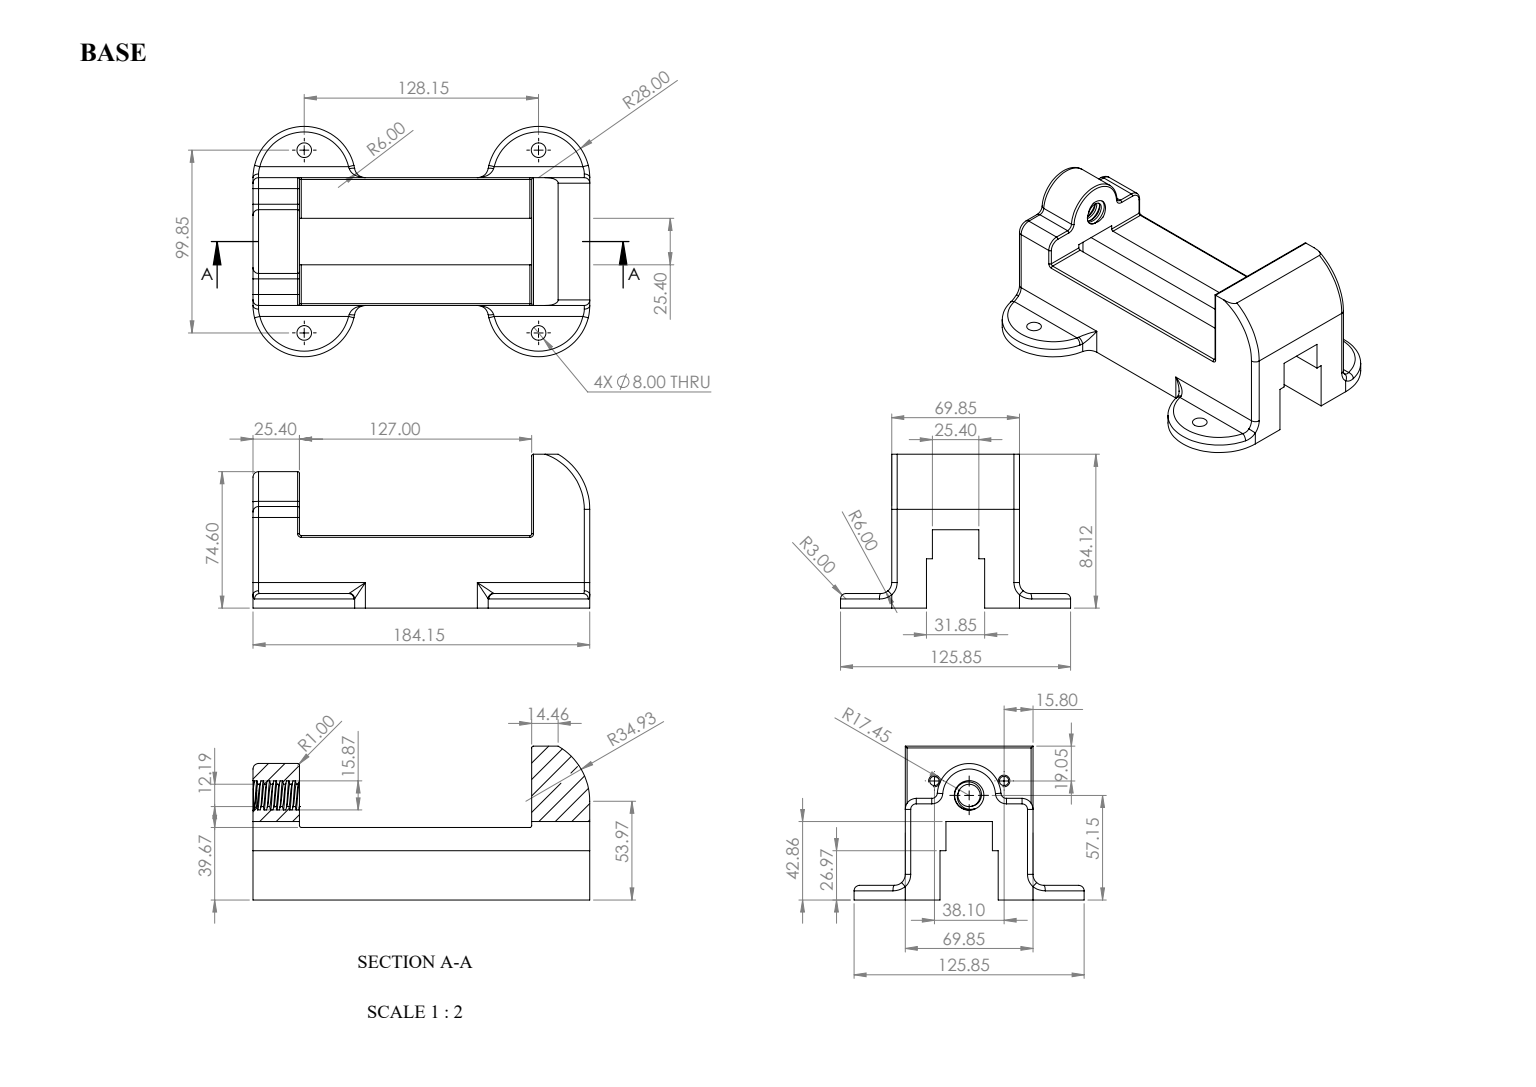
ISO-10303-21;
HEADER;
FILE_DESCRIPTION (('STEP AP214'),
    '1' );
FILE_NAME ('1.0 Base.step',
    '2026-10-06T08:51:13',
    ( '' ),
    ( '' ),
    'SwSTEP 2.0',
    'SolidWorks 2021',
    '' );
FILE_SCHEMA (( 'AUTOMOTIVE_DESIGN' ));
ENDSEC;

DATA;
#2=DIRECTION ( 'NONE',  ( 0.000000000000000000, 0.000000000000000000, -1.000000000000000000 ) ) ;
#4=CARTESIAN_POINT ( 'NONE',  ( 156.1499999999997783, -49.14999999999999147, -40.92499999999998295 ) ) ;
#20=DIRECTION ( 'NONE',  ( -1.000000000000000000, -0.000000000000000000, -0.000000000000000000 ) ) ;
#21=CYLINDRICAL_SURFACE ( 'NONE', #62371, 5.999999999999998224 ) ;
#28=AXIS2_PLACEMENT_3D ( 'NONE', #83260, #28167, #72429 ) ;
#56=ORIENTED_EDGE ( 'NONE', *, *, #91353, .F. ) ;
#80=CARTESIAN_POINT ( 'NONE',  ( 166.6274442290528555, 26.96999999999994202, -32.76433874914447131 ) ) ;
#88=CARTESIAN_POINT ( 'NONE',  ( 23.54623647476855552, -7.934999999999990727, 4.858786175617117713E-16 ) ) ;
#107=LINE ( 'NONE', #77033, #97406 ) ;
#112=MECHANICAL_DESIGN_GEOMETRIC_PRESENTATION_REPRESENTATION('',(#37206),#67225);
#141=( NAMED_UNIT ( * ) SI_UNIT ( $, .STERADIAN. ) SOLID_ANGLE_UNIT ( ) );
#143=ORIENTED_EDGE ( 'NONE', *, *, #47317, .T. ) ;
#169=AXIS2_PLACEMENT_3D ( 'NONE', #60485, #124990, #72084 ) ;
#182=CARTESIAN_POINT ( 'NONE',  ( 0.1600000000000011136, 3.289720434613005118, -7.220939306079887210 ) ) ;
#201=ORIENTED_EDGE ( 'NONE', *, *, #80508, .F. ) ;
#210=AXIS2_PLACEMENT_3D ( 'NONE', #18854, #51517, #105848 ) ;
#244=B_SPLINE_CURVE_WITH_KNOTS ( 'NONE', 3,
 ( #116047, #19597, #116769, #42097, #141380, #17451, #127667, #74728, #105869, #52917, #50814, #86307 ),
 .UNSPECIFIED., .F., .F.,
 ( 4, 2, 2, 2, 2, 4 ),
 ( 9.813815432834144085E-18, 0.001837441947543535809, 0.003674883895087062077, 0.004593604868858823694, 0.005512325842630587044, 0.007349767790174136298 ),
 .UNSPECIFIED. ) ;
#248=ADVANCED_FACE ( 'NONE', ( #84846 ), #37182, .F. ) ;
#274=CARTESIAN_POINT ( 'NONE',  ( -0.2245968585647807325, -2.126176841940958351, -7.934999999999989839 ) ) ;
#307=SURFACE_SIDE_STYLE ('',( #35140 ) ) ;
#315=ORIENTED_EDGE ( 'NONE', *, *, #1789, .F. ) ;
#365=MECHANICAL_DESIGN_GEOMETRIC_PRESENTATION_REPRESENTATION('',(#53591),#69867);
#369=EDGE_CURVE ( 'NONE', #137573, #138987, #81190, .T. ) ;
#372=CARTESIAN_POINT ( 'NONE',  ( 24.39999999999999858, -5.520864266206504263E-14, 0.000000000000000000 ) ) ;
#377=SURFACE_STYLE_USAGE ( .BOTH. , #24296 ) ;
#387=( NAMED_UNIT ( * ) SI_UNIT ( $, .STERADIAN. ) SOLID_ANGLE_UNIT ( ) );
#408=AXIS2_PLACEMENT_3D ( 'NONE', #118351, #30665, #74896 ) ;
#412=LINE ( 'NONE', #119338, #62884 ) ;
#443=MECHANICAL_DESIGN_GEOMETRIC_PRESENTATION_REPRESENTATION('',(#97739),#18987);
#457=CARTESIAN_POINT ( 'NONE',  ( 1.504139616203772789, -3.047499999999994547, 5.278424836066145431 ) ) ;
#484=CARTESIAN_POINT ( 'NONE',  ( 10.33290314143522082, -3.967499999999994476, 6.871911579029513106 ) ) ;
#486=DIRECTION ( 'NONE',  ( 0.000000000000000000, 0.000000000000000000, -1.000000000000000000 ) ) ;
#518=ORIENTED_EDGE ( 'NONE', *, *, #141850, .T. ) ;
#524=( NAMED_UNIT ( * ) SI_UNIT ( $, .STERADIAN. ) SOLID_ANGLE_UNIT ( ) );
#528=CARTESIAN_POINT ( 'NONE',  ( 18.22916666666666785, -6.094999999999989093, 1.633150327867691765 ) ) ;
#532=VECTOR ( 'NONE', #82631, 1000.000000000000000 ) ;
#538=COLOUR_RGB ( '', 0.09019608, 0.27058824, 0.51372549) ;
#587=ORIENTED_EDGE ( 'NONE', *, *, #53900, .F. ) ;
#590=CARTESIAN_POINT ( 'NONE',  ( 18.00456980810188767, 6.871911579029510442, -3.967499999999998916 ) ) ;
#592=CARTESIAN_POINT ( 'NONE',  ( 166.4267503027637929, 26.96999999999993847, 33.05223327726561422 ) ) ;
#634=CARTESIAN_POINT ( 'NONE',  ( 24.39999999999999858, -16.48000000000005016, 33.92499999999998295 ) ) ;
#651=B_SPLINE_CURVE_WITH_KNOTS ( 'NONE', 3,
 ( #139201, #42017, #96340, #72543, #117387, #140584, #118840, #17386, #41274, #9323, #39892, #85482, #18060, #129710, #30417, #19530, #31144, #107932, #8601, #52849, #97044, #141306, #86234, #119521, #53605, #103316, #91068, #114212, #48245, #79507, #101192, #14894, #25050, #57018 ),
 .UNSPECIFIED., .F., .F.,
 ( 4, 2, 2, 2, 2, 2, 2, 2, 2, 2, 2, 2, 2, 2, 2, 2, 4 ),
 ( 0.000000000000000000, 0.002428652292010244872, 0.003642978438015367741, 0.004857304584020490611, 0.006071630730025613480, 0.007285956876030735482, 0.008500283022035860087, 0.009714609168040984691, 0.01032177224104354613, 0.01092893531404610583, 0.01214326146005123043, 0.01335758760605635503, 0.01457191375206147964, 0.01578623989806660424, 0.01700056604407173058, 0.01821489219007685345, 0.01942921833608197632 ),
 .UNSPECIFIED. ) ;
#666=CARTESIAN_POINT ( 'NONE',  ( 16.10873647476855552, -5.808823158059033709, 5.808823158059035485 ) ) ;
#672=VERTEX_POINT ( 'NONE', #81409 ) ;
#679=FILL_AREA_STYLE ('',( #44971 ) ) ;
#692=FILL_AREA_STYLE_COLOUR ( '', #111503 ) ;
#702=CARTESIAN_POINT ( 'NONE',  ( 20.68706980810189222, -2.126176841940956130, 7.934999999999991616 ) ) ;
#720=CARTESIAN_POINT ( 'NONE',  ( 22.75000000000000355, -7.464222240803106570E-16, -6.094999999999989981 ) ) ;
#725=DIRECTION ( 'NONE',  ( -1.000000000000000000, 0.000000000000000000, -0.000000000000000000 ) ) ;
#768=EDGE_CURVE ( 'NONE', #109345, #74861, #53227, .T. ) ;
#785=EDGE_CURVE ( 'NONE', #137573, #33799, #105265, .T. ) ;
#826=CARTESIAN_POINT ( 'NONE',  ( 28.21290314143522338, 3.967499999999992699, -6.871911579029513994 ) ) ;
#875=EDGE_LOOP ( 'NONE', ( #85490, #63150, #94760, #112992 ) ) ;
#892=CARTESIAN_POINT ( 'NONE',  ( 1.342642840338568844, 0.4167709042101988004, 6.752357159661401376 ) ) ;
#910=ORIENTED_EDGE ( 'NONE', *, *, #110228, .T. ) ;
#939=ADVANCED_FACE ( 'NONE', ( #54479 ), #21, .F. ) ;
#946=AXIS2_PLACEMENT_3D ( 'NONE', #78392, #9523, #76993 ) ;
#975=ADVANCED_FACE ( 'NONE', ( #25374 ), #2165, .F. ) ;
#998=CARTESIAN_POINT ( 'NONE',  ( 31.98330628287044064, 6.094999999999991758, 1.633150327867687102 ) ) ;
#1009=EDGE_CURVE ( 'NONE', #4395, #106598, #120848, .T. ) ;
#1028=PRESENTATION_STYLE_ASSIGNMENT (( #46764 ) ) ;
#1035=DIRECTION ( 'NONE',  ( -0.000000000000000000, 1.000000000000000000, -0.000000000000000000 ) ) ;
#1043=( NAMED_UNIT ( * ) SI_UNIT ( $, .STERADIAN. ) SOLID_ANGLE_UNIT ( ) );
#1061=UNCERTAINTY_MEASURE_WITH_UNIT (LENGTH_MEASURE( 1.000000000000000082E-05 ), #107553, 'distance_accuracy_value', 'NONE');
#1082=AXIS2_PLACEMENT_3D ( 'NONE', #48681, #26916, #84193 ) ;
#1090=DIRECTION ( 'NONE',  ( -1.000000000000000000, -0.000000000000000000, 0.000000000000000000 ) ) ;
#1101=CIRCLE ( 'NONE', #47540, 2.552699999999990865 ) ;
#1141=CARTESIAN_POINT ( 'NONE',  ( 4.420806282870438864, 3.047499999999997655, 5.278424836066143655 ) ) ;
#1154=ORIENTED_EDGE ( 'NONE', *, *, #33420, .T. ) ;
#1163=CARTESIAN_POINT ( 'NONE',  ( 6.462472949537106715, -7.464222240803106570E-16, -6.094999999999989981 ) ) ;
#1194=CARTESIAN_POINT ( 'NONE',  ( 17.04123647476855652, 0.000000000000000000, 7.934999999999990727 ) ) ;
#1203=CARTESIAN_POINT ( 'NONE',  ( 156.1500000000000057, -49.14999999999999147, 49.92499999999997584 ) ) ;
#1221=( NAMED_UNIT ( * ) SI_UNIT ( $, .STERADIAN. ) SOLID_ANGLE_UNIT ( ) );
#1229=ORIENTED_EDGE ( 'NONE', *, *, #123542, .F. ) ;
#1240=CARTESIAN_POINT ( 'NONE',  ( 15.60416666666666430, -1.633150327867691987, -6.094999999999989093 ) ) ;
#1265=CARTESIAN_POINT ( 'NONE',  ( 156.1499999999997783, -52.14999999999999147, 34.92500000000004690 ) ) ;
#1268=CARTESIAN_POINT ( 'NONE',  ( 184.1499999999998067, -3.180000000000061444, 31.92499999999998295 ) ) ;
#1297=CARTESIAN_POINT ( 'NONE',  ( 24.85873647476855552, 5.808823158059031044, -5.808823158059037262 ) ) ;
#1322=CARTESIAN_POINT ( 'NONE',  ( 25.39999999999999858, 0.000000000000000000, 0.000000000000000000 ) ) ;
#1327=SURFACE_STYLE_FILL_AREA ( #56502 ) ;
#1332=ORIENTED_EDGE ( 'NONE', *, *, #26827, .F. ) ;
#1354=CARTESIAN_POINT ( 'NONE',  ( 13.75413961620377457, 3.047499999999993214, -5.278424836066146320 ) ) ;
#1363=CARTESIAN_POINT ( 'NONE',  ( 22.08790314143522338, 6.871911579029515771, 3.967499999999989146 ) ) ;
#1392=SURFACE_SIDE_STYLE ('',( #100744 ) ) ;
#1393=UNCERTAINTY_MEASURE_WITH_UNIT (LENGTH_MEASURE( 1.000000000000000082E-05 ), #82010, 'distance_accuracy_value', 'NONE');
#1407=CARTESIAN_POINT ( 'NONE',  ( 21.85373647476855297, -5.808823158059035485, -5.808823158059033709 ) ) ;
#1408=CARTESIAN_POINT ( 'NONE',  ( 0.7079031414352193741, -6.871911579029513106, -3.967499999999993587 ) ) ;
#1447=TOROIDAL_SURFACE ( 'NONE', #52377, 16.45000000000002061, 1.000000000000000000 ) ;
#1454=EDGE_CURVE ( 'NONE', #23170, #56532, #105103, .T. ) ;
#1462=DIRECTION ( 'NONE',  ( -0.000000000000000000, 1.000000000000000000, 0.000000000000000000 ) ) ;
#1477=STYLED_ITEM ( 'NONE', ( #106319 ), #33707 ) ;
#1480=CARTESIAN_POINT ( 'NONE',  ( 24.39999999999999858, -7.600000000000061817, 28.92499999999998650 ) ) ;
#1482=COLOUR_RGB ( '', 0.66274510, 0.83137255, 0.94901961) ;
#1484=ORIENTED_EDGE ( 'NONE', *, *, #38988, .F. ) ;
#1494=VECTOR ( 'NONE', #70882, 1000.000000000000000 ) ;
#1525=CARTESIAN_POINT ( 'NONE',  ( 23.98373647476855197, -5.808823158059035485, -5.808823158059033709 ) ) ;
#1556=CIRCLE ( 'NONE', #98752, 3.000000000000003109 ) ;
#1568=DIRECTION ( 'NONE',  ( 0.000000000000000000, 5.075120898959323014E-15, 1.000000000000000000 ) ) ;
#1597=DIRECTION ( 'NONE',  ( 0.000000000000000000, -0.000000000000000000, -1.000000000000000000 ) ) ;
#1618=CARTESIAN_POINT ( 'NONE',  ( 152.4000000000000057, 26.55578643762684266, -34.51078643762689069 ) ) ;
#1627=( LENGTH_UNIT ( ) NAMED_UNIT ( * ) SI_UNIT ( .MILLI., .METRE. ) );
#1645=DIRECTION ( 'NONE',  ( -0.000000000000000000, -1.000000000000000000, 0.000000000000000000 ) ) ;
#1687=EDGE_CURVE ( 'NONE', #77069, #96033, #119634, .T. ) ;
#1689=VECTOR ( 'NONE', #126123, 1000.000000000000227 ) ;
#1690=CARTESIAN_POINT ( 'NONE',  ( -1.245430191898114103, -6.871911579029512218, 3.967499999999996252 ) ) ;
#1722=SURFACE_SIDE_STYLE ('',( #57606 ) ) ;
#1732=CARTESIAN_POINT ( 'NONE',  ( 0.000000000000000000, -43.14999999999996305, -31.92499999999998295 ) ) ;
#1733=( LENGTH_UNIT ( ) NAMED_UNIT ( * ) SI_UNIT ( .MILLI., .METRE. ) );
#1789=EDGE_CURVE ( 'NONE', #98679, #119012, #89647, .T. ) ;
#1819=( BOUNDED_SURFACE ( )  B_SPLINE_SURFACE ( 3, 2, ( 
 ( #75238, #141164, #5640 ),
 ( #30275, #8477, #72404 ),
 ( #73785, #50607, #62935 ),
 ( #52728, #28860, #94792 ),
 ( #40465, #19397, #96921 ),
 ( #63650, #52038, #84666 ),
 ( #117253, #128868, #116573 ),
 ( #7786, #119399, #17258 ),
 ( #20093, #61519, #96217 ),
 ( #7051, #139052, #62213 ),
 ( #106368, #104975, #29544 ),
 ( #140459, #41150, #118705 ) ),
 .UNSPECIFIED., .F., .F., .F. ) 
 B_SPLINE_SURFACE_WITH_KNOTS ( ( 4, 2, 2, 2, 2, 4 ),
 ( 3, 3 ),
 ( 0.000000000000000000, 0.001647923167088021293, 0.002471884750632031939, 0.003295846334176042586, 0.004943769501264063879, 0.006591692668352085172 ),
 ( 0.000000000000000000, 1.000000000000000000 ),
 .UNSPECIFIED. ) 
 GEOMETRIC_REPRESENTATION_ITEM ( )  RATIONAL_B_SPLINE_SURFACE ( (
 ( 1.000000000000000000, 0.7071067811865475727, 1.000000000000000000),
 ( 1.000000000000000000, 0.7122033721489959834, 1.000000000000000000),
 ( 1.000000000000000000, 0.7158366153114920083, 1.000000000000000000),
 ( 1.000000000000000000, 0.7192720032935927543, 1.000000000000000000),
 ( 1.000000000000000000, 0.7200809050419634261, 1.000000000000000000),
 ( 1.000000000000000000, 0.7210491446662590231, 1.000000000000000000),
 ( 1.000000000000000000, 0.7212054070301950892, 1.000000000000000000),
 ( 1.000000000000000000, 0.7207522793911053105, 1.000000000000000000),
 ( 1.000000000000000000, 0.7192424821648278899, 1.000000000000000000),
 ( 1.000000000000000000, 0.7143802006615703748, 1.000000000000000000),
 ( 1.000000000000000000, 0.7109884861396060796, 1.000000000000000000),
 ( 1.000000000000000000, 0.7071067811865475727, 1.000000000000000000) ) ) 
 REPRESENTATION_ITEM ( '' )  SURFACE ( )  );
#1824=CARTESIAN_POINT ( 'NONE',  ( 3.108306282870440640, 1.633150327867692431, -6.094999999999989093 ) ) ;
#1849=CARTESIAN_POINT ( 'NONE',  ( 3.545806282870439308, 5.278424836066143655, -3.047499999999997655 ) ) ;
#1857=CARTESIAN_POINT ( 'NONE',  ( 156.1500000000000057, -49.14999999999999147, -49.92499999999968452 ) ) ;
#1881=CARTESIAN_POINT ( 'NONE',  ( 23.74956980810188867, 3.967499999999998916, 6.871911579029510442 ) ) ;
#1889=FILL_AREA_STYLE ('',( #136727 ) ) ;
#1893=SURFACE_SIDE_STYLE ('',( #93240 ) ) ;
#1898=DIRECTION ( 'NONE',  ( 0.000000000000000000, 0.000000000000000000, 1.000000000000000000 ) ) ;
#1909=CIRCLE ( 'NONE', #85349, 1.000000000000000888 ) ;
#1913=SURFACE_STYLE_USAGE ( .BOTH. , #78832 ) ;
#1930=CARTESIAN_POINT ( 'NONE',  ( 9.625000000000001776, 6.094999999999989981, -1.119633336120465690E-15 ) ) ;
#1931=CARTESIAN_POINT ( 'NONE',  ( 23.02040314143522082, 7.934999999999988951, -2.126176841940961904 ) ) ;
#1941=CYLINDRICAL_SURFACE ( 'NONE', #89996, 6.094999999999989093 ) ;
#1943=CARTESIAN_POINT ( 'NONE',  ( 126.2665610010987649, -48.52444309369079178, -36.09967824800681768 ) ) ;
#1986=CARTESIAN_POINT ( 'NONE',  ( 25.34729149122530245, 7.934999999999992504, 0.7443565279215664798 ) ) ;
#1988=MECHANICAL_DESIGN_GEOMETRIC_PRESENTATION_REPRESENTATION('',(#117493),#76141);
#1990=CARTESIAN_POINT ( 'NONE',  ( 122.6835989386367345, -49.14999999999999147, 40.92499999999998295 ) ) ;
#1992=CARTESIAN_POINT ( 'NONE',  ( 25.39999999999999858, -7.600000000000055600, -34.92499999999998295 ) ) ;
#2000=MECHANICAL_DESIGN_GEOMETRIC_PRESENTATION_REPRESENTATION('',(#32175),#101598);
#2002=EDGE_LOOP ( 'NONE', ( #24135, #30818, #116626, #50545 ) ) ;
#2035=EDGE_CURVE ( 'NONE', #89687, #67143, #85183, .T. ) ;
#2058=DIRECTION ( 'NONE',  ( 0.000000000000000000, 0.000000000000000000, 1.000000000000000000 ) ) ;
#2062=B_SPLINE_CURVE_WITH_KNOTS ( 'NONE', 3,
 ( #100924, #13179, #111820, #90042, #23356, #101638, #45166, #79231, #89342, #135028, #47329, #123436, #2291, #46612, #58919, #35722, #91500, #12482, #113220, #122669, #79942, #135712, #56764, #113949, #124113, #69039, #24790, #36396 ),
 .UNSPECIFIED., .F., .F.,
 ( 4, 2, 2, 2, 2, 2, 2, 2, 2, 2, 2, 2, 2, 4 ),
 ( 0.002830889048686786869, 0.003748869865235868355, 0.004666850681784949842, 0.005584831498334031329, 0.006502812314883112815, 0.008338773947981275789, 0.009256754764530356408, 0.01017473558107943703, 0.01109271639762851765, 0.01201069721417759653, 0.01292867803072667542, 0.01384665884727575430, 0.01568262048037391554, 0.01751858211347207331 ),
 .UNSPECIFIED. ) ;
#2063=CARTESIAN_POINT ( 'NONE',  ( 16.40040314143521982, -7.934999999999989839, 2.126176841940957907 ) ) ;
#2070=ORIENTED_EDGE ( 'NONE', *, *, #46056, .T. ) ;
#2076=SURFACE_STYLE_USAGE ( .BOTH. , #123925 ) ;
#2092=SURFACE_SIDE_STYLE ('',( #68167 ) ) ;
#2104=CARTESIAN_POINT ( 'NONE',  ( 23.16623647476855652, 7.934999999999990727, -1.457635852685135314E-15 ) ) ;
#2106=VECTOR ( 'NONE', #67234, 1000.000000000000000 ) ;
#2153=EDGE_CURVE ( 'NONE', #103874, #56532, #135388, .T. ) ;
#2158=CARTESIAN_POINT ( 'NONE',  ( 8.649972949537106715, -4.461849672132299105, 4.461849672132299993 ) ) ;
#2165=PLANE ( 'NONE',  #97069 ) ;
#2168=ORIENTED_EDGE ( 'NONE', *, *, #2569, .T. ) ;
#2219=ORIENTED_EDGE ( 'NONE', *, *, #107714, .F. ) ;
#2238=CARTESIAN_POINT ( 'NONE',  ( 24.27540314143521982, -2.126176841940958351, -7.934999999999989839 ) ) ;
#2245=ORIENTED_EDGE ( 'NONE', *, *, #101650, .F. ) ;
#2246=CARTESIAN_POINT ( 'NONE',  ( 25.39999999999999858, 1.194621026894847171, -17.40906030209848510 ) ) ;
#2278=LINE ( 'NONE', #124814, #21647 ) ;
#2291=CARTESIAN_POINT ( 'NONE',  ( 1.000065336733412913, -5.551087553957981591, -4.428894815882122415 ) ) ;
#2414=AXIS2_PLACEMENT_3D ( 'NONE', #81917, #4980, #106434 ) ;
#2417=CARTESIAN_POINT ( 'NONE',  ( 3.858736474768553304, 5.808823158059031044, -5.808823158059038150 ) ) ;
#2444=CARTESIAN_POINT ( 'NONE',  ( 21.19163961620376924, 6.094999999999988205, -1.633150327867694651 ) ) ;
#2449=EDGE_CURVE ( 'NONE', #21837, #31597, #130626, .T. ) ;
#2455=CARTESIAN_POINT ( 'NONE',  ( 0.2704031414352194296, -7.934999999999989839, 2.126176841940957907 ) ) ;
#2461=UNCERTAINTY_MEASURE_WITH_UNIT (LENGTH_MEASURE( 1.000000000000000082E-05 ), #59794, 'distance_accuracy_value', 'NONE');
#2466=CARTESIAN_POINT ( 'NONE',  ( 156.1500000000000057, -49.14999999999999147, 45.92499999999998295 ) ) ;
#2473=CARTESIAN_POINT ( 'NONE',  ( 26.40000000000000568, -17.48000000000005016, 12.69999999999954454 ) ) ;
#2482=UNCERTAINTY_MEASURE_WITH_UNIT (LENGTH_MEASURE( 1.000000000000000082E-05 ), #112838, 'distance_accuracy_value', 'NONE');
#2484=DIRECTION ( 'NONE',  ( -1.000000000000000000, -0.000000000000000000, 0.000000000000000000 ) ) ;
#2547=CIRCLE ( 'NONE', #139195, 25.00000000000002842 ) ;
#2558=( GEOMETRIC_REPRESENTATION_CONTEXT ( 3 ) GLOBAL_UNCERTAINTY_ASSIGNED_CONTEXT ( ( #139093 ) ) GLOBAL_UNIT_ASSIGNED_CONTEXT ( ( #79225, #54587, #141 ) ) REPRESENTATION_CONTEXT ( 'NONE', 'WORKASPACE' ) );
#2569=EDGE_CURVE ( 'NONE', #119600, #105140, #15754, .T. ) ;
#2572=ORIENTED_EDGE ( 'NONE', *, *, #62327, .T. ) ;
#2594=CARTESIAN_POINT ( 'NONE',  ( 8.212472949537106715, 0.000000000000000000, 6.094999999999989981 ) ) ;
#2606=SURFACE_STYLE_FILL_AREA ( #78778 ) ;
#2621=( LENGTH_UNIT ( ) NAMED_UNIT ( * ) SI_UNIT ( .MILLI., .METRE. ) );
#2630=CARTESIAN_POINT ( 'NONE',  ( 19.66623647476855297, 7.934999999999990727, -1.457635852685135314E-15 ) ) ;
#2660=ORIENTED_EDGE ( 'NONE', *, *, #41190, .F. ) ;
#2675=CARTESIAN_POINT ( 'NONE',  ( 17.50000000000000000, 0.000000000000000000, 6.094999999999989981 ) ) ;
#2677=CARTESIAN_POINT ( 'NONE',  ( 24.18706980810188867, -2.126176841940956130, 7.934999999999990727 ) ) ;
#2691=CARTESIAN_POINT ( 'NONE',  ( 124.0768256643040388, -45.23984008851422089, -35.04755940937664604 ) ) ;
#2693=DIRECTION ( 'NONE',  ( 0.000000000000000000, 0.000000000000000000, 1.000000000000000000 ) ) ;
#2739=FACE_OUTER_BOUND ( 'NONE', #96191, .T. ) ;
#2740=CARTESIAN_POINT ( 'NONE',  ( 25.15040314143521627, 7.934999999999988951, -2.126176841940961904 ) ) ;
#2753=EDGE_CURVE ( 'NONE', #89590, #131877, #7216, .T. ) ;
#2777=VERTEX_POINT ( 'NONE', #129650 ) ;
#2786=STYLED_ITEM ( 'NONE', ( #120887 ), #31273 ) ;
#2799=CARTESIAN_POINT ( 'NONE',  ( 14.33747294953710494, 6.094999999999989981, -1.119633336120465690E-15 ) ) ;
#2808=CARTESIAN_POINT ( 'NONE',  ( 30.69206980810189123, -7.934999999999991616, -2.126176841940955242 ) ) ;
#2831=STYLED_ITEM ( 'NONE', ( #89354 ), #66228 ) ;
#2835=CARTESIAN_POINT ( 'NONE',  ( 60.76962477605442814, -44.19516442797058886, -34.92499999999998295 ) ) ;
#2842=UNCERTAINTY_MEASURE_WITH_UNIT (LENGTH_MEASURE( 1.000000000000000082E-05 ), #105526, 'distance_accuracy_value', 'NONE');
#2852=CARTESIAN_POINT ( 'NONE',  ( 23.31206980810188512, 7.934999999999993392, 2.126176841940951689 ) ) ;
#2862=B_SPLINE_CURVE_WITH_KNOTS ( 'NONE', 3,
 ( #57172, #101347, #46299, #18589, #127377, #96156, #83174, #116512, #70891, #16449, #94730, #40400, #51980, #60754 ),
 .UNSPECIFIED., .F., .F.,
 ( 4, 2, 2, 2, 2, 2, 4 ),
 ( 0.000000000000000000, 0.001506850370412668103, 0.002260275555619002154, 0.003013700740825336205, 0.003767125926031670256, 0.004520551111238004308, 0.006027401481650672410 ),
 .UNSPECIFIED. ) ;
#2879=CARTESIAN_POINT ( 'NONE',  ( 26.40000000000000568, -16.48000000000005016, 34.92499999999998295 ) ) ;
#2909=CARTESIAN_POINT ( 'NONE',  ( 1.233736474768552860, 5.808823158059035485, 5.808823158059032821 ) ) ;
#2933=ADVANCED_FACE ( 'NONE', ( #92376 ), #37674, .T. ) ;
#2978=CARTESIAN_POINT ( 'NONE',  ( 29.52540314143522338, 2.126176841940962348, 7.934999999999989839 ) ) ;
#2979=CARTESIAN_POINT ( 'NONE',  ( 0.6504031414352192675, 7.934999999999989839, -2.126176841940961904 ) ) ;
#3010=EDGE_CURVE ( 'NONE', #9331, #58595, #93214, .T. ) ;
#3016=SURFACE_STYLE_USAGE ( .BOTH. , #22088 ) ;
#3105=FILL_AREA_STYLE ('',( #68415 ) ) ;
#3140=VERTEX_POINT ( 'NONE', #21270 ) ;
#3149=CARTESIAN_POINT ( 'NONE',  ( -1.099596858564781066, -7.934999999999989839, 2.126176841940957907 ) ) ;
#3172=CARTESIAN_POINT ( 'NONE',  ( 20.60830628287044419, 1.633150327867706864, -6.094999999999981100 ) ) ;
#3181=AXIS2_PLACEMENT_3D ( 'NONE', #78101, #67216, #1898 ) ;
#3185=DIRECTION ( 'NONE',  ( -0.000000000000000000, 0.000000000000000000, 1.000000000000000000 ) ) ;
#3192=FILL_AREA_STYLE ('',( #26399 ) ) ;
#3206=CARTESIAN_POINT ( 'NONE',  ( 24.39999999999999858, -16.48000000000005016, 34.92499999999998295 ) ) ;
#3278=( LENGTH_UNIT ( ) NAMED_UNIT ( * ) SI_UNIT ( .MILLI., .METRE. ) );
#3307=CARTESIAN_POINT ( 'NONE',  ( 2.087472949537105826, -6.094999999999989981, 3.732111120401553285E-16 ) ) ;
#3324=ORIENTED_EDGE ( 'NONE', *, *, #105654, .T. ) ;
#3328=( NAMED_UNIT ( * ) SI_UNIT ( $, .STERADIAN. ) SOLID_ANGLE_UNIT ( ) );
#3338=CARTESIAN_POINT ( 'NONE',  ( 26.66623647476855652, 7.934999999999990727, -1.457635852685135314E-15 ) ) ;
#3354=MECHANICAL_DESIGN_GEOMETRIC_PRESENTATION_REPRESENTATION('',(#65920),#119170);
#3369=SURFACE_STYLE_FILL_AREA ( #102724 ) ;
#3383=CARTESIAN_POINT ( 'NONE',  ( 19.25000000000000355, -7.464222240803106570E-16, -6.094999999999989981 ) ) ;
#3440=CARTESIAN_POINT ( 'NONE',  ( 55.56056557994604361, -49.14999999999999147, -39.86617647058817937 ) ) ;
#3447=( GEOMETRIC_REPRESENTATION_CONTEXT ( 3 ) GLOBAL_UNCERTAINTY_ASSIGNED_CONTEXT ( ( #46051 ) ) GLOBAL_UNIT_ASSIGNED_CONTEXT ( ( #123452, #36410, #103772 ) ) REPRESENTATION_CONTEXT ( 'NONE', 'WORKASPACE' ) );
#3501=CARTESIAN_POINT ( 'NONE',  ( 25.44206980810188412, 7.934999999999993392, 2.126176841940951689 ) ) ;
#3503=LINE ( 'NONE', #47794, #110755 ) ;
#3529=( NAMED_UNIT ( * ) PLANE_ANGLE_UNIT ( ) SI_UNIT ( $, .RADIAN. ) );
#3537=( BOUNDED_CURVE ( )  B_SPLINE_CURVE ( 2, ( #138028, #61913, #72821, #114807, #71352, #93800, #25682, #126417, #59081, #4581, #92352, #27829, #94498 ),
 .UNSPECIFIED., .F., .T. ) 
 B_SPLINE_CURVE_WITH_KNOTS ( ( 3, 2, 2, 2, 2, 2, 3 ),
 ( 0.3000000000000000444, 0.3083333333333334036, 0.3166666666666667074, 0.3250000000000000666, 0.3333333333333333703, 0.3416666666666667296, 0.3500000000000000333 ),
 .UNSPECIFIED. ) 
 CURVE ( )  GEOMETRIC_REPRESENTATION_ITEM ( )  RATIONAL_B_SPLINE_CURVE ( ( 0.9999999999999997780, 0.9659258262890685343, 1.000000000000000000, 0.9659258262890683122, 1.000000000000000000, 0.9659258262890683122, 1.000000000000000000, 0.9659258262890683122, 1.000000000000000000, 0.9659258262890683122, 1.000000000000000000, 0.9659258262890680902, 1.000000000000000222 ) ) 
 REPRESENTATION_ITEM ( '' )  );
#3545=CARTESIAN_POINT ( 'NONE',  ( 30.45790314143522437, 6.871911579029515771, 3.967499999999989146 ) ) ;
#3558=CARTESIAN_POINT ( 'NONE',  ( 25.39999999999999858, -57.15000000000009095, 34.92499999999998295 ) ) ;
#3574=CARTESIAN_POINT ( 'NONE',  ( 25.39999999999999858, -43.14999999999999147, 34.92499999999998295 ) ) ;
#3600=CARTESIAN_POINT ( 'NONE',  ( 1.962903141435219601, -3.967499999999994476, 6.871911579029513106 ) ) ;
#3601=EDGE_CURVE ( 'NONE', #112055, #60580, #89222, .T. ) ;
#3620=DIRECTION ( 'NONE',  ( 0.000000000000000000, 0.000000000000000000, -1.000000000000000000 ) ) ;
#3633=ORIENTED_EDGE ( 'NONE', *, *, #118658, .T. ) ;
#3660=CARTESIAN_POINT ( 'NONE',  ( 32.73373647476854842, 5.808823158059036373, 5.808823158059032821 ) ) ;
#3662=CARTESIAN_POINT ( 'NONE',  ( 0.9420698081018860082, 7.934999999999993392, 2.126176841940951689 ) ) ;
#3666=CIRCLE ( 'NONE', #29167, 5.999999999999998224 ) ;
#3677=CARTESIAN_POINT ( 'NONE',  ( 56.90810577924025893, -46.18886352141517904, -34.92499999999998295 ) ) ;
#3695=DIRECTION ( 'NONE',  ( 0.000000000000000000, -1.000000000000000000, 0.000000000000000000 ) ) ;
#3702=CARTESIAN_POINT ( 'NONE',  ( 184.1500000000000057, -30.18000000000009564, -15.92500000000064375 ) ) ;
#3707=ORIENTED_EDGE ( 'NONE', *, *, #112697, .F. ) ;
#3713=EDGE_LOOP ( 'NONE', ( #114435, #13870, #8632, #138126 ) ) ;
#3729=CARTESIAN_POINT ( 'NONE',  ( 0.7902862351827044662, 7.048400157404861588, 1.962111654240061398 ) ) ;
#3737=( LENGTH_UNIT ( ) NAMED_UNIT ( * ) SI_UNIT ( .MILLI., .METRE. ) );
#3746=DIRECTION ( 'NONE',  ( -1.000000000000000000, -0.000000000000000000, 0.000000000000000000 ) ) ;
#3788=SURFACE_STYLE_FILL_AREA ( #37178 ) ;
#3809=( GEOMETRIC_REPRESENTATION_CONTEXT ( 3 ) GLOBAL_UNCERTAINTY_ASSIGNED_CONTEXT ( ( #30502 ) ) GLOBAL_UNIT_ASSIGNED_CONTEXT ( ( #103757, #72641, #27642 ) ) REPRESENTATION_CONTEXT ( 'NONE', 'WORKASPACE' ) );
#3824=CARTESIAN_POINT ( 'NONE',  ( 5.608736474768551972, -5.808823158059033709, 5.808823158059035485 ) ) ;
#3832=CARTESIAN_POINT ( 'NONE',  ( 24.50000000000000000, 0.000000000000000000, 6.094999999999989981 ) ) ;
#3843=EDGE_CURVE ( 'NONE', #4395, #28418, #104084, .T. ) ;
#3863=CARTESIAN_POINT ( 'NONE',  ( 1.145403141435219485, -2.126176841940958351, -7.934999999999989839 ) ) ;
#3891=UNCERTAINTY_MEASURE_WITH_UNIT (LENGTH_MEASURE( 1.000000000000000082E-05 ), #7913, 'distance_accuracy_value', 'NONE');
#3906=COLOUR_RGB ( '', 0.40784314, 0.44705882, 0.49803922) ;
#3966=( NAMED_UNIT ( * ) SI_UNIT ( $, .STERADIAN. ) SOLID_ANGLE_UNIT ( ) );
#3982=CARTESIAN_POINT ( 'NONE',  ( 10.25413961620377457, 3.047499999999993214, -5.278424836066146320 ) ) ;
#4005=SURFACE_STYLE_USAGE ( .BOTH. , #25818 ) ;
#4011=ORIENTED_EDGE ( 'NONE', *, *, #127323, .T. ) ;
#4014=CARTESIAN_POINT ( 'NONE',  ( 18.35373647476854941, -5.808823158059035485, -5.808823158059033709 ) ) ;
#4047=( NAMED_UNIT ( * ) SI_UNIT ( $, .STERADIAN. ) SOLID_ANGLE_UNIT ( ) );
#4061=CARTESIAN_POINT ( 'NONE',  ( 20.12500000000000000, 6.094999999999989981, -1.119633336120465690E-15 ) ) ;
#4111=FILL_AREA_STYLE_COLOUR ( '', #91954 ) ;
#4147=ADVANCED_FACE ( 'NONE', ( #92736 ), #28926, .F. ) ;
#4156=SURFACE_STYLE_USAGE ( .BOTH. , #17921 ) ;
#4174=CARTESIAN_POINT ( 'NONE',  ( 23.98373647476855197, -5.808823158059035485, -5.808823158059033709 ) ) ;
#4197=FILL_AREA_STYLE_COLOUR ( '', #16370 ) ;
#4217=CARTESIAN_POINT ( 'NONE',  ( 24.39999999999999858, -2.599999999999900169, -1.445354724476153568E-14 ) ) ;
#4218=CARTESIAN_POINT ( 'NONE',  ( 30.31206980810188512, 7.934999999999993392, 2.126176841940951689 ) ) ;
#4220=CARTESIAN_POINT ( 'NONE',  ( 15.21247294953710671, 0.000000000000000000, 6.094999999999989981 ) ) ;
#4228=FILL_AREA_STYLE_COLOUR ( '', #87383 ) ;
#4232=MECHANICAL_DESIGN_GEOMETRIC_PRESENTATION_REPRESENTATION('',(#34422),#124659);
#4237=COLOUR_RGB ( '', 0.09019608, 0.27058824, 0.51372549) ;
#4257=CONICAL_SURFACE ( 'NONE', #36705, 2.552699999999928693, 1.029744258676634772 ) ;
#4267=FACE_OUTER_BOUND ( 'NONE', #27129, .T. ) ;
#4277=CARTESIAN_POINT ( 'NONE',  ( 3.275403141435219823, -2.126176841940958351, -7.934999999999988951 ) ) ;
#4278=( LENGTH_UNIT ( ) NAMED_UNIT ( * ) SI_UNIT ( .MILLI., .METRE. ) );
#4285=CIRCLE ( 'NONE', #64597, 2.552699999999990865 ) ;
#4299=( NAMED_UNIT ( * ) PLANE_ANGLE_UNIT ( ) SI_UNIT ( $, .RADIAN. ) );
#4324=COLOUR_RGB ( '', 0.66274510, 0.83137255, 0.94901961) ;
#4327=FILL_AREA_STYLE_COLOUR ( '', #10280 ) ;
#4344=CARTESIAN_POINT ( 'NONE',  ( -0.9537635252314473622, -7.934999999999990727, 4.858786175617117713E-16 ) ) ;
#4355=( NAMED_UNIT ( * ) SI_UNIT ( $, .STERADIAN. ) SOLID_ANGLE_UNIT ( ) );
#4357=LINE ( 'NONE', #1992, #28863 ) ;
#4360=SURFACE_SIDE_STYLE ('',( #15271 ) ) ;
#4386=CARTESIAN_POINT ( 'NONE',  ( 2.187499999999999556, 4.461849672132297329, -4.461849672132302658 ) ) ;
#4395=VERTEX_POINT ( 'NONE', #65617 ) ;
#4466=STYLED_ITEM ( 'NONE', ( #105922 ), #96794 ) ;
#4495=MECHANICAL_DESIGN_GEOMETRIC_PRESENTATION_REPRESENTATION('',(#18400),#32319);
#4503=B_SPLINE_CURVE_WITH_KNOTS ( 'NONE', 3,
 ( #32332, #76565, #120745, #21451 ),
 .UNSPECIFIED., .F., .F.,
 ( 4, 4 ),
 ( 0.000000000000000000, 0.001824211539880358363 ),
 .UNSPECIFIED. ) ;
#4516=CARTESIAN_POINT ( 'NONE',  ( 5.171236474768553748, 0.000000000000000000, 7.934999999999990727 ) ) ;
#4554=CARTESIAN_POINT ( 'NONE',  ( 3.187069808101886448, -2.126176841940956130, 7.934999999999991616 ) ) ;
#4571=( NAMED_UNIT ( * ) PLANE_ANGLE_UNIT ( ) SI_UNIT ( $, .RADIAN. ) );
#4581=CARTESIAN_POINT ( 'NONE',  ( 11.81250000000000178, -4.461849672132299993, -4.461849672132299105 ) ) ;
#4610=CARTESIAN_POINT ( 'NONE',  ( 25.39999999999999858, -2.599999999999908606, 1.319531433729349815E-14 ) ) ;
#4627=CYLINDRICAL_SURFACE ( 'NONE', #126308, 5.999999999999998224 ) ;
#4645=VECTOR ( 'NONE', #19677, 1000.000000000000000 ) ;
#4662=SHAPE_DEFINITION_REPRESENTATION ( #15602, #40289 ) ;
#4696=CARTESIAN_POINT ( 'NONE',  ( 13.17080628287043886, -3.047499999999997211, -5.278424836066143655 ) ) ;
#4718=( NAMED_UNIT ( * ) PLANE_ANGLE_UNIT ( ) SI_UNIT ( $, .RADIAN. ) );
#4727=CARTESIAN_POINT ( 'NONE',  ( 20.83290314143522082, -3.967499999999994476, 6.871911579029513106 ) ) ;
#4764=CARTESIAN_POINT ( 'NONE',  ( 156.1499999999997783, -52.14999999999999147, -34.92499999999975557 ) ) ;
#4779=CARTESIAN_POINT ( 'NONE',  ( 27.85416666666666785, 1.633150327867695095, 6.094999999999988205 ) ) ;
#4804=CARTESIAN_POINT ( 'NONE',  ( 1.534715839894093881, -2.368487323979017400, 6.120741323661095024 ) ) ;
#4807=ORIENTED_EDGE ( 'NONE', *, *, #20774, .T. ) ;
#4814=( NAMED_UNIT ( * ) PLANE_ANGLE_UNIT ( ) SI_UNIT ( $, .RADIAN. ) );
#4831=ORIENTED_EDGE ( 'NONE', *, *, #48583, .F. ) ;
#4849=SURFACE_STYLE_USAGE ( .BOTH. , #94045 ) ;
#4852=SURFACE_STYLE_USAGE ( .BOTH. , #70905 ) ;
#4872=ORIENTED_EDGE ( 'NONE', *, *, #107178, .F. ) ;
#4906=FILL_AREA_STYLE_COLOUR ( '', #83444 ) ;
#4910=CARTESIAN_POINT ( 'NONE',  ( 29.96290314143522338, -3.967499999999994476, 6.871911579029513106 ) ) ;
#4916=MECHANICAL_DESIGN_GEOMETRIC_PRESENTATION_REPRESENTATION('',(#51342),#48971);
#4954=CARTESIAN_POINT ( 'NONE',  ( 33.08290314143522437, 3.967499999999992699, -6.871911579029513994 ) ) ;
#4955=CARTESIAN_POINT ( 'NONE',  ( 6.249569808101886004, 3.967499999999998916, 6.871911579029510442 ) ) ;
#4963=ORIENTED_EDGE ( 'NONE', *, *, #113865, .T. ) ;
#4971=VECTOR ( 'NONE', #7647, 1000.000000000000000 ) ;
#4980=DIRECTION ( 'NONE',  ( 0.2400000000000085398, 0.000000000000000000, -0.9707728879609256456 ) ) ;
#4990=ORIENTED_EDGE ( 'NONE', *, *, #122325, .F. ) ;
#5009=FILL_AREA_STYLE ('',( #59471 ) ) ;
#5019=CARTESIAN_POINT ( 'NONE',  ( 8.962903141435219823, -3.967499999999994476, 6.871911579029513106 ) ) ;
#5021=CARTESIAN_POINT ( 'NONE',  ( 21.29166666666666785, -3.047499999999994547, 5.278424836066145431 ) ) ;
#5030=EDGE_CURVE ( 'NONE', #53957, #2777, #59742, .T. ) ;
#5048=CARTESIAN_POINT ( 'NONE',  ( 131.5423521607622490, -49.05583548141700589, 39.86617647058822911 ) ) ;
#5063=ORIENTED_EDGE ( 'NONE', *, *, #50610, .F. ) ;
#5080=DIRECTION ( 'NONE',  ( 0.000000000000000000, -0.000000000000000000, 1.000000000000000000 ) ) ;
#5091=CARTESIAN_POINT ( 'NONE',  ( 3.421236474768552860, -9.717572351234235426E-16, -7.934999999999990727 ) ) ;
#5095=( NAMED_UNIT ( * ) SI_UNIT ( $, .STERADIAN. ) SOLID_ANGLE_UNIT ( ) );
#5102=FILL_AREA_STYLE_COLOUR ( '', #42754 ) ;
#5104=CARTESIAN_POINT ( 'NONE',  ( 183.9400257540259531, -51.66308182546809746, -38.35990878063539355 ) ) ;
#5117=ADVANCED_FACE ( 'NONE', ( #15237 ), #37016, .F. ) ;
#5124=STYLED_ITEM ( 'NONE', ( #127792 ), #25975 ) ;
#5136=CYLINDRICAL_SURFACE ( 'NONE', #12259, 6.094999999999989093 ) ;
#5141=CARTESIAN_POINT ( 'NONE',  ( 24.39999999999999858, -2.600000000000013856, 20.40202195861968448 ) ) ;
#5143=EDGE_CURVE ( 'NONE', #60071, #48370, #140733, .T. ) ;
#5165=AXIS2_PLACEMENT_3D ( 'NONE', #117507, #137881, #71926 ) ;
#5175=ORIENTED_EDGE ( 'NONE', *, *, #110228, .F. ) ;
#5238=DIRECTION ( 'NONE',  ( 1.000000000000000000, 0.000000000000000000, 0.000000000000000000 ) ) ;
#5240=VERTEX_POINT ( 'NONE', #42762 ) ;
#5275=CARTESIAN_POINT ( 'NONE',  ( 5.900403141435219823, -7.934999999999989839, 2.126176841940957907 ) ) ;
#5277=VERTEX_POINT ( 'NONE', #44929 ) ;
#5289=DIRECTION ( 'NONE',  ( 0.000000000000000000, -1.000000000000000000, 0.000000000000000000 ) ) ;
#5303=CARTESIAN_POINT ( 'NONE',  ( 22.06663961620377279, 1.633150327867675555, 6.094999999999998863 ) ) ;
#5306=FILL_AREA_STYLE_COLOUR ( '', #110919 ) ;
#5315=CARTESIAN_POINT ( 'NONE',  ( 2.749569808101886004, 3.967499999999998916, 6.871911579029510442 ) ) ;
#5340=SURFACE_STYLE_FILL_AREA ( #69961 ) ;
#5341=VERTEX_POINT ( 'NONE', #22374 ) ;
#5373=CARTESIAN_POINT ( 'NONE',  ( 27.99999999999999645, -49.14999999999999147, -53.92499999999967741 ) ) ;
#5443=CARTESIAN_POINT ( 'NONE',  ( 16.67080628287043709, -3.047499999999997211, -5.278424836066143655 ) ) ;
#5449=COLOUR_RGB ( '', 0.66274510, 0.83137255, 0.94901961) ;
#5493=CARTESIAN_POINT ( 'NONE',  ( 3.730677800976860414, -49.14999999999999147, -40.92499999999998295 ) ) ;
#5525=CARTESIAN_POINT ( 'NONE',  ( 27.70833333333333570, 3.047499999999997655, 5.278424836066143655 ) ) ;
#5542=( NAMED_UNIT ( * ) SI_UNIT ( $, .STERADIAN. ) SOLID_ANGLE_UNIT ( ) );
#5551=CARTESIAN_POINT ( 'NONE',  ( 13.12500000000000178, 6.094999999999989981, -1.119633336120465690E-15 ) ) ;
#5553=CARTESIAN_POINT ( 'NONE',  ( 1.586284118322663916, -3.036554765565917968, 5.760036735694805010 ) ) ;
#5594=PRESENTATION_STYLE_ASSIGNMENT (( #4852 ) ) ;
#5627=CARTESIAN_POINT ( 'NONE',  ( 131.8806778009765708, -49.14999999999999147, 40.92499999999998295 ) ) ;
#5640=CARTESIAN_POINT ( 'NONE',  ( 0.8183591370940052068, -52.14999999999999147, 41.64499999999997470 ) ) ;
#5645=CARTESIAN_POINT ( 'NONE',  ( 32.00456980810188412, 6.871911579029510442, -3.967499999999998916 ) ) ;
#5682=EDGE_CURVE ( 'NONE', #106911, #141737, #13233, .T. ) ;
#5691=CARTESIAN_POINT ( 'NONE',  ( 33.37456980810188156, 6.871911579029510442, -3.967499999999998916 ) ) ;
#5692=CARTESIAN_POINT ( 'NONE',  ( 11.20790314143521904, -6.871911579029513106, -3.967499999999993587 ) ) ;
#5727=CARTESIAN_POINT ( 'NONE',  ( 7.729166666666666075, -6.094999999999989093, 1.633150327867691542 ) ) ;
#5732=STYLED_ITEM ( 'NONE', ( #133041 ), #88424 ) ;
#5738=CARTESIAN_POINT ( 'NONE',  ( 2.999999999999999112, -1.600000000000012301, -20.40202195861969514 ) ) ;
#5747=CARTESIAN_POINT ( 'NONE',  ( 10.85873647476855197, 5.808823158059031044, -5.808823158059037262 ) ) ;
#5764=CARTESIAN_POINT ( 'NONE',  ( 5.979166666666666075, 6.094999999999988205, -1.633150327867694651 ) ) ;
#5814=PRESENTATION_STYLE_ASSIGNMENT (( #105159 ) ) ;
#5823=DIRECTION ( 'NONE',  ( 0.000000000000000000, -1.000000000000000000, -1.286409696682840916E-16 ) ) ;
#5840=ORIENTED_EDGE ( 'NONE', *, *, #768, .F. ) ;
#5842=FILL_AREA_STYLE_COLOUR ( '', #108488 ) ;
#5845=UNCERTAINTY_MEASURE_WITH_UNIT (LENGTH_MEASURE( 1.000000000000000082E-05 ), #115592, 'distance_accuracy_value', 'NONE');
#5849=VECTOR ( 'NONE', #77625, 1000.000000000000000 ) ;
#5860=CARTESIAN_POINT ( 'NONE',  ( 28.00000000000002487, -49.14999999999999147, 34.92500000000003268 ) ) ;
#5870=CARTESIAN_POINT ( 'NONE',  ( 152.4000000000000057, -17.48000000000005016, 33.92499999999998295 ) ) ;
#5887=FILL_AREA_STYLE_COLOUR ( '', #129432 ) ;
#5931=CARTESIAN_POINT ( 'NONE',  ( 26.40000000000000568, -17.48000000000005016, 33.92499999999998295 ) ) ;
#5974=( LENGTH_UNIT ( ) NAMED_UNIT ( * ) SI_UNIT ( .MILLI., .METRE. ) );
#5975=CARTESIAN_POINT ( 'NONE',  ( 12.46290314143521982, -3.967499999999994476, 6.871911579029513106 ) ) ;
#6008=CARTESIAN_POINT ( 'NONE',  ( 1.291236474768552966, -9.717572351234235426E-16, -7.934999999999990727 ) ) ;
#6022=CARTESIAN_POINT ( 'NONE',  ( 25.39999999999999858, -7.600000000000061817, 28.92499999999998650 ) ) ;
#6024=SURFACE_STYLE_USAGE ( .BOTH. , #103918 ) ;
#6042=VECTOR ( 'NONE', #92227, 1000.000000000000000 ) ;
#6062=ORIENTED_EDGE ( 'NONE', *, *, #94553, .T. ) ;
#6073=CARTESIAN_POINT ( 'NONE',  ( 156.1499999999997783, -52.14999999999999147, -34.92499999999975557 ) ) ;
#6085=ORIENTED_EDGE ( 'NONE', *, *, #43646, .F. ) ;
#6088=CARTESIAN_POINT ( 'NONE',  ( 184.1500000000000057, -14.29000000000013593, 12.69999999999954632 ) ) ;
#6110=( GEOMETRIC_REPRESENTATION_CONTEXT ( 3 ) GLOBAL_UNCERTAINTY_ASSIGNED_CONTEXT ( ( #66366 ) ) GLOBAL_UNIT_ASSIGNED_CONTEXT ( ( #12189, #133982, #23043 ) ) REPRESENTATION_CONTEXT ( 'NONE', 'WORKASPACE' ) );
#6142=CARTESIAN_POINT ( 'NONE',  ( 13.46247294953710494, -7.464222240803106570E-16, -6.094999999999989981 ) ) ;
#6157=ADVANCED_FACE ( 'NONE', ( #112419 ), #45761, .F. ) ;
#6160=ORIENTED_EDGE ( 'NONE', *, *, #23573, .T. ) ;
#6174=CARTESIAN_POINT ( 'NONE',  ( 30.16623647476855652, 7.934999999999990727, -1.457635852685135314E-15 ) ) ;
#6188=CARTESIAN_POINT ( 'NONE',  ( 0.7113915074146799356, -49.19295221407797669, -41.21232802154111141 ) ) ;
#6214=SURFACE_SIDE_STYLE ('',( #49800 ) ) ;
#6219=CARTESIAN_POINT ( 'NONE',  ( 20.85416666666666075, 1.633150327867695095, 6.094999999999988205 ) ) ;
#6238=FILL_AREA_STYLE ('',( #84582 ) ) ;
#6246=VECTOR ( 'NONE', #87593, 1000.000000000000000 ) ;
#6255=CARTESIAN_POINT ( 'NONE',  ( 184.1500000000000057, -30.18000000000009564, 15.92499999999935945 ) ) ;
#6288=ORIENTED_EDGE ( 'NONE', *, *, #47317, .F. ) ;
#6291=CARTESIAN_POINT ( 'NONE',  ( 11.85830628287044242, -1.633150327867709528, 6.094999999999979323 ) ) ;
#6324=AXIS2_PLACEMENT_3D ( 'NONE', #1990, #36804, #81050 ) ;
#6328=( NAMED_UNIT ( * ) PLANE_ANGLE_UNIT ( ) SI_UNIT ( $, .RADIAN. ) );
#6331=COLOUR_RGB ( '', 0.08235294, 0.09019608, 0.10196078) ;
#6333=CARTESIAN_POINT ( 'NONE',  ( 6.249569808101886004, 3.967499999999998916, 6.871911579029510442 ) ) ;
#6374=CARTESIAN_POINT ( 'NONE',  ( 30.16623647476855652, 7.934999999999990727, -1.457635852685135314E-15 ) ) ;
#6375=CARTESIAN_POINT ( 'NONE',  ( 10.04123647476855297, 0.000000000000000000, 7.934999999999990727 ) ) ;
#6398=( NAMED_UNIT ( * ) SI_UNIT ( $, .STERADIAN. ) SOLID_ANGLE_UNIT ( ) );
#6409=CARTESIAN_POINT ( 'NONE',  ( 123.3803752239310541, -44.19516442798762768, 34.92499999999998295 ) ) ;
#6427=AXIS2_PLACEMENT_3D ( 'NONE', #98853, #42374, #53209 ) ;
#6432=CARTESIAN_POINT ( 'NONE',  ( 5.317069808101886785, -2.126176841940956130, 7.934999999999990727 ) ) ;
#6501=DIRECTION ( 'NONE',  ( 0.000000000000000000, 0.000000000000000000, 1.000000000000000000 ) ) ;
#6503=CARTESIAN_POINT ( 'NONE',  ( 11.15040314143521982, 7.934999999999989839, -2.126176841940961904 ) ) ;
#6513=ORIENTED_EDGE ( 'NONE', *, *, #369, .T. ) ;
#6514=CARTESIAN_POINT ( 'NONE',  ( 151.4000000000000057, -16.48000000000005016, -33.92499999999998295 ) ) ;
#6516=CARTESIAN_POINT ( 'NONE',  ( 183.7681020908649714, -51.95642703809001972, -39.54367611436801866 ) ) ;
#6545=CARTESIAN_POINT ( 'NONE',  ( 2.770833333333333925, 6.094999999999991758, 1.633150327867686880 ) ) ;
#6560=ORIENTED_EDGE ( 'NONE', *, *, #1789, .T. ) ;
#6561=VERTEX_POINT ( 'NONE', #17429 ) ;
#6582=DIRECTION ( 'NONE',  ( -1.000000000000000000, 0.000000000000000000, 0.000000000000000000 ) ) ;
#6585=FILL_AREA_STYLE_COLOUR ( '', #97108 ) ;
#6595=LINE ( 'NONE', #116113, #25603 ) ;
#6656=AXIS2_PLACEMENT_3D ( 'NONE', #90986, #135214, #11217 ) ;
#6682=CARTESIAN_POINT ( 'NONE',  ( 11.44206980810188767, 7.934999999999993392, 2.126176841940951689 ) ) ;
#6713=CARTESIAN_POINT ( 'NONE',  ( 10.62456980810188689, -6.871911579029512218, 3.967499999999996252 ) ) ;
#6731=( GEOMETRIC_REPRESENTATION_CONTEXT ( 3 ) GLOBAL_UNCERTAINTY_ASSIGNED_CONTEXT ( ( #30139 ) ) GLOBAL_UNIT_ASSIGNED_CONTEXT ( ( #121693, #97057, #63788 ) ) REPRESENTATION_CONTEXT ( 'NONE', 'WORKASPACE' ) );
#6758=PRESENTATION_STYLE_ASSIGNMENT (( #63376 ) ) ;
#6799=VECTOR ( 'NONE', #44639, 1000.000000000000000 ) ;
#6833=DIRECTION ( 'NONE',  ( 0.000000000000000000, 0.000000000000000000, 1.000000000000000000 ) ) ;
#6834=CARTESIAN_POINT ( 'NONE',  ( 2.999999999999999112, -5.520864266206504263E-14, 0.000000000000000000 ) ) ;
#6855=CARTESIAN_POINT ( 'NONE',  ( 16.23330628287043353, -6.094999999999989981, -1.633150327867689100 ) ) ;
#6930=CARTESIAN_POINT ( 'NONE',  ( 34.41666666666667140, 5.278424836066147208, 3.047499999999990550 ) ) ;
#6952=CARTESIAN_POINT ( 'NONE',  ( 1.573529187797693574, -2.874494765961987497, 5.856845438429902018 ) ) ;
#6955=FACE_OUTER_BOUND ( 'NONE', #44327, .T. ) ;
#6994=EDGE_CURVE ( 'NONE', #62992, #119600, #73181, .T. ) ;
#6998=CARTESIAN_POINT ( 'NONE',  ( 25.39999999999999858, -5.520864266206504263E-14, 0.000000000000000000 ) ) ;
#7015=EDGE_CURVE ( 'NONE', #87517, #66916, #85704, .T. ) ;
#7031=FACE_BOUND ( 'NONE', #121992, .T. ) ;
#7044=CIRCLE ( 'NONE', #88135, 5.999999999999998224 ) ;
#7051=CARTESIAN_POINT ( 'NONE',  ( 3.010427959778288365, -48.08977582060914813, 37.49964900842618931 ) ) ;
#7054=CARTESIAN_POINT ( 'NONE',  ( 5.228736474768552078, 5.808823158059031044, -5.808823158059038150 ) ) ;
#7063=VECTOR ( 'NONE', #56221, 1000.000000000000000 ) ;
#7090=UNCERTAINTY_MEASURE_WITH_UNIT (LENGTH_MEASURE( 1.000000000000000082E-05 ), #95434, 'distance_accuracy_value', 'NONE');
#7102=CARTESIAN_POINT ( 'NONE',  ( 7.583333333333333925, -5.278424836066144543, 3.047499999999995879 ) ) ;
#7104=CARTESIAN_POINT ( 'NONE',  ( 10.18706980810188512, -2.126176841940956130, 7.934999999999990727 ) ) ;
#7115=AXIS2_PLACEMENT_3D ( 'NONE', #136900, #70271, #2058 ) ;
#7130=CARTESIAN_POINT ( 'NONE',  ( 55.64345981607718272, -48.97294124528174564, 39.12804664298385404 ) ) ;
#7139=COLOUR_RGB ( '', 0.09019608, 0.27058824, 0.51372549) ;
#7164=CARTESIAN_POINT ( 'NONE',  ( 4.587903141435219823, 6.871911579029515771, 3.967499999999989146 ) ) ;
#7182=CARTESIAN_POINT ( 'NONE',  ( 25.39999999999999858, -1.600000000000060929, 28.92500000000001847 ) ) ;
#7185=SURFACE_SIDE_STYLE ('',( #73217 ) ) ;
#7216=CIRCLE ( 'NONE', #134568, 6.094999999999989093 ) ;
#7227=SURFACE_STYLE_USAGE ( .BOTH. , #142773 ) ;
#7237=CARTESIAN_POINT ( 'NONE',  ( 5.171236474768553748, 0.000000000000000000, 7.934999999999990727 ) ) ;
#7266=VECTOR ( 'NONE', #105847, 1000.000000000000000 ) ;
#7322=( NAMED_UNIT ( * ) PLANE_ANGLE_UNIT ( ) SI_UNIT ( $, .RADIAN. ) );
#7335=( NAMED_UNIT ( * ) PLANE_ANGLE_UNIT ( ) SI_UNIT ( $, .RADIAN. ) );
#7380=CARTESIAN_POINT ( 'NONE',  ( 3.730677800976790248, -49.14999999999999147, 40.92499999999998295 ) ) ;
#7383=CARTESIAN_POINT ( 'NONE',  ( 181.1500000000000057, -43.14999999999999147, -40.92499999999998295 ) ) ;
#7398=ADVANCED_FACE ( 'NONE', ( #73054 ), #116524, .T. ) ;
#7420=CARTESIAN_POINT ( 'NONE',  ( 16.10873647476855552, -5.808823158059033709, 5.808823158059035485 ) ) ;
#7452=CARTESIAN_POINT ( 'NONE',  ( 16.02040314143522082, 7.934999999999989839, -2.126176841940961904 ) ) ;
#7471=VECTOR ( 'NONE', #37741, 1000.000000000000000 ) ;
#7524=SURFACE_SIDE_STYLE ('',( #131478 ) ) ;
#7536=CARTESIAN_POINT ( 'NONE',  ( 153.4000000000000057, -1.600000000000094458, 33.92499999999998295 ) ) ;
#7541=SURFACE_STYLE_FILL_AREA ( #18402 ) ;
#7593=CARTESIAN_POINT ( 'NONE',  ( 15.64997294953710671, -4.461849672132299105, 4.461849672132299993 ) ) ;
#7618=ORIENTED_EDGE ( 'NONE', *, *, #116171, .F. ) ;
#7623=CARTESIAN_POINT ( 'NONE',  ( 30.02040314143521726, 7.934999999999989839, -2.126176841940961904 ) ) ;
#7639=CARTESIAN_POINT ( 'NONE',  ( 0.5414528859221161561, -52.10163751122234999, -40.43817685073778279 ) ) ;
#7647=DIRECTION ( 'NONE',  ( 0.000000000000000000, -2.556434596176436521E-15, -1.000000000000000000 ) ) ;
#7651=COLOUR_RGB ( '', 0.08235294, 0.09019608, 0.10196078) ;
#7662=CARTESIAN_POINT ( 'NONE',  ( 0.000000000000000000, 0.000000000000000000, 0.000000000000000000 ) ) ;
#7666=FILL_AREA_STYLE_COLOUR ( '', #90669 ) ;
#7676=CARTESIAN_POINT ( 'NONE',  ( 28.43750000000000355, -4.461849672132299105, 4.461849672132299993 ) ) ;
#7686=CIRCLE ( 'NONE', #125798, 5.999999999999998224 ) ;
#7736=CARTESIAN_POINT ( 'NONE',  ( 180.4193221990230143, -49.14999999999999147, 40.92499999999998295 ) ) ;
#7748=CARTESIAN_POINT ( 'NONE',  ( 122.6835989386367345, -57.15000000000009095, 34.92499999999998295 ) ) ;
#7776=( LENGTH_UNIT ( ) NAMED_UNIT ( * ) SI_UNIT ( .MILLI., .METRE. ) );
#7786=CARTESIAN_POINT ( 'NONE',  ( 3.100164867288737636, -48.63026969829241608, 38.45492102172730142 ) ) ;
#7790=CARTESIAN_POINT ( 'NONE',  ( 8.291236474768552966, -9.717572351234235426E-16, -7.934999999999990727 ) ) ;
#7802=( NAMED_UNIT ( * ) SI_UNIT ( $, .STERADIAN. ) SOLID_ANGLE_UNIT ( ) );
#7820=CARTESIAN_POINT ( 'NONE',  ( 56.00844637038503748, -48.60795469097138977, -38.18754904900253422 ) ) ;
#7840=CARTESIAN_POINT ( 'NONE',  ( 3.500000000000000444, 0.000000000000000000, 6.094999999999989981 ) ) ;
#7841=CARTESIAN_POINT ( 'NONE',  ( 7.416236474768552078, -7.934999999999990727, 4.858786175617117713E-16 ) ) ;
#7867=CARTESIAN_POINT ( 'NONE',  ( 59.09089496824217491, -46.71325913968129129, 35.40428284070832632 ) ) ;
#7893=CARTESIAN_POINT ( 'NONE',  ( 7.942069808101886785, 7.934999999999992504, 2.126176841940951689 ) ) ;
#7908=AXIS2_PLACEMENT_3D ( 'NONE', #106381, #84678, #141939 ) ;
#7913=( LENGTH_UNIT ( ) NAMED_UNIT ( * ) SI_UNIT ( .MILLI., .METRE. ) );
#7935=FACE_BOUND ( 'NONE', #73889, .T. ) ;
#7954=DIRECTION ( 'NONE',  ( 0.000000000000000000, 0.000000000000000000, -1.000000000000000000 ) ) ;
#7962=CARTESIAN_POINT ( 'NONE',  ( 8.087903141435219823, 6.871911579029515771, 3.967499999999989146 ) ) ;
#7969=EDGE_CURVE ( 'NONE', #79775, #53362, #53220, .T. ) ;
#7983=EDGE_LOOP ( 'NONE', ( #79443, #2245, #129630, #14927 ) ) ;
#8089=SURFACE_STYLE_FILL_AREA ( #64646 ) ;
#8106=COLOUR_RGB ( '', 0.09019608, 0.27058824, 0.51372549) ;
#8127=CARTESIAN_POINT ( 'NONE',  ( 22.37956980810188767, 3.967499999999998916, 6.871911579029510442 ) ) ;
#8154=CARTESIAN_POINT ( 'NONE',  ( 4.812500000000000000, -4.461849672132299993, -4.461849672132299105 ) ) ;
#8161=CARTESIAN_POINT ( 'NONE',  ( 13.39540314143521904, 2.126176841940962348, 7.934999999999989839 ) ) ;
#8174=FILL_AREA_STYLE_COLOUR ( '', #125320 ) ;
#8195=CARTESIAN_POINT ( 'NONE',  ( 10.50000000000000000, 0.000000000000000000, 6.094999999999989981 ) ) ;
#8277=( NAMED_UNIT ( * ) PLANE_ANGLE_UNIT ( ) SI_UNIT ( $, .RADIAN. ) );
#8280=DIRECTION ( 'NONE',  ( 0.000000000000000000, -1.000000000000000000, 0.000000000000000000 ) ) ;
#8288=EDGE_CURVE ( 'NONE', #26834, #50573, #47239, .T. ) ;
#8290=CARTESIAN_POINT ( 'NONE',  ( 26.44163961620376924, -6.094999999999989093, 1.633150327867691765 ) ) ;
#8322=CARTESIAN_POINT ( 'NONE',  ( 32.35373647476855297, -5.808823158059035485, -5.808823158059033709 ) ) ;
#8328=VERTEX_POINT ( 'NONE', #42032 ) ;
#8366=CARTESIAN_POINT ( 'NONE',  ( 30.62500000000000355, 6.094999999999989981, -1.119633336120465690E-15 ) ) ;
#8371=ORIENTED_EDGE ( 'NONE', *, *, #127305, .T. ) ;
#8385=CARTESIAN_POINT ( 'NONE',  ( 131.8806778009766276, -49.14999999999999147, -40.92499999999998295 ) ) ;
#8408=STYLED_ITEM ( 'NONE', ( #109723 ), #111305 ) ;
#8412=SURFACE_STYLE_FILL_AREA ( #41087 ) ;
#8456=LINE ( 'NONE', #83218, #99586 ) ;
#8477=CARTESIAN_POINT ( 'NONE',  ( 0.7113915074196556221, -49.19295221407733010, 41.21232802153977559 ) ) ;
#8480=CARTESIAN_POINT ( 'NONE',  ( 2.457903141435219485, 6.871911579029515771, 3.967499999999989146 ) ) ;
#8504=CARTESIAN_POINT ( 'NONE',  ( 55.47138350052864553, -49.14501756083437556, -40.36361034346621324 ) ) ;
#8518=( LENGTH_UNIT ( ) NAMED_UNIT ( * ) SI_UNIT ( .MILLI., .METRE. ) );
#8522=CARTESIAN_POINT ( 'NONE',  ( 3.791666666666666963, -3.047499999999994547, 5.278424836066145431 ) ) ;
#8523=CARTESIAN_POINT ( 'NONE',  ( 13.10373647476855297, 5.808823158059035485, 5.808823158059032821 ) ) ;
#8535=CARTESIAN_POINT ( 'NONE',  ( 131.3130295073068226, -48.90295371244954481, -39.18578444878617262 ) ) ;
#8540=EDGE_CURVE ( 'NONE', #93434, #68280, #91259, .T. ) ;
#8542=CARTESIAN_POINT ( 'NONE',  ( -1.807144792967049773E-15, -50.24077216217763464, 35.40405119785170029 ) ) ;
#8549=CARTESIAN_POINT ( 'NONE',  ( 54.24578869845078088, -47.96374157527325366, 37.32649486623284929 ) ) ;
#8556=CARTESIAN_POINT ( 'NONE',  ( 130.9531400719712906, -48.66302742222553235, 38.53170190052306054 ) ) ;
#8575=CARTESIAN_POINT ( 'NONE',  ( 15.96290314143521805, -3.967499999999994476, 6.871911579029513106 ) ) ;
#8597=VERTEX_POINT ( 'NONE', #13643 ) ;
#8598=SURFACE_STYLE_FILL_AREA ( #31141 ) ;
#8601=CARTESIAN_POINT ( 'NONE',  ( 25.39999999999999858, 4.836323036001208386, -6.294117125145909597 ) ) ;
#8609=CIRCLE ( 'NONE', #27177, 1.000000000000000888 ) ;
#8616=DIRECTION ( 'NONE',  ( -1.000000000000000000, -0.000000000000000000, -0.000000000000000000 ) ) ;
#8632=ORIENTED_EDGE ( 'NONE', *, *, #28784, .F. ) ;
#8644=EDGE_LOOP ( 'NONE', ( #129095, #201 ) ) ;
#8650=CARTESIAN_POINT ( 'NONE',  ( 12.46290314143521982, -3.967499999999994476, 6.871911579029513106 ) ) ;
#8658=CARTESIAN_POINT ( 'NONE',  ( 131.7507865773015681, -49.14999999999999147, -40.57473644908944266 ) ) ;
#8663=CARTESIAN_POINT ( 'NONE',  ( 61.46640106136302961, -43.14999999999999147, -34.92499999999998295 ) ) ;
#8687=DIRECTION ( 'NONE',  ( 0.000000000000000000, 0.000000000000000000, -1.000000000000000000 ) ) ;
#8723=VERTEX_POINT ( 'NONE', #29518 ) ;
#8749=AXIS2_PLACEMENT_3D ( 'NONE', #81267, #103672, #127610 ) ;
#8773=ADVANCED_FACE ( 'NONE', ( #19375 ), #74469, .T. ) ;
#8790=DIRECTION ( 'NONE',  ( 0.9843059135694992579, 0.000000000000000000, -0.1764705882353009014 ) ) ;
#8812=EDGE_CURVE ( 'NONE', #80652, #31146, #92844, .T. ) ;
#8813=CARTESIAN_POINT ( 'NONE',  ( 15.52540314143522160, 2.126176841940962348, 7.934999999999989839 ) ) ;
#8836=CARTESIAN_POINT ( 'NONE',  ( 3.500000000000000444, 0.000000000000000000, 6.094999999999989981 ) ) ;
#8842=CARTESIAN_POINT ( 'NONE',  ( 14.56206980810188334, -7.934999999999991616, -2.126176841940955242 ) ) ;
#8873=SURFACE_STYLE_FILL_AREA ( #50495 ) ;
#8906=CARTESIAN_POINT ( 'NONE',  ( 9.524972949537108491, -4.461849672132299993, -4.461849672132299105 ) ) ;
#8911=FILL_AREA_STYLE_COLOUR ( '', #67955 ) ;
#8925=CARTESIAN_POINT ( 'NONE',  ( 0.000000000000000000, 0.000000000000000000, 0.000000000000000000 ) ) ;
#8983=CARTESIAN_POINT ( 'NONE',  ( 28.33747294953710849, 6.094999999999989981, -1.119633336120465690E-15 ) ) ;
#9009=STYLED_ITEM ( 'NONE', ( #13081 ), #113213 ) ;
#9058=CIRCLE ( 'NONE', #90127, 3.999999999999996447 ) ;
#9059=COLOUR_RGB ( '', 0.72549020, 0.75294118, 0.79215686) ;
#9072=CARTESIAN_POINT ( 'NONE',  ( 30.33333333333333570, 5.278424836066143655, -3.047499999999997655 ) ) ;
#9132=CARTESIAN_POINT ( 'NONE',  ( 183.7681020908654261, -51.95642703808907470, 39.54367611436589414 ) ) ;
#9162=CARTESIAN_POINT ( 'NONE',  ( -1.558360383796227655, -6.094999999999989093, 1.633150327867691765 ) ) ;
#9190=CARTESIAN_POINT ( 'NONE',  ( 11.93706980810188689, 2.126176841940952134, -7.934999999999993392 ) ) ;
#9209=EDGE_LOOP ( 'NONE', ( #126002, #32613, #23661, #139940 ) ) ;
#9224=( GEOMETRIC_REPRESENTATION_CONTEXT ( 3 ) GLOBAL_UNCERTAINTY_ASSIGNED_CONTEXT ( ( #24410 ) ) GLOBAL_UNIT_ASSIGNED_CONTEXT ( ( #34609, #112183, #133921 ) ) REPRESENTATION_CONTEXT ( 'NONE', 'WORKASPACE' ) );
#9229=DIRECTION ( 'NONE',  ( 0.000000000000000000, 0.000000000000000000, 1.000000000000000000 ) ) ;
#9235=CARTESIAN_POINT ( 'NONE',  ( 1.020833333333333481, -6.094999999999989981, -1.633150327867689100 ) ) ;
#9236=CARTESIAN_POINT ( 'NONE',  ( 18.06206980810188867, -7.934999999999990727, -2.126176841940955242 ) ) ;
#9238=PLANE ( 'NONE',  #30410 ) ;
#9243=VECTOR ( 'NONE', #115543, 1000.000000000000000 ) ;
#9275=CARTESIAN_POINT ( 'NONE',  ( 128.5894344200537489, -52.00875322212550600, 39.86617647058824332 ) ) ;
#9293=CARTESIAN_POINT ( 'NONE',  ( 13.92123647476855197, -9.717572351234235426E-16, -7.934999999999990727 ) ) ;
#9295=CARTESIAN_POINT ( 'NONE',  ( 160.4290834833332440, 26.96999999999994913, 34.92499999999999716 ) ) ;
#9308=ORIENTED_EDGE ( 'NONE', *, *, #86393, .T. ) ;
#9323=CARTESIAN_POINT ( 'NONE',  ( 25.40000000000001279, 0.9275341018601235277, -7.891049174277950051 ) ) ;
#9331=VERTEX_POINT ( 'NONE', #115644 ) ;
#9371=VECTOR ( 'NONE', #19258, 1000.000000000000000 ) ;
#9372=CARTESIAN_POINT ( 'NONE',  ( 9.108736474768550195, -5.808823158059033709, 5.808823158059035485 ) ) ;
#9410=CARTESIAN_POINT ( 'NONE',  ( 0.1600000000000004752, -2.314171071560278126, -7.597438125929392605 ) ) ;
#9413=FILL_AREA_STYLE_COLOUR ( '', #32192 ) ;
#9438=STYLED_ITEM ( 'NONE', ( #80911 ), #115316 ) ;
#9449=CARTESIAN_POINT ( 'NONE',  ( 23.91666666666666785, 5.278424836066147208, 3.047499999999990550 ) ) ;
#9497=CARTESIAN_POINT ( 'NONE',  ( 156.1500000000000057, -49.14999999999999147, -53.92499999999968452 ) ) ;
#9512=FACE_OUTER_BOUND ( 'NONE', #24619, .T. ) ;
#9523=DIRECTION ( 'NONE',  ( -0.000000000000000000, 1.000000000000000000, -0.000000000000000000 ) ) ;
#9556=CARTESIAN_POINT ( 'NONE',  ( 17.71290314143521982, 3.967499999999992699, -6.871911579029513994 ) ) ;
#9588=VERTEX_POINT ( 'NONE', #80770 ) ;
#9666=CARTESIAN_POINT ( 'NONE',  ( 9.233306282870437087, -6.094999999999989981, -1.633150327867689322 ) ) ;
#9693=ORIENTED_EDGE ( 'NONE', *, *, #71235, .T. ) ;
#9719=DIRECTION ( 'NONE',  ( 0.000000000000000000, -1.734723475976807686E-15, 1.000000000000000000 ) ) ;
#9740=CARTESIAN_POINT ( 'NONE',  ( 26.73330628287044064, -6.094999999999989981, -1.633150327867689100 ) ) ;
#9829=CARTESIAN_POINT ( 'NONE',  ( 32.37500000000000000, -6.094999999999989981, 3.732111120401553285E-16 ) ) ;
#9837=( LENGTH_UNIT ( ) NAMED_UNIT ( * ) SI_UNIT ( .MILLI., .METRE. ) );
#9840=STYLED_ITEM ( 'NONE', ( #54637 ), #79516 ) ;
#9847=CARTESIAN_POINT ( 'NONE',  ( 128.5894344200537773, -52.00875322212549179, -39.86617647058817226 ) ) ;
#9865=DIRECTION ( 'NONE',  ( -0.000000000000000000, 1.000000000000000000, 0.000000000000000000 ) ) ;
#9873=VECTOR ( 'NONE', #89713, 1000.000000000000000 ) ;
#9883=AXIS2_PLACEMENT_3D ( 'NONE', #11182, #88811, #46771 ) ;
#9888=SURFACE_STYLE_FILL_AREA ( #121044 ) ;
#9908=EDGE_CURVE ( 'NONE', #26733, #80864, #135693, .T. ) ;
#9945=CARTESIAN_POINT ( 'NONE',  ( 17.18706980810188867, -2.126176841940956130, 7.934999999999991616 ) ) ;
#9947=CARTESIAN_POINT ( 'NONE',  ( 28.00000000000002487, -49.14999999999999147, -34.92499999999976978 ) ) ;
#9953=CARTESIAN_POINT ( 'NONE',  ( 19.97916666666666785, 6.094999999999988205, -1.633150327867694651 ) ) ;
#9954=FILL_AREA_STYLE ('',( #20106 ) ) ;
#9980=FACE_OUTER_BOUND ( 'NONE', #96212, .T. ) ;
#9986=DIRECTION ( 'NONE',  ( 0.000000000000000000, -1.000000000000000000, 0.000000000000000000 ) ) ;
#9996=CARTESIAN_POINT ( 'NONE',  ( 5.833333333333333925, 5.278424836066143655, -3.047499999999997655 ) ) ;
#9997=CARTESIAN_POINT ( 'NONE',  ( 20.39540314143521726, 2.126176841940962348, 7.934999999999988951 ) ) ;
#9998=SURFACE_STYLE_USAGE ( .BOTH. , #120150 ) ;
#10010=CARTESIAN_POINT ( 'NONE',  ( 131.4501442085549456, -48.99436351328196082, -39.52330221398180754 ) ) ;
#10017=DIRECTION ( 'NONE',  ( -0.000000000000000000, -4.625929269271485322E-15, -1.000000000000000000 ) ) ;
#10021=DIRECTION ( 'NONE',  ( -0.9843059135694992579, 0.000000000000000000, -0.1764705882353013178 ) ) ;
#10032=CARTESIAN_POINT ( 'NONE',  ( 128.0481121284663857, -51.19676978474465301, 38.21513923100059884 ) ) ;
#10033=MECHANICAL_DESIGN_GEOMETRIC_PRESENTATION_REPRESENTATION('',(#24014),#63375);
#10070=DIRECTION ( 'NONE',  ( -1.000000000000000000, -0.000000000000000000, -0.000000000000000000 ) ) ;
#10071=ORIENTED_EDGE ( 'NONE', *, *, #69687, .T. ) ;
#10103=ORIENTED_EDGE ( 'NONE', *, *, #56682, .F. ) ;
#10122=CARTESIAN_POINT ( 'NONE',  ( 22.23373647476855197, 5.808823158059036373, 5.808823158059032821 ) ) ;
#10142=DIRECTION ( 'NONE',  ( 0.000000000000000000, 0.000000000000000000, -1.000000000000000000 ) ) ;
#10188=CARTESIAN_POINT ( 'NONE',  ( 22.75000000000000355, -7.464222240803106570E-16, -6.094999999999989981 ) ) ;
#10202=DIRECTION ( 'NONE',  ( -1.000000000000000000, -0.000000000000000000, 0.000000000000000000 ) ) ;
#10241=CARTESIAN_POINT ( 'NONE',  ( 3.225639847634929946, -48.88932940808381744, 39.16623080367947551 ) ) ;
#10254=FILL_AREA_STYLE_COLOUR ( '', #19489 ) ;
#10280=COLOUR_RGB ( '', 0.40784314, 0.44705882, 0.49803922) ;
#10284=CARTESIAN_POINT ( 'NONE',  ( 19.75456980810189123, -6.871911579029512218, 3.967499999999996252 ) ) ;
#10323=SURFACE_SIDE_STYLE ('',( #119783 ) ) ;
#10379=CARTESIAN_POINT ( 'NONE',  ( 9.816639616203772789, -1.633150327867681995, -6.094999999999993534 ) ) ;
#10385=( NAMED_UNIT ( * ) PLANE_ANGLE_UNIT ( ) SI_UNIT ( $, .RADIAN. ) );
#10427=CARTESIAN_POINT ( 'NONE',  ( 0.000000000000000000, -43.14999999999999147, -31.92499999999998295 ) ) ;
#10440=CARTESIAN_POINT ( 'NONE',  ( 25.39999999999999858, -43.14999999999999147, -40.92499999999998295 ) ) ;
#10449=CARTESIAN_POINT ( 'NONE',  ( 26.87913961620377634, -5.278424836066145431, -3.047499999999993658 ) ) ;
#10462=DIRECTION ( 'NONE',  ( -1.000000000000000000, -0.000000000000000000, -0.000000000000000000 ) ) ;
#10475=DIRECTION ( 'NONE',  ( 0.000000000000000000, 0.000000000000000000, -1.000000000000000000 ) ) ;
#10492=CARTESIAN_POINT ( 'NONE',  ( 55.28643332384051945, -49.19207878844169812, 41.22112633374686652 ) ) ;
#10518=STYLED_ITEM ( 'NONE', ( #99147 ), #120916 ) ;
#10554=ORIENTED_EDGE ( 'NONE', *, *, #86393, .F. ) ;
#10586=CARTESIAN_POINT ( 'NONE',  ( 183.6687791239614569, -49.11951764990740088, 40.13200514437710353 ) ) ;
#10596=AXIS2_PLACEMENT_3D ( 'NONE', #137744, #115212, #26115 ) ;
#10615=CARTESIAN_POINT ( 'NONE',  ( 1.212472949537106048, 0.000000000000000000, 6.094999999999989981 ) ) ;
#10639=ORIENTED_EDGE ( 'NONE', *, *, #124402, .F. ) ;
#10642=CARTESIAN_POINT ( 'NONE',  ( 9.895403141435220817, 2.126176841940962348, 7.934999999999989839 ) ) ;
#10648=ORIENTED_EDGE ( 'NONE', *, *, #116500, .T. ) ;
#10649=( NAMED_UNIT ( * ) SI_UNIT ( $, .STERADIAN. ) SOLID_ANGLE_UNIT ( ) );
#10682=CARTESIAN_POINT ( 'NONE',  ( 11.08333333333333393, -5.278424836066144543, 3.047499999999995879 ) ) ;
#10683=CARTESIAN_POINT ( 'NONE',  ( 14.85373647476855297, -5.808823158059035485, -5.808823158059033709 ) ) ;
#10706=SURFACE_SIDE_STYLE ('',( #15515 ) ) ;
#10707=FILL_AREA_STYLE_COLOUR ( '', #121557 ) ;
#10722=CARTESIAN_POINT ( 'NONE',  ( 131.4501442085630742, -48.99436351328139239, 39.52330221397870247 ) ) ;
#10739=CARTESIAN_POINT ( 'NONE',  ( 18.87956980810189123, 3.967499999999998916, 6.871911579029510442 ) ) ;
#10757=FILL_AREA_STYLE_COLOUR ( '', #50726 ) ;
#10788=DIRECTION ( 'NONE',  ( 1.000000000000000000, 0.000000000000000000, 0.000000000000000000 ) ) ;
#10808=VECTOR ( 'NONE', #94018, 1000.000000000000000 ) ;
#10813=CARTESIAN_POINT ( 'NONE',  ( 17.71290314143521982, 3.967499999999992699, -6.871911579029513994 ) ) ;
#10899=ORIENTED_EDGE ( 'NONE', *, *, #106226, .T. ) ;
#10944=AXIS2_PLACEMENT_3D ( 'NONE', #23122, #33373, #67409 ) ;
#10972=DIRECTION ( 'NONE',  ( 0.000000000000000000, -1.000000000000000000, 0.000000000000000000 ) ) ;
#10975=CARTESIAN_POINT ( 'NONE',  ( 30.10873647476854842, -5.808823158059033709, 5.808823158059035485 ) ) ;
#10985=CARTESIAN_POINT ( 'NONE',  ( 25.39999999999999858, 7.464222240803104598E-16, -6.094999999999989093 ) ) ;
#10990=ORIENTED_EDGE ( 'NONE', *, *, #47309, .T. ) ;
#10994=CARTESIAN_POINT ( 'NONE',  ( 6.462472949537106715, -7.464222240803106570E-16, -6.094999999999989981 ) ) ;
#11010=ORIENTED_EDGE ( 'NONE', *, *, #89778, .T. ) ;
#11011=COLOUR_RGB ( '', 0.09019608, 0.27058824, 0.51372549) ;
#11030=( BOUNDED_CURVE ( )  B_SPLINE_CURVE ( 2, ( #131040, #89662, #142627, #99085, #120854, #9953, #43320, #133890, #45484, #54225, #32442, #55625, #100557 ),
 .UNSPECIFIED., .F., .T. ) 
 B_SPLINE_CURVE_WITH_KNOTS ( ( 3, 2, 2, 2, 2, 2, 3 ),
 ( 0.5500000000000001554, 0.5583333333333334592, 0.5666666666666667629, 0.5750000000000000666, 0.5833333333333334814, 0.5916666666666667851, 0.6000000000000000888 ),
 .UNSPECIFIED. ) 
 CURVE ( )  GEOMETRIC_REPRESENTATION_ITEM ( )  RATIONAL_B_SPLINE_CURVE ( ( 0.9999999999999995559, 0.9659258262890687563, 1.000000000000000000, 0.9659258262890683122, 1.000000000000000000, 0.9659258262890683122, 1.000000000000000000, 0.9659258262890683122, 1.000000000000000000, 0.9659258262890683122, 1.000000000000000000, 0.9659258262890678681, 1.000000000000000444 ) ) 
 REPRESENTATION_ITEM ( '' )  );
#11040=DIRECTION ( 'NONE',  ( -1.000000000000000000, -0.000000000000000000, -0.000000000000000000 ) ) ;
#11053=EDGE_CURVE ( 'NONE', #113523, #127303, #66268, .T. ) ;
#11054=DIRECTION ( 'NONE',  ( 1.000000000000000000, 0.000000000000000000, 0.000000000000000000 ) ) ;
#11064=CYLINDRICAL_SURFACE ( 'NONE', #133604, 5.999999999999998224 ) ;
#11081=( NAMED_UNIT ( * ) SI_UNIT ( $, .STERADIAN. ) SOLID_ANGLE_UNIT ( ) );
#11130=FILL_AREA_STYLE_COLOUR ( '', #55949 ) ;
#11131=VECTOR ( 'NONE', #98065, 1000.000000000000000 ) ;
#11137=ORIENTED_EDGE ( 'NONE', *, *, #785, .F. ) ;
#11138=CARTESIAN_POINT ( 'NONE',  ( 127.2418942207595194, -46.18886352141515772, -34.92499999999998295 ) ) ;
#11140=CARTESIAN_POINT ( 'NONE',  ( 21.19163961620376924, 6.094999999999988205, -1.633150327867694651 ) ) ;
#11148=ORIENTED_EDGE ( 'NONE', *, *, #1454, .T. ) ;
#11179=FACE_OUTER_BOUND ( 'NONE', #19784, .T. ) ;
#11182=CARTESIAN_POINT ( 'NONE',  ( 131.5423521607622490, -52.00875322212550600, 39.33676470588235929 ) ) ;
#11183=SURFACE_SIDE_STYLE ('',( #91477 ) ) ;
#11209=UNCERTAINTY_MEASURE_WITH_UNIT (LENGTH_MEASURE( 1.000000000000000082E-05 ), #69662, 'distance_accuracy_value', 'NONE');
#11210=MECHANICAL_DESIGN_GEOMETRIC_PRESENTATION_REPRESENTATION('',(#29753),#129311);
#11217=DIRECTION ( 'NONE',  ( 0.9707728879609256456, 0.000000000000000000, -0.2400000000000085398 ) ) ;
#11233=DIRECTION ( 'NONE',  ( 0.000000000000000000, 0.000000000000000000, 1.000000000000000000 ) ) ;
#11247=CARTESIAN_POINT ( 'NONE',  ( 128.9683591370938416, -52.14999999999999147, -41.64500000000001023 ) ) ;
#11249=B_SPLINE_CURVE_WITH_KNOTS ( 'NONE', 3,
 ( #96614, #51024, #139494, #140854, #82244, #38716, #82939, #11765 ),
 .UNSPECIFIED., .F., .F.,
 ( 4, 2, 2, 4 ),
 ( 2.778266744796018861E-17, 0.001415444524343407963, 0.002123166786515097524, 0.002830889048686786869 ),
 .UNSPECIFIED. ) ;
#11271=EDGE_CURVE ( 'NONE', #65560, #18319, #31609, .T. ) ;
#11297=VECTOR ( 'NONE', #38101, 1000.000000000000000 ) ;
#11312=CARTESIAN_POINT ( 'NONE',  ( -0.8291937171295610254, -3.047499999999997211, -5.278424836066143655 ) ) ;
#11327=VERTEX_POINT ( 'NONE', #106793 ) ;
#11342=CARTESIAN_POINT ( 'NONE',  ( 15.58290314143522082, 3.967499999999992699, -6.871911579029513994 ) ) ;
#11384=CARTESIAN_POINT ( 'NONE',  ( 13.70833333333333393, 3.047499999999997655, 5.278424836066143655 ) ) ;
#11399=( NAMED_UNIT ( * ) SI_UNIT ( $, .STERADIAN. ) SOLID_ANGLE_UNIT ( ) );
#11402=CIRCLE ( 'NONE', #13686, 3.000000000000000444 ) ;
#11451=CARTESIAN_POINT ( 'NONE',  ( 15.23373647476855375, 5.808823158059035485, 5.808823158059032821 ) ) ;
#11455=DIRECTION ( 'NONE',  ( 0.000000000000000000, 1.000000000000000000, 0.000000000000000000 ) ) ;
#11467=EDGE_LOOP ( 'NONE', ( #129244, #91493, #71513, #39499 ) ) ;
#11519=CARTESIAN_POINT ( 'NONE',  ( 14.79623647476855375, 7.934999999999990727, -1.457635852685135314E-15 ) ) ;
#11554=UNCERTAINTY_MEASURE_WITH_UNIT (LENGTH_MEASURE( 1.000000000000000082E-05 ), #123803, 'distance_accuracy_value', 'NONE');
#11564=CARTESIAN_POINT ( 'NONE',  ( 18.35373647476854941, -5.808823158059035485, -5.808823158059033709 ) ) ;
#11584=( NAMED_UNIT ( * ) PLANE_ANGLE_UNIT ( ) SI_UNIT ( $, .RADIAN. ) );
#11689=EDGE_CURVE ( 'NONE', #19565, #14349, #2062, .T. ) ;
#11690=CARTESIAN_POINT ( 'NONE',  ( 24.85873647476855908, 5.808823158059031044, -5.808823158059038150 ) ) ;
#11702=ADVANCED_FACE ( 'NONE', ( #48008 ), #26238, .T. ) ;
#11715=CIRCLE ( 'NONE', #78936, 2.552699999999990865 ) ;
#11765=CARTESIAN_POINT ( 'NONE',  ( 1.666965064704732269, -1.287028696899377367E-11, -6.428034935295263708 ) ) ;
#11768=CARTESIAN_POINT ( 'NONE',  ( 0.3485740145173168991, 5.832717272428934230, -5.114375124908068670 ) ) ;
#11777=ORIENTED_EDGE ( 'NONE', *, *, #34197, .T. ) ;
#11790=FACE_OUTER_BOUND ( 'NONE', #97705, .T. ) ;
#11836=DIRECTION ( 'NONE',  ( 1.000000000000000000, 0.000000000000000000, 0.000000000000000000 ) ) ;
#11860=( GEOMETRIC_REPRESENTATION_CONTEXT ( 3 ) GLOBAL_UNCERTAINTY_ASSIGNED_CONTEXT ( ( #111437 ) ) GLOBAL_UNIT_ASSIGNED_CONTEXT ( ( #91839, #68693, #48348 ) ) REPRESENTATION_CONTEXT ( 'NONE', 'WORKASPACE' ) );
#11873=STYLED_ITEM ( 'NONE', ( #91727 ), #41693 ) ;
#11874=CARTESIAN_POINT ( 'NONE',  ( 29.79580628287044419, -5.278424836066144543, 3.047499999999995879 ) ) ;
#11893=ORIENTED_EDGE ( 'NONE', *, *, #91461, .T. ) ;
#11905=CARTESIAN_POINT ( 'NONE',  ( 152.4000000000000057, 0.000000000000000000, -33.92499999999998295 ) ) ;
#11916=VERTEX_POINT ( 'NONE', #52259 ) ;
#11929=CARTESIAN_POINT ( 'NONE',  ( 2.999999999999999112, 1.194621026894847171, -17.40906030209848510 ) ) ;
#11930=FILL_AREA_STYLE_COLOUR ( '', #74211 ) ;
#11940=TOROIDAL_SURFACE ( 'NONE', #92986, 4.000000000000000000, 1.000000000000000000 ) ;
#11943=DIRECTION ( 'NONE',  ( 1.000000000000000000, 0.000000000000000000, 0.000000000000000000 ) ) ;
#11982=CARTESIAN_POINT ( 'NONE',  ( 16.96247294953710849, -7.464222240803106570E-16, -6.094999999999989981 ) ) ;
#12040=AXIS2_PLACEMENT_3D ( 'NONE', #54086, #85228, #139664 ) ;
#12053=CARTESIAN_POINT ( 'NONE',  ( 10.83747294953710671, 6.094999999999989981, -1.119633336120465690E-15 ) ) ;
#12073=FACE_OUTER_BOUND ( 'NONE', #15808, .T. ) ;
#12083=CARTESIAN_POINT ( 'NONE',  ( 10.77040314143521904, -7.934999999999989839, 2.126176841940957907 ) ) ;
#12091=FACE_OUTER_BOUND ( 'NONE', #107319, .T. ) ;
#12128=CARTESIAN_POINT ( 'NONE',  ( 13.12500000000000178, 6.094999999999989981, -1.119633336120465690E-15 ) ) ;
#12129=CARTESIAN_POINT ( 'NONE',  ( 24.62456980810188867, -6.871911579029512218, 3.967499999999996252 ) ) ;
#12138=( GEOMETRIC_REPRESENTATION_CONTEXT ( 3 ) GLOBAL_UNCERTAINTY_ASSIGNED_CONTEXT ( ( #139282 ) ) GLOBAL_UNIT_ASSIGNED_CONTEXT ( ( #60207, #4299, #14543 ) ) REPRESENTATION_CONTEXT ( 'NONE', 'WORKASPACE' ) );
#12149=ORIENTED_EDGE ( 'NONE', *, *, #36653, .F. ) ;
#12151=FILL_AREA_STYLE ('',( #34634 ) ) ;
#12162=CARTESIAN_POINT ( 'NONE',  ( 156.1500000000000057, -49.14999999999999147, -45.92499999999969162 ) ) ;
#12172=LINE ( 'NONE', #57158, #84826 ) ;
#12174=CARTESIAN_POINT ( 'NONE',  ( 184.0791405606631201, -51.15040958483977818, 36.98623100868706359 ) ) ;
#12181=CIRCLE ( 'NONE', #90864, 1.000000000000000888 ) ;
#12189=( LENGTH_UNIT ( ) NAMED_UNIT ( * ) SI_UNIT ( .MILLI., .METRE. ) );
#12190=CARTESIAN_POINT ( 'NONE',  ( 20.92123647476855197, -9.717572351234235426E-16, -7.934999999999990727 ) ) ;
#12192=CARTESIAN_POINT ( 'NONE',  ( 164.2063197296438943, 26.96999999999993847, 34.37654022073930804 ) ) ;
#12196=ADVANCED_FACE ( 'NONE', ( #71723, #49272, #113780 ), #94855, .F. ) ;
#12210=PRESENTATION_STYLE_ASSIGNMENT (( #55751 ) ) ;
#12214=FILL_AREA_STYLE_COLOUR ( '', #72423 ) ;
#12259=AXIS2_PLACEMENT_3D ( 'NONE', #71892, #104476, #35707 ) ;
#12260=CARTESIAN_POINT ( 'NONE',  ( 19.60873647476855197, -5.808823158059033709, 5.808823158059035485 ) ) ;
#12277=( LENGTH_UNIT ( ) NAMED_UNIT ( * ) SI_UNIT ( .MILLI., .METRE. ) );
#12304=CARTESIAN_POINT ( 'NONE',  ( 22.43706980810188867, 2.126176841940952134, -7.934999999999993392 ) ) ;
#12332=CARTESIAN_POINT ( 'NONE',  ( 23.33333333333333570, 5.278424836066143655, -3.047499999999997655 ) ) ;
#12361=CARTESIAN_POINT ( 'NONE',  ( 1.525403141435219379, 2.126176841940962348, 7.934999999999988951 ) ) ;
#12366=ORIENTED_EDGE ( 'NONE', *, *, #97459, .T. ) ;
#12389=CARTESIAN_POINT ( 'NONE',  ( 24.98330628287044419, 6.094999999999991758, 1.633150327867686880 ) ) ;
#12394=VECTOR ( 'NONE', #64123, 1000.000000000000000 ) ;
#12410=ORIENTED_EDGE ( 'NONE', *, *, #45473, .T. ) ;
#12423=MECHANICAL_DESIGN_GEOMETRIC_PRESENTATION_REPRESENTATION('',(#9840),#142126);
#12427=CARTESIAN_POINT ( 'NONE',  ( 28.50456980810189123, 6.871911579029510442, -3.967499999999998916 ) ) ;
#12428=FILL_AREA_STYLE_COLOUR ( '', #9059 ) ;
#12439=ORIENTED_EDGE ( 'NONE', *, *, #123410, .F. ) ;
#12442=CARTESIAN_POINT ( 'NONE',  ( 128.0531643868628464, -51.20434817233906699, -36.87500513592858198 ) ) ;
#12458=CARTESIAN_POINT ( 'NONE',  ( 27.99999999999996803, -49.14999999999999147, 53.92499999999996874 ) ) ;
#12478=( GEOMETRIC_REPRESENTATION_CONTEXT ( 3 ) GLOBAL_UNCERTAINTY_ASSIGNED_CONTEXT ( ( #89525 ) ) GLOBAL_UNIT_ASSIGNED_CONTEXT ( ( #61011, #103038, #136367 ) ) REPRESENTATION_CONTEXT ( 'NONE', 'WORKASPACE' ) );
#12482=CARTESIAN_POINT ( 'NONE',  ( 0.7519484157939031466, -6.935901868405398574, -2.430364388579535628 ) ) ;
#12525=ORIENTED_EDGE ( 'NONE', *, *, #30202, .F. ) ;
#12601=CARTESIAN_POINT ( 'NONE',  ( 30.81663961620377279, -1.633150327867691987, -6.094999999999989093 ) ) ;
#12612=SURFACE_SIDE_STYLE ('',( #111952 ) ) ;
#12620=SURFACE_SIDE_STYLE ('',( #89473 ) ) ;
#12632=CARTESIAN_POINT ( 'NONE',  ( -0.3129301918981139408, -2.126176841940956130, 7.934999999999991616 ) ) ;
#12659=DIRECTION ( 'NONE',  ( 0.000000000000000000, 0.000000000000000000, -1.000000000000000000 ) ) ;
#12666=CARTESIAN_POINT ( 'NONE',  ( 15.64997294953710671, -4.461849672132299105, 4.461849672132299993 ) ) ;
#12676=DIRECTION ( 'NONE',  ( -1.000000000000000000, -0.000000000000000000, -0.000000000000000000 ) ) ;
#12704=EDGE_CURVE ( 'NONE', #63837, #93434, #114860, .T. ) ;
#12712=ORIENTED_EDGE ( 'NONE', *, *, #86051, .T. ) ;
#12742=CARTESIAN_POINT ( 'NONE',  ( 55.56056557994604361, -52.00875322212549179, -39.86617647058817937 ) ) ;
#12754=ORIENTED_EDGE ( 'NONE', *, *, #129002, .F. ) ;
#12761=CARTESIAN_POINT ( 'NONE',  ( 10.39997294953710671, 4.461849672132297329, -4.461849672132302658 ) ) ;
#12766=ADVANCED_FACE ( 'NONE', ( #138947 ), #1447, .T. ) ;
#12771=SURFACE_STYLE_USAGE ( .BOTH. , #69330 ) ;
#12780=( LENGTH_UNIT ( ) NAMED_UNIT ( * ) SI_UNIT ( .MILLI., .METRE. ) );
#12791=CARTESIAN_POINT ( 'NONE',  ( 20.68706980810189222, -2.126176841940956130, 7.934999999999991616 ) ) ;
#12821=FILL_AREA_STYLE ('',( #133220 ) ) ;
#12832=DIRECTION ( 'NONE',  ( 0.000000000000000000, 0.000000000000000000, -1.000000000000000000 ) ) ;
#12835=CARTESIAN_POINT ( 'NONE',  ( 12.68750000000000178, 4.461849672132297329, -4.461849672132302658 ) ) ;
#12848=CARTESIAN_POINT ( 'NONE',  ( 125.3761450143287846, -47.18881911353553704, -35.55177538329112963 ) ) ;
#12868=( BOUNDED_CURVE ( )  B_SPLINE_CURVE ( 2, ( #126933, #38522, #39247, #4386, #116065, #48687, #83460, #6545, #51551, #107333, #87733, #74007, #141393 ),
 .UNSPECIFIED., .F., .T. ) 
 B_SPLINE_CURVE_WITH_KNOTS ( ( 3, 2, 2, 2, 2, 2, 3 ),
 ( 0.05711758424084519004, 0.05833333333333333426, 0.06666666666666666574, 0.07500000000000001110, 0.08333333333333334259, 0.09166666666666667407, 0.1000000000000000333 ),
 .UNSPECIFIED. ) 
 CURVE ( )  GEOMETRIC_REPRESENTATION_ITEM ( )  RATIONAL_B_SPLINE_CURVE ( ( 0.9915083049239661328, 0.9950289225080382050, 1.000000000000000000, 0.9659258262890683122, 1.000000000000000000, 0.9659258262890683122, 1.000000000000000000, 0.9659258262890683122, 1.000000000000000000, 0.9659258262890683122, 1.000000000000000000, 0.9659258262890682012, 1.000000000000000222 ) ) 
 REPRESENTATION_ITEM ( '' )  );
#12917=ORIENTED_EDGE ( 'NONE', *, *, #31591, .T. ) ;
#12950=CARTESIAN_POINT ( 'NONE',  ( 15.06663961620376924, 1.633150327867695095, 6.094999999999988205 ) ) ;
#12961=CARTESIAN_POINT ( 'NONE',  ( 20.92123647476855197, -9.717572351234235426E-16, -7.934999999999990727 ) ) ;
#12984=CARTESIAN_POINT ( 'NONE',  ( 58.54058136200957563, -46.07581969935342414, -35.63601533997326243 ) ) ;
#12993=UNCERTAINTY_MEASURE_WITH_UNIT (LENGTH_MEASURE( 1.000000000000000082E-05 ), #36176, 'distance_accuracy_value', 'NONE');
#13007=CARTESIAN_POINT ( 'NONE',  ( 23.02040314143522082, 7.934999999999989839, -2.126176841940961904 ) ) ;
#13038=ORIENTED_EDGE ( 'NONE', *, *, #80551, .T. ) ;
#13040=EDGE_CURVE ( 'NONE', #56501, #66484, #105750, .T. ) ;
#13062=CARTESIAN_POINT ( 'NONE',  ( 2.837903141435219379, -6.871911579029513106, -3.967499999999993587 ) ) ;
#13068=ORIENTED_EDGE ( 'NONE', *, *, #54836, .T. ) ;
#13075=PRESENTATION_STYLE_ASSIGNMENT (( #32733 ) ) ;
#13081=PRESENTATION_STYLE_ASSIGNMENT (( #100126 ) ) ;
#13084=DIRECTION ( 'NONE',  ( 0.000000000000000000, 0.000000000000000000, -1.000000000000000000 ) ) ;
#13094=CONICAL_SURFACE ( 'NONE', #75638, 8.094999999999991758, 0.7853981633974466137 ) ;
#13110=SURFACE_STYLE_FILL_AREA ( #103004 ) ;
#13119=CARTESIAN_POINT ( 'NONE',  ( 160.4291323974385080, 26.96999999999993847, -34.92499999999998295 ) ) ;
#13124=CARTESIAN_POINT ( 'NONE',  ( 26.02540314143521982, 2.126176841940962348, 7.934999999999989839 ) ) ;
#13140=CARTESIAN_POINT ( 'NONE',  ( 125.7224624600519718, -47.70829528212275505, -34.92499999999998295 ) ) ;
#13148=ORIENTED_EDGE ( 'NONE', *, *, #44883, .F. ) ;
#13163=EDGE_LOOP ( 'NONE', ( #131900, #67205, #120225, #106376, #37906, #53500, #23601, #97238 ) ) ;
#13179=CARTESIAN_POINT ( 'NONE',  ( 1.632902354900489739, -0.3019974585920503496, -6.462097645098976884 ) ) ;
#13193=CARTESIAN_POINT ( 'NONE',  ( 1.074257766332453956, 4.331830624465606405, 5.540583863682179810 ) ) ;
#13210=VECTOR ( 'NONE', #22245, 1000.000000000000000 ) ;
#13233=CIRCLE ( 'NONE', #142817, 3.999999999999996447 ) ;
#13259=DIRECTION ( 'NONE',  ( 0.000000000000000000, -0.000000000000000000, -1.000000000000000000 ) ) ;
#13300=CARTESIAN_POINT ( 'NONE',  ( 3.567069808101885897, 2.126176841940952134, -7.934999999999993392 ) ) ;
#13337=SURFACE_SIDE_STYLE ('',( #34403 ) ) ;
#13347=( NAMED_UNIT ( * ) PLANE_ANGLE_UNIT ( ) SI_UNIT ( $, .RADIAN. ) );
#13350=ADVANCED_FACE ( 'NONE', ( #94881 ), #118298, .T. ) ;
#13359=( LENGTH_UNIT ( ) NAMED_UNIT ( * ) SI_UNIT ( .MILLI., .METRE. ) );
#13460=CARTESIAN_POINT ( 'NONE',  ( 8.066639616203771013, 1.633150327867695095, 6.094999999999988205 ) ) ;
#13495=CARTESIAN_POINT ( 'NONE',  ( 18.20790314143522082, -6.871911579029513106, -3.967499999999993587 ) ) ;
#13542=CARTESIAN_POINT ( 'NONE',  ( 17.06250000000000000, 4.461849672132300881, 4.461849672132299105 ) ) ;
#13543=CARTESIAN_POINT ( 'NONE',  ( 23.16623647476855652, 7.934999999999990727, -1.457635852685135314E-15 ) ) ;
#13548=CIRCLE ( 'NONE', #69165, 3.999999999999989786 ) ;
#13600=CARTESIAN_POINT ( 'NONE',  ( 23.40040314143521982, -7.934999999999988951, 2.126176841940957907 ) ) ;
#13604=SURFACE_SIDE_STYLE ('',( #91225 ) ) ;
#13643=CARTESIAN_POINT ( 'NONE',  ( 20.46247294953710849, -7.464222240803106570E-16, -6.094999999999989981 ) ) ;
#13664=CARTESIAN_POINT ( 'NONE',  ( 33.02540314143521272, 2.126176841940962348, 7.934999999999989839 ) ) ;
#13671=EDGE_CURVE ( 'NONE', #59338, #96891, #133028, .T. ) ;
#13686=AXIS2_PLACEMENT_3D ( 'NONE', #24693, #89249, #68254 ) ;
#13690=CIRCLE ( 'NONE', #110959, 1.000000000000000888 ) ;
#13691=ADVANCED_FACE ( 'NONE', ( #91634 ), #102533, .F. ) ;
#13709=CARTESIAN_POINT ( 'NONE',  ( 22.87456980810188867, 6.871911579029510442, -3.967499999999998916 ) ) ;
#13710=CARTESIAN_POINT ( 'NONE',  ( 0.8537364747685527444, -5.808823158059035485, -5.808823158059033709 ) ) ;
#13711=STYLED_ITEM ( 'NONE', ( #77425 ), #47657 ) ;
#13727=VECTOR ( 'NONE', #51617, 1000.000000000000000 ) ;
#13744=CARTESIAN_POINT ( 'NONE',  ( 53.19685992802467212, -48.66302742222553945, 38.53170190052308186 ) ) ;
#13751=COLOUR_RGB ( '', 0.09019608, 0.27058824, 0.51372549) ;
#13820=CIRCLE ( 'NONE', #124995, 2.999999999999999556 ) ;
#13824=COLOUR_RGB ( '', 0.40784314, 0.44705882, 0.49803922) ;
#13835=CARTESIAN_POINT ( 'NONE',  ( 29.08790314143522338, 6.871911579029515771, 3.967499999999989146 ) ) ;
#13837=CARTESIAN_POINT ( 'NONE',  ( 2.546236474768552860, -7.934999999999990727, 4.858786175617117713E-16 ) ) ;
#13842=DIRECTION ( 'NONE',  ( 0.000000000000000000, 0.06845965770171351383, 0.9976538855070752332 ) ) ;
#13843=FACE_OUTER_BOUND ( 'NONE', #118527, .T. ) ;
#13869=STYLED_ITEM ( 'NONE', ( #112173 ), #75511 ) ;
#13870=ORIENTED_EDGE ( 'NONE', *, *, #16097, .F. ) ;
#13873=CYLINDRICAL_SURFACE ( 'NONE', #1082, 3.000000000000000000 ) ;
#13877=FILL_AREA_STYLE_COLOUR ( '', #16934 ) ;
#13933=CIRCLE ( 'NONE', #83745, 25.00000000000002842 ) ;
#13950=AXIS2_PLACEMENT_3D ( 'NONE', #115577, #138824, #113469 ) ;
#13960=ORIENTED_EDGE ( 'NONE', *, *, #124570, .F. ) ;
#13971=CARTESIAN_POINT ( 'NONE',  ( 25.39999999999999858, -5.520864266206504263E-14, -33.92499999999998295 ) ) ;
#13975=ORIENTED_EDGE ( 'NONE', *, *, #39040, .F. ) ;
#13976=( GEOMETRIC_REPRESENTATION_CONTEXT ( 3 ) GLOBAL_UNCERTAINTY_ASSIGNED_CONTEXT ( ( #49068 ) ) GLOBAL_UNIT_ASSIGNED_CONTEXT ( ( #46955, #124457, #1221 ) ) REPRESENTATION_CONTEXT ( 'NONE', 'WORKASPACE' ) );
#13984=EDGE_CURVE ( 'NONE', #25649, #94899, #56338, .T. ) ;
#14013=( NAMED_UNIT ( * ) PLANE_ANGLE_UNIT ( ) SI_UNIT ( $, .RADIAN. ) );
#14015=CARTESIAN_POINT ( 'NONE',  ( 0.2129031414352194063, 3.967499999999992699, -6.871911579029513994 ) ) ;
#14038=CARTESIAN_POINT ( 'NONE',  ( 25.39999999999999858, 0.000000000000000000, 0.000000000000000000 ) ) ;
#14044=DIRECTION ( 'NONE',  ( -0.2399999999999971323, 0.000000000000000000, 0.9707728879609286432 ) ) ;
#14063=EDGE_LOOP ( 'NONE', ( #117598, #86310, #38216, #128693 ) ) ;
#14065=STYLED_ITEM ( 'NONE', ( #139314 ), #22381 ) ;
#14070=CARTESIAN_POINT ( 'NONE',  ( 183.7627343495646812, -51.96230815476841514, -39.57541490114648042 ) ) ;
#14071=FILL_AREA_STYLE_COLOUR ( '', #90457 ) ;
#14075=STYLED_ITEM ( 'NONE', ( #104240 ), #27794 ) ;
#14086=UNCERTAINTY_MEASURE_WITH_UNIT (LENGTH_MEASURE( 1.000000000000000082E-05 ), #43043, 'distance_accuracy_value', 'NONE');
#14111=VERTEX_POINT ( 'NONE', #17007 ) ;
#14138=EDGE_LOOP ( 'NONE', ( #106849, #67321, #26184, #48568 ) ) ;
#14148=CARTESIAN_POINT ( 'NONE',  ( 181.1500000000000057, -3.180000000000061444, 34.92499999999998295 ) ) ;
#14162=SURFACE_STYLE_USAGE ( .BOTH. , #83009 ) ;
#14197=CARTESIAN_POINT ( 'NONE',  ( 3.254139616203772345, 3.047499999999993214, -5.278424836066146320 ) ) ;
#14208=DIRECTION ( 'NONE',  ( -1.000000000000000000, -0.000000000000000000, -0.000000000000000000 ) ) ;
#14223=MECHANICAL_DESIGN_GEOMETRIC_PRESENTATION_REPRESENTATION('',(#35064),#92984);
#14227=DIRECTION ( 'NONE',  ( 0.000000000000000000, 0.000000000000000000, 1.000000000000000000 ) ) ;
#14235=CARTESIAN_POINT ( 'NONE',  ( 26.37456980810188867, 6.871911579029510442, -3.967499999999998916 ) ) ;
#14244=SURFACE_STYLE_FILL_AREA ( #1889 ) ;
#14246=UNCERTAINTY_MEASURE_WITH_UNIT (LENGTH_MEASURE( 1.000000000000000082E-05 ), #5974, 'distance_accuracy_value', 'NONE');
#14255=CARTESIAN_POINT ( 'NONE',  ( 128.9683591370937563, -52.14999999999999147, 41.64499999999997470 ) ) ;
#14276=DIRECTION ( 'NONE',  ( -0.000000000000000000, -0.000000000000000000, -1.000000000000000000 ) ) ;
#14281=CARTESIAN_POINT ( 'NONE',  ( 24.79166666666667140, -3.047499999999994547, 5.278424836066145431 ) ) ;
#14283=CARTESIAN_POINT ( 'NONE',  ( 23.89540314143522437, 2.126176841940962348, 7.934999999999988951 ) ) ;
#14329=EDGE_CURVE ( 'NONE', #117767, #60012, #39501, .T. ) ;
#14333=( GEOMETRIC_REPRESENTATION_CONTEXT ( 3 ) GLOBAL_UNCERTAINTY_ASSIGNED_CONTEXT ( ( #86851 ) ) GLOBAL_UNIT_ASSIGNED_CONTEXT ( ( #47663, #91824, #4047 ) ) REPRESENTATION_CONTEXT ( 'NONE', 'WORKASPACE' ) );
#14349=VERTEX_POINT ( 'NONE', #21988 ) ;
#14413=CARTESIAN_POINT ( 'NONE',  ( 23.83790314143521982, -6.871911579029513106, -3.967499999999993587 ) ) ;
#14438=VECTOR ( 'NONE', #119134, 1000.000000000000000 ) ;
#14449=UNCERTAINTY_MEASURE_WITH_UNIT (LENGTH_MEASURE( 1.000000000000000082E-05 ), #74958, 'distance_accuracy_value', 'NONE');
#14457=CARTESIAN_POINT ( 'NONE',  ( 23.89540314143522437, 2.126176841940962348, 7.934999999999989839 ) ) ;
#14488=ORIENTED_EDGE ( 'NONE', *, *, #108616, .T. ) ;
#14511=SURFACE_STYLE_USAGE ( .BOTH. , #111692 ) ;
#14543=( NAMED_UNIT ( * ) SI_UNIT ( $, .STERADIAN. ) SOLID_ANGLE_UNIT ( ) );
#14546=ORIENTED_EDGE ( 'NONE', *, *, #69663, .F. ) ;
#14554=FILL_AREA_STYLE_COLOUR ( '', #25197 ) ;
#14561=DIRECTION ( 'NONE',  ( 0.000000000000000000, 0.000000000000000000, 1.000000000000000000 ) ) ;
#14581=CARTESIAN_POINT ( 'NONE',  ( 1.671236474768553082, 0.000000000000000000, 7.934999999999990727 ) ) ;
#14598=CARTESIAN_POINT ( 'NONE',  ( 180.8090197240767054, -49.02095135882321131, -39.67421197283155720 ) ) ;
#14606=CIRCLE ( 'NONE', #135099, 2.999999999999992450 ) ;
#14645=STYLED_ITEM ( 'NONE', ( #103010 ), #43643 ) ;
#14662=PRESENTATION_STYLE_ASSIGNMENT (( #93659 ) ) ;
#14700=EDGE_LOOP ( 'NONE', ( #106079, #50304, #90858, #136400, #35050, #11010 ) ) ;
#14705=ORIENTED_EDGE ( 'NONE', *, *, #45745, .T. ) ;
#14752=CARTESIAN_POINT ( 'NONE',  ( 3.712903141435219379, 3.967499999999992699, -6.871911579029513994 ) ) ;
#14754=ORIENTED_EDGE ( 'NONE', *, *, #85006, .T. ) ;
#14765=DIRECTION ( 'NONE',  ( 0.000000000000000000, -1.000000000000000000, 0.000000000000000000 ) ) ;
#14778=FILL_AREA_STYLE ('',( #5306 ) ) ;
#14786=CARTESIAN_POINT ( 'NONE',  ( 8.728736474768551190, 5.808823158059031044, -5.808823158059038150 ) ) ;
#14804=CARTESIAN_POINT ( 'NONE',  ( 151.4000000000000057, -18.48000000000005372, -33.92499999999998295 ) ) ;
#14810=( NAMED_UNIT ( * ) SI_UNIT ( $, .STERADIAN. ) SOLID_ANGLE_UNIT ( ) );
#14844=CARTESIAN_POINT ( 'NONE',  ( 3.000000000000000000, -49.85820393249939286, 34.92500000000001847 ) ) ;
#14868=( BOUNDED_CURVE ( )  B_SPLINE_CURVE ( 2, ( #140160, #18322, #62596, #87192, #28545, #96593, #31388, #86492, #106782, #140833, #85748, #53111, #97311 ),
 .UNSPECIFIED., .F., .T. ) 
 B_SPLINE_CURVE_WITH_KNOTS ( ( 3, 2, 2, 2, 2, 2, 3 ),
 ( 0.2000000000000000666, 0.2083333333333333981, 0.2166666666666667018, 0.2250000000000000333, 0.2333333333333333648, 0.2416666666666666963, 0.2500000000000000000 ),
 .UNSPECIFIED. ) 
 CURVE ( )  GEOMETRIC_REPRESENTATION_ITEM ( )  RATIONAL_B_SPLINE_CURVE ( ( 0.9999999999999997780, 0.9659258262890685343, 1.000000000000000000, 0.9659258262890683122, 1.000000000000000000, 0.9659258262890683122, 1.000000000000000000, 0.9659258262890683122, 1.000000000000000000, 0.9659258262890683122, 1.000000000000000000, 0.9659258262890683122, 1.000000000000000000 ) ) 
 REPRESENTATION_ITEM ( '' )  );
#14870=EDGE_CURVE ( 'NONE', #37393, #36041, #2862, .T. ) ;
#14882=ORIENTED_EDGE ( 'NONE', *, *, #38940, .F. ) ;
#14894=CARTESIAN_POINT ( 'NONE',  ( 25.40000000000000213, 7.917808315101192207, 0.6621923558222658768 ) ) ;
#14909=CARTESIAN_POINT ( 'NONE',  ( 5.149972949537104938, -4.461849672132299105, 4.461849672132299993 ) ) ;
#14927=ORIENTED_EDGE ( 'NONE', *, *, #36879, .T. ) ;
#14928=SURFACE_STYLE_USAGE ( .BOTH. , #70089 ) ;
#14937=CARTESIAN_POINT ( 'NONE',  ( 18.64540314143522437, -2.126176841940958351, -7.934999999999989839 ) ) ;
#14965=DIRECTION ( 'NONE',  ( 0.000000000000000000, 0.06845965770171351383, 0.9976538855070752332 ) ) ;
#14985=CARTESIAN_POINT ( 'NONE',  ( 26.68750000000000355, 4.461849672132297329, -4.461849672132302658 ) ) ;
#15008=CARTESIAN_POINT ( 'NONE',  ( 24.39999999999999858, 1.194621026894846283, 17.40906030209848510 ) ) ;
#15015=EDGE_LOOP ( 'NONE', ( #139587, #61648, #88616, #27870 ) ) ;
#15029=LINE ( 'NONE', #72334, #1494 ) ;
#15039=CYLINDRICAL_SURFACE ( 'NONE', #73555, 34.93000000000001393 ) ;
#15068=ORIENTED_EDGE ( 'NONE', *, *, #68907, .F. ) ;
#15083=SURFACE_STYLE_FILL_AREA ( #105652 ) ;
#15098=ORIENTED_EDGE ( 'NONE', *, *, #96479, .T. ) ;
#15100=CARTESIAN_POINT ( 'NONE',  ( 29.23373647476855552, 5.808823158059036373, 5.808823158059032821 ) ) ;
#15118=VERTEX_POINT ( 'NONE', #99745 ) ;
#15120=( NAMED_UNIT ( * ) PLANE_ANGLE_UNIT ( ) SI_UNIT ( $, .RADIAN. ) );
#15129=DIRECTION ( 'NONE',  ( -1.000000000000000000, -0.000000000000000000, 0.000000000000000000 ) ) ;
#15131=EDGE_CURVE ( 'NONE', #42602, #62992, #412, .T. ) ;
#15144=CARTESIAN_POINT ( 'NONE',  ( 26.81206980810188512, 7.934999999999993392, 2.126176841940951689 ) ) ;
#15158=CARTESIAN_POINT ( 'NONE',  ( 23.23330628287043709, -6.094999999999989981, -1.633150327867689322 ) ) ;
#15175=FACE_OUTER_BOUND ( 'NONE', #39786, .T. ) ;
#15193=ORIENTED_EDGE ( 'NONE', *, *, #54951, .T. ) ;
#15201=CARTESIAN_POINT ( 'NONE',  ( 2.983736474768552860, -5.808823158059035485, -5.808823158059033709 ) ) ;
#15202=SURFACE_SIDE_STYLE ('',( #115940 ) ) ;
#15213=CARTESIAN_POINT ( 'NONE',  ( 151.4000000000000057, -16.48000000000005016, 0.000000000000000000 ) ) ;
#15237=FACE_OUTER_BOUND ( 'NONE', #7983, .T. ) ;
#15271=SURFACE_STYLE_FILL_AREA ( #49406 ) ;
#15301=DIRECTION ( 'NONE',  ( -0.9707728879609287542, 0.000000000000000000, -0.2399999999999954392 ) ) ;
#15304=ADVANCED_FACE ( 'NONE', ( #81595 ), #128644, .F. ) ;
#15335=CARTESIAN_POINT ( 'NONE',  ( 24.39999999999999858, -2.599999999999908606, 1.319531433729349815E-14 ) ) ;
#15349=MECHANICAL_DESIGN_GEOMETRIC_PRESENTATION_REPRESENTATION('',(#1477),#121836);
#15364=AXIS2_PLACEMENT_3D ( 'NONE', #74979, #61954, #51786 ) ;
#15377=CARTESIAN_POINT ( 'NONE',  ( 28.00000000000002487, -57.14999999999999147, 34.92500000000003268 ) ) ;
#15399=CARTESIAN_POINT ( 'NONE',  ( 58.42753753994784205, -47.70829528212276927, -34.92499999999998295 ) ) ;
#15415=ORIENTED_EDGE ( 'NONE', *, *, #135373, .F. ) ;
#15424=CARTESIAN_POINT ( 'NONE',  ( 9.837903141435219823, -6.871911579029513106, -3.967499999999993587 ) ) ;
#15447=CARTESIAN_POINT ( 'NONE',  ( 6.899972949537105826, 4.461849672132297329, -4.461849672132302658 ) ) ;
#15455=CIRCLE ( 'NONE', #17743, 3.999999999999996447 ) ;
#15458=CARTESIAN_POINT ( 'NONE',  ( 9.166236474768552966, 7.934999999999990727, -1.457635852685135314E-15 ) ) ;
#15465=EDGE_CURVE ( 'NONE', #60580, #126231, #31479, .T. ) ;
#15477=CYLINDRICAL_SURFACE ( 'NONE', #169, 28.00000000000002487 ) ;
#15481=ORIENTED_EDGE ( 'NONE', *, *, #78375, .F. ) ;
#15515=SURFACE_STYLE_FILL_AREA ( #137353 ) ;
#15519=CARTESIAN_POINT ( 'NONE',  ( 0.000000000000000000, -43.14999999999999147, -34.92499999999998295 ) ) ;
#15526=DIRECTION ( 'NONE',  ( 0.000000000000000000, 0.000000000000000000, 1.000000000000000000 ) ) ;
#15539=ORIENTED_EDGE ( 'NONE', *, *, #14870, .F. ) ;
#15585=CARTESIAN_POINT ( 'NONE',  ( 13.60830628287044064, 1.633150327867687324, -6.094999999999991758 ) ) ;
#15596=EDGE_CURVE ( 'NONE', #57246, #141239, #22692, .T. ) ;
#15602=PRODUCT_DEFINITION_SHAPE ( 'NONE', 'NONE',  #37749 ) ;
#15613=CARTESIAN_POINT ( 'NONE',  ( 24.77040314143521726, -7.934999999999989839, 2.126176841940957907 ) ) ;
#15645=EDGE_CURVE ( 'NONE', #59338, #18319, #79265, .T. ) ;
#15665=CARTESIAN_POINT ( 'NONE',  ( 27.12500000000000355, 6.094999999999989981, -1.119633336120465690E-15 ) ) ;
#15725=( NAMED_UNIT ( * ) PLANE_ANGLE_UNIT ( ) SI_UNIT ( $, .RADIAN. ) );
#15726=ORIENTED_EDGE ( 'NONE', *, *, #74130, .T. ) ;
#15743=VERTEX_POINT ( 'NONE', #16861 ) ;
#15754=LINE ( 'NONE', #36155, #44444 ) ;
#15760=FILL_AREA_STYLE_COLOUR ( '', #46776 ) ;
#15780=CARTESIAN_POINT ( 'NONE',  ( 27.92123647476855197, -9.717572351234235426E-16, -7.934999999999990727 ) ) ;
#15785=EDGE_CURVE ( 'NONE', #29858, #46809, #120156, .T. ) ;
#15808=EDGE_LOOP ( 'NONE', ( #114681, #70304, #38984, #25529, #1229, #14754 ) ) ;
#15817=UNCERTAINTY_MEASURE_WITH_UNIT (LENGTH_MEASURE( 1.000000000000000082E-05 ), #94570, 'distance_accuracy_value', 'NONE');
#15828=CARTESIAN_POINT ( 'NONE',  ( 29.72873647476855297, 5.808823158059031044, -5.808823158059038150 ) ) ;
#15829=CARTESIAN_POINT ( 'NONE',  ( 7.270403141435218153, -7.934999999999988951, 2.126176841940957907 ) ) ;
#15844=AXIS2_PLACEMENT_3D ( 'NONE', #9947, #21555, #65816 ) ;
#15861=CARTESIAN_POINT ( 'NONE',  ( 52.60764783923757903, -49.05583548141700589, 39.86617647058822200 ) ) ;
#15868=FILL_AREA_STYLE_COLOUR ( '', #87268 ) ;
#15891=CARTESIAN_POINT ( 'NONE',  ( 8.525403141435219823, 2.126176841940962348, 7.934999999999988951 ) ) ;
#15895=SURFACE_STYLE_USAGE ( .BOTH. , #15202 ) ;
#15907=CARTESIAN_POINT ( 'NONE',  ( 5.250000000000000000, -7.464222240803106570E-16, -6.094999999999989981 ) ) ;
#15917=SURFACE_STYLE_USAGE ( .BOTH. , #136311 ) ;
#15944=FACE_OUTER_BOUND ( 'NONE', #25192, .T. ) ;
#15962=CARTESIAN_POINT ( 'NONE',  ( 3.712903141435219379, 3.967499999999992699, -6.871911579029513994 ) ) ;
#15987=ORIENTED_EDGE ( 'NONE', *, *, #121896, .F. ) ;
#15989=MECHANICAL_DESIGN_GEOMETRIC_PRESENTATION_REPRESENTATION('',(#80836),#78548);
#16000=SURFACE_STYLE_FILL_AREA ( #115302 ) ;
#16041=SURFACE_SIDE_STYLE ('',( #36418 ) ) ;
#16051=PRESENTATION_STYLE_ASSIGNMENT (( #26967 ) ) ;
#16086=PRESENTATION_STYLE_ASSIGNMENT (( #47392 ) ) ;
#16097=EDGE_CURVE ( 'NONE', #62156, #42914, #72545, .T. ) ;
#16103=VERTEX_POINT ( 'NONE', #5048 ) ;
#16114=ADVANCED_FACE ( 'NONE', ( #137766 ), #116707, .F. ) ;
#16117=VECTOR ( 'NONE', #101448, 1000.000000000000000 ) ;
#16140=CARTESIAN_POINT ( 'NONE',  ( 7.358736474768553748, 5.808823158059031044, -5.808823158059038150 ) ) ;
#16162=VECTOR ( 'NONE', #67200, 1000.000000000000000 ) ;
#16163=AXIS2_PLACEMENT_3D ( 'NONE', #6514, #95715, #51522 ) ;
#16177=CARTESIAN_POINT ( 'NONE',  ( 4.499569808101886892, -3.967499999999998028, -6.871911579029511330 ) ) ;
#16203=SURFACE_STYLE_USAGE ( .BOTH. , #39446 ) ;
#16263=MECHANICAL_DESIGN_GEOMETRIC_PRESENTATION_REPRESENTATION('',(#69517),#25498);
#16301=CARTESIAN_POINT ( 'NONE',  ( 181.0474453055293793, -48.63825160239813528, -38.47250499286692360 ) ) ;
#16317=CARTESIAN_POINT ( 'NONE',  ( 14.48330628287044064, 6.094999999999991758, 1.633150327867687102 ) ) ;
#16334=ADVANCED_FACE ( 'NONE', ( #54344 ), #37726, .T. ) ;
#16346=CARTESIAN_POINT ( 'NONE',  ( 30.89540314143522437, 2.126176841940962348, 7.934999999999989839 ) ) ;
#16370=COLOUR_RGB ( '', 0.31764706, 0.68627451, 0.89019608) ;
#16381=DIRECTION ( 'NONE',  ( 0.000000000000000000, -1.000000000000000000, 0.000000000000000000 ) ) ;
#16387=ORIENTED_EDGE ( 'NONE', *, *, #133719, .F. ) ;
#16395=CARTESIAN_POINT ( 'NONE',  ( 22.31249999999999645, -4.461849672132299993, -4.461849672132299105 ) ) ;
#16415=AXIS2_PLACEMENT_3D ( 'NONE', #130721, #65468, #31385 ) ;
#16422=( NAMED_UNIT ( * ) PLANE_ANGLE_UNIT ( ) SI_UNIT ( $, .RADIAN. ) );
#16449=CARTESIAN_POINT ( 'NONE',  ( 25.40000000000000568, -6.022532542321925142, -4.245577695859290124 ) ) ;
#16450=PRESENTATION_STYLE_ASSIGNMENT (( #83175 ) ) ;
#16468=DIRECTION ( 'NONE',  ( 0.000000000000000000, 0.000000000000000000, 1.000000000000000000 ) ) ;
#16490=AXIS2_PLACEMENT_3D ( 'NONE', #46821, #1090, #132384 ) ;
#16528=CARTESIAN_POINT ( 'NONE',  ( 24.56706980810189123, 2.126176841940952134, -7.934999999999993392 ) ) ;
#16540=FILL_AREA_STYLE ('',( #138348 ) ) ;
#16573=CARTESIAN_POINT ( 'NONE',  ( 5.421010862427522170E-17, 0.000000000000000000, 6.094999999999989981 ) ) ;
#16574=CARTESIAN_POINT ( 'NONE',  ( 5.228736474768553855, 5.808823158059031044, -5.808823158059037262 ) ) ;
#16577=CIRCLE ( 'NONE', #97606, 4.000000000000000000 ) ;
#16617=( LENGTH_UNIT ( ) NAMED_UNIT ( * ) SI_UNIT ( .MILLI., .METRE. ) );
#16639=CARTESIAN_POINT ( 'NONE',  ( 10.56706980810188767, 2.126176841940952134, -7.934999999999992504 ) ) ;
#16645=PRESENTATION_STYLE_ASSIGNMENT (( #15895 ) ) ;
#16718=CARTESIAN_POINT ( 'NONE',  ( 32.58790314143522693, 6.871911579029515771, 3.967499999999989146 ) ) ;
#16722=SURFACE_STYLE_FILL_AREA ( #39201 ) ;
#16733=CARTESIAN_POINT ( 'NONE',  ( 183.6085471140778225, -52.10163751122234288, -40.43817685073710066 ) ) ;
#16741=DIRECTION ( 'NONE',  ( -1.000000000000000000, -0.000000000000000000, -0.000000000000000000 ) ) ;
#16761=LINE ( 'NONE', #137123, #83759 ) ;
#16833=EDGE_CURVE ( 'NONE', #108472, #104144, #137812, .T. ) ;
#16861=CARTESIAN_POINT ( 'NONE',  ( 2.000000000000256239, -6.019044215166783118, 0.9592349742722835471 ) ) ;
#16864=PRESENTATION_STYLE_ASSIGNMENT (( #103147 ) ) ;
#16893=CARTESIAN_POINT ( 'NONE',  ( 2.999999999999999112, -7.600000000000061817, 34.92499999999998295 ) ) ;
#16900=CARTESIAN_POINT ( 'NONE',  ( 11.29623647476855375, 7.934999999999990727, -1.457635852685135314E-15 ) ) ;
#16932=CARTESIAN_POINT ( 'NONE',  ( 5.666236474768552966, 7.934999999999990727, -1.457635852685135314E-15 ) ) ;
#16934=COLOUR_RGB ( '', 0.66274510, 0.83137255, 0.94901961) ;
#16946=CARTESIAN_POINT ( 'NONE',  ( 183.6042742895559172, -52.10338527932237440, -40.45859298138255156 ) ) ;
#16947=ORIENTED_EDGE ( 'NONE', *, *, #91461, .F. ) ;
#16950=CIRCLE ( 'NONE', #35511, 3.999999999999996447 ) ;
#16965=UNCERTAINTY_MEASURE_WITH_UNIT (LENGTH_MEASURE( 1.000000000000000082E-05 ), #43590, 'distance_accuracy_value', 'NONE');
#17000=AXIS2_PLACEMENT_3D ( 'NONE', #14844, #102599, #34471 ) ;
#17007=CARTESIAN_POINT ( 'NONE',  ( 55.56056557994604361, -57.14999999999999147, -39.86617647058817937 ) ) ;
#17035=PRESENTATION_STYLE_ASSIGNMENT (( #14162 ) ) ;
#17070=CARTESIAN_POINT ( 'NONE',  ( 15.79580628287043709, -5.278424836066144543, 3.047499999999995879 ) ) ;
#17090=DIRECTION ( 'NONE',  ( 0.000000000000000000, 1.000000000000000000, -3.469446951953614189E-15 ) ) ;
#17101=CARTESIAN_POINT ( 'NONE',  ( 30.60373647476856007, 5.808823158059036373, 5.808823158059032821 ) ) ;
#17113=CARTESIAN_POINT ( 'NONE',  ( 0.2099742459738602463, -51.66308182546714534, -38.35990878063566356 ) ) ;
#17130=EDGE_CURVE ( 'NONE', #107938, #64706, #124045, .T. ) ;
#17148=CARTESIAN_POINT ( 'NONE',  ( 21.58333333333333570, -5.278424836066144543, 3.047499999999995879 ) ) ;
#17172=CARTESIAN_POINT ( 'NONE',  ( 1.394470636259349527, -0.3801107925066945503, 6.692409305308472334 ) ) ;
#17182=CARTESIAN_POINT ( 'NONE',  ( 184.1500000000000057, -14.29000000000013593, 12.69999999999954632 ) ) ;
#17200=SURFACE_STYLE_USAGE ( .BOTH. , #93331 ) ;
#17211=SURFACE_STYLE_FILL_AREA ( #18607 ) ;
#17213=SURFACE_STYLE_FILL_AREA ( #61475 ) ;
#17221=ORIENTED_EDGE ( 'NONE', *, *, #119476, .T. ) ;
#17258=CARTESIAN_POINT ( 'NONE',  ( 0.1121846519738732423, -51.37040454773215714, 37.49526731631105037 ) ) ;
#17260=CARTESIAN_POINT ( 'NONE',  ( 6.541236474768552966, 0.000000000000000000, 7.934999999999990727 ) ) ;
#17272=( NAMED_UNIT ( * ) PLANE_ANGLE_UNIT ( ) SI_UNIT ( $, .RADIAN. ) );
#17290=UNCERTAINTY_MEASURE_WITH_UNIT (LENGTH_MEASURE( 1.000000000000000082E-05 ), #128184, 'distance_accuracy_value', 'NONE');
#17303=CARTESIAN_POINT ( 'NONE',  ( 0.1458333333333333981, -1.633150327867689988, 6.094999999999989981 ) ) ;
#17304=CARTESIAN_POINT ( 'NONE',  ( 9.312069808101886892, 7.934999999999992504, 2.126176841940951689 ) ) ;
#17327=SURFACE_STYLE_FILL_AREA ( #60890 ) ;
#17331=LINE ( 'NONE', #3574, #123981 ) ;
#17360=CARTESIAN_POINT ( 'NONE',  ( 11.44206980810188767, 7.934999999999992504, 2.126176841940951689 ) ) ;
#17367=MECHANICAL_DESIGN_GEOMETRIC_PRESENTATION_REPRESENTATION('',(#105422),#84560);
#17386=CARTESIAN_POINT ( 'NONE',  ( 25.40000000000000568, -0.2953647482591277851, -7.939948287776192437 ) ) ;
#17426=CARTESIAN_POINT ( 'NONE',  ( 7.358736474768553748, 5.808823158059031044, -5.808823158059038150 ) ) ;
#17429=CARTESIAN_POINT ( 'NONE',  ( 55.18164086290604331, -52.14999999999999147, 41.64499999999997470 ) ) ;
#17431=LINE ( 'NONE', #82710, #62896 ) ;
#17451=CARTESIAN_POINT ( 'NONE',  ( 0.2153679725188837879, -51.67626207039724306, -38.40320453011149482 ) ) ;
#17454=PRESENTATION_STYLE_ASSIGNMENT (( #50821 ) ) ;
#17456=CARTESIAN_POINT ( 'NONE',  ( 25.39999999999999858, -57.15000000000008384, -34.92499999999998295 ) ) ;
#17457=UNCERTAINTY_MEASURE_WITH_UNIT (LENGTH_MEASURE( 1.000000000000000082E-05 ), #68939, 'distance_accuracy_value', 'NONE');
#17497=FACE_BOUND ( 'NONE', #111787, .T. ) ;
#17499=SURFACE_SIDE_STYLE ('',( #84905 ) ) ;
#17549=VERTEX_POINT ( 'NONE', #99981 ) ;
#17577=ORIENTED_EDGE ( 'NONE', *, *, #3843, .T. ) ;
#17584=CARTESIAN_POINT ( 'NONE',  ( 5.462903141435219823, -3.967499999999994476, 6.871911579029513106 ) ) ;
#17590=CARTESIAN_POINT ( 'NONE',  ( 25.40000000000000568, -6.088644610809077484, -0.2782657062331916342 ) ) ;
#17593=AXIS2_PLACEMENT_3D ( 'NONE', #20707, #19295, #119302 ) ;
#17615=CARTESIAN_POINT ( 'NONE',  ( 2.895403141435219485, 2.126176841940962348, 7.934999999999989839 ) ) ;
#17632=LINE ( 'NONE', #95926, #48862 ) ;
#17662=CARTESIAN_POINT ( 'NONE',  ( 25.39999999999999858, 0.000000000000000000, 0.000000000000000000 ) ) ;
#17685=VERTEX_POINT ( 'NONE', #68768 ) ;
#17689=PRESENTATION_STYLE_ASSIGNMENT (( #80853 ) ) ;
#17696=STYLED_ITEM ( 'NONE', ( #50691 ), #13350 ) ;
#17709=CARTESIAN_POINT ( 'NONE',  ( 9.187500000000001776, 4.461849672132297329, -4.461849672132302658 ) ) ;
#17727=AXIS2_PLACEMENT_3D ( 'NONE', #83932, #137571, #94743 ) ;
#17730=CARTESIAN_POINT ( 'NONE',  ( 180.9243601523648692, -48.88932940808381034, -39.16623080367945420 ) ) ;
#17743=AXIS2_PLACEMENT_3D ( 'NONE', #91886, #66069, #88525 ) ;
#17747=CARTESIAN_POINT ( 'NONE',  ( 15.21247294953710671, 0.000000000000000000, 6.094999999999989981 ) ) ;
#17779=CARTESIAN_POINT ( 'NONE',  ( 32.79123647476855297, -9.717572351234235426E-16, -7.934999999999990727 ) ) ;
#17790=DIRECTION ( 'NONE',  ( 0.000000000000000000, 1.000000000000000000, -2.556434596176436916E-15 ) ) ;
#17792=AXIS2_PLACEMENT_3D ( 'NONE', #133722, #113366, #67788 ) ;
#17794=CARTESIAN_POINT ( 'NONE',  ( 0.2242312616510835910, -48.73293412427781846, -38.67339632249748149 ) ) ;
#17826=DIRECTION ( 'NONE',  ( 0.000000000000000000, 0.000000000000000000, 1.000000000000000000 ) ) ;
#17828=CARTESIAN_POINT ( 'NONE',  ( 29.60416666666666430, -1.633150327867691987, -6.094999999999989093 ) ) ;
#17845=CARTESIAN_POINT ( 'NONE',  ( 13.70833333333333393, 3.047499999999997655, 5.278424836066143655 ) ) ;
#17880=ORIENTED_EDGE ( 'NONE', *, *, #122261, .T. ) ;
#17890=CARTESIAN_POINT ( 'NONE',  ( 151.4000000000000057, -16.48000000000005016, -12.70000000000045404 ) ) ;
#17900=EDGE_LOOP ( 'NONE', ( #114158, #111690, #4831, #143309, #130354, #67370, #13975, #59741, #61371, #27387, #37932, #61730, #47743, #124177, #64216, #119409, #122662, #46592 ) ) ;
#17916=DIRECTION ( 'NONE',  ( 0.000000000000000000, 0.000000000000000000, 1.000000000000000000 ) ) ;
#17921=SURFACE_SIDE_STYLE ('',( #35472 ) ) ;
#17923=ORIENTED_EDGE ( 'NONE', *, *, #47686, .T. ) ;
#17935=SURFACE_SIDE_STYLE ('',( #31013 ) ) ;
#17940=CARTESIAN_POINT ( 'NONE',  ( 3.770403141435219041, -7.934999999999989839, 2.126176841940957907 ) ) ;
#17974=AXIS2_PLACEMENT_3D ( 'NONE', #64500, #40622, #7954 ) ;
#17981=CARTESIAN_POINT ( 'NONE',  ( 27.68706980810188867, -2.126176841940956130, 7.934999999999991616 ) ) ;
#17982=CARTESIAN_POINT ( 'NONE',  ( 7.853736474768552966, -5.808823158059035485, -5.808823158059033709 ) ) ;
#18000=CARTESIAN_POINT ( 'NONE',  ( 25.39999999999999858, 0.000000000000000000, 0.000000000000000000 ) ) ;
#18008=CARTESIAN_POINT ( 'NONE',  ( 61.46640106136304382, -43.15000000000001279, 34.92499999999998295 ) ) ;
#18011=ORIENTED_EDGE ( 'NONE', *, *, #44136, .F. ) ;
#18038=CARTESIAN_POINT ( 'NONE',  ( 7.650403141435218934, 7.934999999999988951, -2.126176841940961904 ) ) ;
#18047=CARTESIAN_POINT ( 'NONE',  ( 17.50000000000000000, 0.000000000000000000, 6.094999999999989981 ) ) ;
#18060=CARTESIAN_POINT ( 'NONE',  ( 25.39999999999999503, 2.515948873491120175, -7.536568151888201506 ) ) ;
#18084=DIRECTION ( 'NONE',  ( -1.000000000000000000, -0.000000000000000000, -0.000000000000000000 ) ) ;
#18097=EDGE_CURVE ( 'NONE', #81966, #87517, #84065, .T. ) ;
#18106=CARTESIAN_POINT ( 'NONE',  ( 6.921236474768553748, -9.717572351234235426E-16, -7.934999999999990727 ) ) ;
#18114=DIRECTION ( 'NONE',  ( 0.000000000000000000, 0.000000000000000000, -1.000000000000000000 ) ) ;
#18120=CARTESIAN_POINT ( 'NONE',  ( 181.1395720402182974, -48.08977582060997946, -37.49964900842754645 ) ) ;
#18170=AXIS2_PLACEMENT_3D ( 'NONE', #73816, #105694, #140483 ) ;
#18178=CARTESIAN_POINT ( 'NONE',  ( 0.000000000000000000, -49.85820393249936444, -34.92499999999998295 ) ) ;
#18244=AXIS2_PLACEMENT_3D ( 'NONE', #74510, #118695, #120088 ) ;
#18282=VECTOR ( 'NONE', #35458, 1000.000000000000000 ) ;
#18284=CARTESIAN_POINT ( 'NONE',  ( 6.337903141435219823, -6.871911579029513106, -3.967499999999993587 ) ) ;
#18294=CARTESIAN_POINT ( 'NONE',  ( 11.12913961620377101, 5.278424836066147208, 3.047499999999990550 ) ) ;
#18315=CARTESIAN_POINT ( 'NONE',  ( 15.43706980810188512, 2.126176841940952134, -7.934999999999993392 ) ) ;
#18319=VERTEX_POINT ( 'NONE', #61825 ) ;
#18321=CARTESIAN_POINT ( 'NONE',  ( 128.5894344200537489, -52.00875322212550600, 39.86617647058822911 ) ) ;
#18322=CARTESIAN_POINT ( 'NONE',  ( 4.858306282870439752, -1.633150327867700202, 6.094999999999985540 ) ) ;
#18361=CARTESIAN_POINT ( 'NONE',  ( 24.39999999999999858, -2.600000000000060929, 28.92500000000001492 ) ) ;
#18383=ADVANCED_FACE ( 'NONE', ( #64657 ), #139873, .T. ) ;
#18386=( LENGTH_UNIT ( ) NAMED_UNIT ( * ) SI_UNIT ( .MILLI., .METRE. ) );
#18400=STYLED_ITEM ( 'NONE', ( #98950 ), #21720 ) ;
#18402=FILL_AREA_STYLE ('',( #86569 ) ) ;
#18452=CARTESIAN_POINT ( 'NONE',  ( 11.12913961620377101, 5.278424836066147208, 3.047499999999990550 ) ) ;
#18470=EDGE_LOOP ( 'NONE', ( #57873, #76751, #93519 ) ) ;
#18488=CARTESIAN_POINT ( 'NONE',  ( 29.43706980810189222, 2.126176841940952134, -7.934999999999993392 ) ) ;
#18510=CARTESIAN_POINT ( 'NONE',  ( 19.25000000000000355, -7.464222240803106570E-16, -6.094999999999989981 ) ) ;
#18534=CARTESIAN_POINT ( 'NONE',  ( 31.93750000000000355, -4.461849672132299105, 4.461849672132299993 ) ) ;
#18544=AXIS2_PLACEMENT_3D ( 'NONE', #14038, #24232, #135160 ) ;
#18589=CARTESIAN_POINT ( 'NONE',  ( 25.40000000000000568, -6.374262171851336589, -2.013297974899656229 ) ) ;
#18590=DIRECTION ( 'NONE',  ( -0.000000000000000000, 1.000000000000000000, -0.000000000000000000 ) ) ;
#18593=DIRECTION ( 'NONE',  ( -0.000000000000000000, -0.000000000000000000, 1.000000000000000000 ) ) ;
#18602=MECHANICAL_DESIGN_GEOMETRIC_PRESENTATION_REPRESENTATION('',(#14065),#113624);
#18607=FILL_AREA_STYLE ('',( #105616 ) ) ;
#18623=CARTESIAN_POINT ( 'NONE',  ( 12.58747294953710671, -6.094999999999989981, 3.732111120401553285E-16 ) ) ;
#18663=CARTESIAN_POINT ( 'NONE',  ( 5.957903141435219929, 6.871911579029515771, 3.967499999999989146 ) ) ;
#18691=CARTESIAN_POINT ( 'NONE',  ( 52.83697049268915436, -48.90295371244931033, -39.18578444878554734 ) ) ;
#18707=CARTESIAN_POINT ( 'NONE',  ( 2.333333333333333481, 5.278424836066143655, -3.047499999999997655 ) ) ;
#18708=AXIS2_PLACEMENT_3D ( 'NONE', #59274, #68024, #2693 ) ;
#18709=CARTESIAN_POINT ( 'NONE',  ( 4.207903141435219929, -6.871911579029513106, -3.967499999999993587 ) ) ;
#18741=CARTESIAN_POINT ( 'NONE',  ( 55.29044309249616163, -47.26730531257655343, 36.54674188582600181 ) ) ;
#18749=CARTESIAN_POINT ( 'NONE',  ( 125.3761450143286993, -47.18881911353552994, 35.55177538329112963 ) ) ;
#18775=CARTESIAN_POINT ( 'NONE',  ( 12.46290314143521982, -3.967499999999994476, 6.871911579029513106 ) ) ;
#18778=CARTESIAN_POINT ( 'NONE',  ( 21.72916666666666785, -6.094999999999989093, 1.633150327867691542 ) ) ;
#18810=ORIENTED_EDGE ( 'NONE', *, *, #92308, .T. ) ;
#18815=MECHANICAL_DESIGN_GEOMETRIC_PRESENTATION_REPRESENTATION('',(#134551),#2558);
#18829=ORIENTED_EDGE ( 'NONE', *, *, #15465, .F. ) ;
#18839=EDGE_CURVE ( 'NONE', #117948, #143110, #95954, .T. ) ;
#18849=CARTESIAN_POINT ( 'NONE',  ( 9.837903141435219823, -6.871911579029513106, -3.967499999999993587 ) ) ;
#18854=CARTESIAN_POINT ( 'NONE',  ( 27.99999999999996803, -49.14999999999999147, 49.92499999999997584 ) ) ;
#18911=ADVANCED_BREP_SHAPE_REPRESENTATION ( '', ( #90242, #127880 ), #141741 ) ;
#18931=CARTESIAN_POINT ( 'NONE',  ( 152.4000000000000057, -18.48000000000005372, -33.92499999999998295 ) ) ;
#18941=CARTESIAN_POINT ( 'NONE',  ( 2.000000000000008882, 7.464222240803104598E-16, -6.094999999999989093 ) ) ;
#18956=STYLED_ITEM ( 'NONE', ( #130273 ), #28818 ) ;
#18987=( GEOMETRIC_REPRESENTATION_CONTEXT ( 3 ) GLOBAL_UNCERTAINTY_ASSIGNED_CONTEXT ( ( #56376 ) ) GLOBAL_UNIT_ASSIGNED_CONTEXT ( ( #37717, #132948, #81957 ) ) REPRESENTATION_CONTEXT ( 'NONE', 'WORKASPACE' ) );
#19009=AXIS2_PLACEMENT_3D ( 'NONE', #89771, #123863, #112955 ) ;
#19024=ORIENTED_EDGE ( 'NONE', *, *, #121757, .T. ) ;
#19025=VERTEX_POINT ( 'NONE', #27373 ) ;
#19033=CARTESIAN_POINT ( 'NONE',  ( 22.08790314143522338, 6.871911579029515771, 3.967499999999989146 ) ) ;
#19065=CARTESIAN_POINT ( 'NONE',  ( 12.81206980810188512, 7.934999999999993392, 2.126176841940951689 ) ) ;
#19123=STYLED_ITEM ( 'NONE', ( #136610 ), #2933 ) ;
#19154=ORIENTED_EDGE ( 'NONE', *, *, #36349, .F. ) ;
#19158=CARTESIAN_POINT ( 'NONE',  ( 122.6835989386367771, -43.14999999999999147, -34.92499999999998295 ) ) ;
#19165=CARTESIAN_POINT ( 'NONE',  ( 0.000000000000000000, -57.15000000000003411, -15.92500000000064730 ) ) ;
#19195=ORIENTED_EDGE ( 'NONE', *, *, #15785, .F. ) ;
#19206=CARTESIAN_POINT ( 'NONE',  ( 24.25413961620377279, 3.047499999999993214, -5.278424836066146320 ) ) ;
#19239=CARTESIAN_POINT ( 'NONE',  ( 31.62456980810188867, -6.871911579029512218, 3.967499999999996252 ) ) ;
#19258=DIRECTION ( 'NONE',  ( 0.000000000000000000, -1.000000000000000000, 0.000000000000000000 ) ) ;
#19287=CARTESIAN_POINT ( 'NONE',  ( 32.22916666666666430, -6.094999999999989093, 1.633150327867691765 ) ) ;
#19295=DIRECTION ( 'NONE',  ( 1.000000000000000000, 0.000000000000000000, -0.000000000000000000 ) ) ;
#19310=CARTESIAN_POINT ( 'NONE',  ( 181.1500000000000057, -3.180000000000061444, -34.92499999999998295 ) ) ;
#19324=CARTESIAN_POINT ( 'NONE',  ( 181.1500000000000057, -43.14999999999999147, -31.92499999999998295 ) ) ;
#19368=ORIENTED_EDGE ( 'NONE', *, *, #97359, .F. ) ;
#19375=FACE_OUTER_BOUND ( 'NONE', #17900, .T. ) ;
#19380=DIRECTION ( 'NONE',  ( -1.000000000000000000, 0.000000000000000000, 0.000000000000000000 ) ) ;
#19397=CARTESIAN_POINT ( 'NONE',  ( 0.4397996348757138296, -49.08473565290604768, 39.91868829876761282 ) ) ;
#19401=CARTESIAN_POINT ( 'NONE',  ( 3.624569808101886448, -6.871911579029512218, 3.967499999999996252 ) ) ;
#19428=CARTESIAN_POINT ( 'NONE',  ( 53.19685992802465080, -48.66302742222551103, -38.53170190052302502 ) ) ;
#19447=CARTESIAN_POINT ( 'NONE',  ( 1.458333333333333481, -3.047499999999997211, -5.278424836066143655 ) ) ;
#19448=CARTESIAN_POINT ( 'NONE',  ( 16.89540314143521726, 2.126176841940962348, 7.934999999999988951 ) ) ;
#19470=CARTESIAN_POINT ( 'NONE',  ( 0.5457257104438434370, -52.10338527932237440, 40.45859298138252313 ) ) ;
#19477=ORIENTED_EDGE ( 'NONE', *, *, #7015, .F. ) ;
#19489=COLOUR_RGB ( '', 0.31764706, 0.68627451, 0.89019608) ;
#19501=CARTESIAN_POINT ( 'NONE',  ( 16.98373647476855197, -5.808823158059035485, -5.808823158059033709 ) ) ;
#19512=DIRECTION ( 'NONE',  ( 0.000000000000000000, 0.000000000000000000, 1.000000000000000000 ) ) ;
#19519=( GEOMETRIC_REPRESENTATION_CONTEXT ( 3 ) GLOBAL_UNCERTAINTY_ASSIGNED_CONTEXT ( ( #93804 ) ) GLOBAL_UNIT_ASSIGNED_CONTEXT ( ( #39029, #17272, #7802 ) ) REPRESENTATION_CONTEXT ( 'NONE', 'WORKASPACE' ) );
#19526=CYLINDRICAL_SURFACE ( 'NONE', #88124, 6.094999999999989093 ) ;
#19530=CARTESIAN_POINT ( 'NONE',  ( 25.40000000000002345, 4.163866272544239244, -6.757773473734751235 ) ) ;
#19538=VECTOR ( 'NONE', #37042, 1000.000000000000000 ) ;
#19565=VERTEX_POINT ( 'NONE', #28503 ) ;
#19571=CARTESIAN_POINT ( 'NONE',  ( 11.58790314143521982, 6.871911579029515771, 3.967499999999989146 ) ) ;
#19597=CARTESIAN_POINT ( 'NONE',  ( 3.681769877398668738E-15, -50.24077216217759911, -35.40405119785167898 ) ) ;
#19611=CARTESIAN_POINT ( 'NONE',  ( 0.1600000000000015299, -4.429882875875668091, -6.591932758761664957 ) ) ;
#19621=VERTEX_POINT ( 'NONE', #116917 ) ;
#19662=( LENGTH_UNIT ( ) NAMED_UNIT ( * ) SI_UNIT ( .MILLI., .METRE. ) );
#19677=DIRECTION ( 'NONE',  ( -0.000000000000000000, 1.000000000000000000, -0.000000000000000000 ) ) ;
#19692=DIRECTION ( 'NONE',  ( -1.000000000000000000, -0.000000000000000000, -0.000000000000000000 ) ) ;
#19700=SURFACE_SIDE_STYLE ('',( #8089 ) ) ;
#19712=SURFACE_SIDE_STYLE ('',( #39358 ) ) ;
#19724=CARTESIAN_POINT ( 'NONE',  ( 184.1499999999998067, -3.180000000000061444, -31.92499999999998295 ) ) ;
#19741=CARTESIAN_POINT ( 'NONE',  ( 13.77540314143521982, -2.126176841940958351, -7.934999999999989839 ) ) ;
#19756=CARTESIAN_POINT ( 'NONE',  ( 152.4000000000000057, -16.48000000000005016, 34.92499999999998295 ) ) ;
#19767=CARTESIAN_POINT ( 'NONE',  ( 25.39999999999999858, -7.600000000000055600, -28.92499999999998650 ) ) ;
#19773=CARTESIAN_POINT ( 'NONE',  ( 13.83290314143522082, -3.967499999999994476, 6.871911579029513106 ) ) ;
#19784=EDGE_LOOP ( 'NONE', ( #54390, #136319, #10554, #86439 ) ) ;
#19827=SURFACE_STYLE_FILL_AREA ( #107555 ) ;
#19853=SURFACE_SIDE_STYLE ('',( #7541 ) ) ;
#19871=ORIENTED_EDGE ( 'NONE', *, *, #15596, .T. ) ;
#19882=LINE ( 'NONE', #118487, #68987 ) ;
#19899=CARTESIAN_POINT ( 'NONE',  ( 21.48330628287043709, 6.094999999999991758, 1.633150327867687102 ) ) ;
#19917=DIRECTION ( 'NONE',  ( 0.000000000000000000, 0.000000000000000000, 1.000000000000000000 ) ) ;
#19971=CARTESIAN_POINT ( 'NONE',  ( 28.00000000000002487, -49.14999999999999147, -34.92499999999976978 ) ) ;
#19981=CARTESIAN_POINT ( 'NONE',  ( 29.31249999999999645, -4.461849672132299993, -4.461849672132299105 ) ) ;
#19999=SURFACE_STYLE_USAGE ( .BOTH. , #88146 ) ;
#20041=ORIENTED_EDGE ( 'NONE', *, *, #15596, .F. ) ;
#20042=CARTESIAN_POINT ( 'NONE',  ( 184.0776099992040429, -48.13855614193184351, 37.56434003615978412 ) ) ;
#20093=CARTESIAN_POINT ( 'NONE',  ( 3.060608989244792966, -48.47007572038103262, 38.12657027910959329 ) ) ;
#20097=CARTESIAN_POINT ( 'NONE',  ( 0.8537364747685527444, -5.808823158059035485, -5.808823158059033709 ) ) ;
#20106=FILL_AREA_STYLE_COLOUR ( '', #41770 ) ;
#20136=CIRCLE ( 'NONE', #34043, 2.999999999999999112 ) ;
#20144=CARTESIAN_POINT ( 'NONE',  ( 6.854166666666666075, 1.633150327867695095, 6.094999999999988205 ) ) ;
#20145=CARTESIAN_POINT ( 'NONE',  ( 12.52040314143522082, 7.934999999999988951, -2.126176841940961904 ) ) ;
#20158=CARTESIAN_POINT ( 'NONE',  ( 0.07085943933668231720, -51.15040958483978528, 36.98623100868706359 ) ) ;
#20173=CARTESIAN_POINT ( 'NONE',  ( 128.2885478629722229, -48.75494892434343797, 38.51155878621300843 ) ) ;
#20183=STYLED_ITEM ( 'NONE', ( #50659 ), #12196 ) ;
#20194=CARTESIAN_POINT ( 'NONE',  ( 14.06706980810188590, 2.126176841940952134, -7.934999999999992504 ) ) ;
#20203=EDGE_LOOP ( 'NONE', ( #115251, #128342, #132191, #140285 ) ) ;
#20224=EDGE_LOOP ( 'NONE', ( #140393, #132355, #25041 ) ) ;
#20269=CARTESIAN_POINT ( 'NONE',  ( 9.692069808101887674, -7.934999999999991616, -2.126176841940955242 ) ) ;
#20276=VERTEX_POINT ( 'NONE', #23681 ) ;
#20321=EDGE_LOOP ( 'NONE', ( #120258, #37792, #37700, #100204 ) ) ;
#20329=CARTESIAN_POINT ( 'NONE',  ( 25.39999999999999858, -43.14999999999999147, 40.92499999999998295 ) ) ;
#20339=CARTESIAN_POINT ( 'NONE',  ( 23.47916666666666785, 6.094999999999988205, -1.633150327867694651 ) ) ;
#20341=AXIS2_PLACEMENT_3D ( 'NONE', #91567, #5238, #116168 ) ;
#20424=CARTESIAN_POINT ( 'NONE',  ( 19.14997294953710494, -4.461849672132299105, 4.461849672132299993 ) ) ;
#20435=VERTEX_POINT ( 'NONE', #114930 ) ;
#20440=CARTESIAN_POINT ( 'NONE',  ( 16.25456980810188767, -6.871911579029512218, 3.967499999999996252 ) ) ;
#20466=CARTESIAN_POINT ( 'NONE',  ( 4.229166666666666963, -6.094999999999989093, 1.633150327867691542 ) ) ;
#20475=CARTESIAN_POINT ( 'NONE',  ( 0.000000000000000000, -4.600000000000055600, -28.92500000000000071 ) ) ;
#20477=( NAMED_UNIT ( * ) SI_UNIT ( $, .STERADIAN. ) SOLID_ANGLE_UNIT ( ) );
#20529=FACE_OUTER_BOUND ( 'NONE', #37565, .T. ) ;
#20534=CARTESIAN_POINT ( 'NONE',  ( 9.379139616203772789, -5.278424836066145431, -3.047499999999993658 ) ) ;
#20545=EDGE_CURVE ( 'NONE', #93784, #20276, #4285, .T. ) ;
#20556=DIRECTION ( 'NONE',  ( -1.000000000000000000, -0.000000000000000000, -0.000000000000000000 ) ) ;
#20578=EDGE_CURVE ( 'NONE', #21546, #62052, #124712, .T. ) ;
#20614=CARTESIAN_POINT ( 'NONE',  ( 25.71247294953710849, 0.000000000000000000, 6.094999999999989981 ) ) ;
#20626=DIRECTION ( 'NONE',  ( -1.000000000000000000, -0.000000000000000000, 0.000000000000000000 ) ) ;
#20634=CARTESIAN_POINT ( 'NONE',  ( 2.999999999999999112, -47.62213595499956398, -36.92499999999996874 ) ) ;
#20644=ORIENTED_EDGE ( 'NONE', *, *, #68373, .F. ) ;
#20661=( NAMED_UNIT ( * ) SI_UNIT ( $, .STERADIAN. ) SOLID_ANGLE_UNIT ( ) );
#20701=CARTESIAN_POINT ( 'NONE',  ( 34.70833333333333570, 3.047499999999997655, 5.278424836066143655 ) ) ;
#20707=CARTESIAN_POINT ( 'NONE',  ( 0.000000000000000000, -43.14999999999999147, 40.92499999999998295 ) ) ;
#20711=CARTESIAN_POINT ( 'NONE',  ( 2.999999999999999112, -1.600000000000060929, 28.92500000000001847 ) ) ;
#20721=CARTESIAN_POINT ( 'NONE',  ( 24.39999999999999858, -7.600000000000055600, -28.92499999999998650 ) ) ;
#20751=CARTESIAN_POINT ( 'NONE',  ( 181.1500000000000057, -47.62213595499959951, 36.92500000000000426 ) ) ;
#20761=EDGE_LOOP ( 'NONE', ( #17221, #59005, #20837, #80904 ) ) ;
#20765=CARTESIAN_POINT ( 'NONE',  ( 183.3316408629057719, -49.14999999999998437, 41.64499999999997470 ) ) ;
#20774=EDGE_CURVE ( 'NONE', #97401, #17549, #45306, .T. ) ;
#20775=CARTESIAN_POINT ( 'NONE',  ( 2.233306282870438864, -6.094999999999989981, -1.633150327867689322 ) ) ;
#20817=CARTESIAN_POINT ( 'NONE',  ( 14.85373647476855474, -5.808823158059035485, -5.808823158059033709 ) ) ;
#20837=ORIENTED_EDGE ( 'NONE', *, *, #142868, .F. ) ;
#20852=AXIS2_PLACEMENT_3D ( 'NONE', #123052, #134657, #23728 ) ;
#20854=( NAMED_UNIT ( * ) PLANE_ANGLE_UNIT ( ) SI_UNIT ( $, .RADIAN. ) );
#20861=CARTESIAN_POINT ( 'NONE',  ( 3.062499999999999556, 4.461849672132300881, 4.461849672132299105 ) ) ;
#20862=CARTESIAN_POINT ( 'NONE',  ( 16.16623647476855652, 7.934999999999990727, -1.457635852685135314E-15 ) ) ;
#20903=CARTESIAN_POINT ( 'NONE',  ( 184.1500000000000057, -30.18000000000009564, -15.92500000000064375 ) ) ;
#20916=CARTESIAN_POINT ( 'NONE',  ( 14.79623647476855375, 7.934999999999990727, -1.457635852685135314E-15 ) ) ;
#20929=ADVANCED_FACE ( 'NONE', ( #29214 ), #73459, .T. ) ;
#20969=CARTESIAN_POINT ( 'NONE',  ( 184.1499999999998067, -3.180000000000061444, -34.92499999999998295 ) ) ;
#20991=CARTESIAN_POINT ( 'NONE',  ( 17.85873647476854842, 5.808823158059031044, -5.808823158059038150 ) ) ;
#20992=ORIENTED_EDGE ( 'NONE', *, *, #124402, .T. ) ;
#21024=CARTESIAN_POINT ( 'NONE',  ( 174.7500000000000000, 7.919999999999947526, 19.12499999999998224 ) ) ;
#21033=CARTESIAN_POINT ( 'NONE',  ( 24.39999999999999858, -1.600000000000094458, 34.92499999999998295 ) ) ;
#21035=CARTESIAN_POINT ( 'NONE',  ( 27.99999999999996803, -57.14999999999999147, 49.92499999999997584 ) ) ;
#21129=CARTESIAN_POINT ( 'NONE',  ( 24.54580628287043709, 5.278424836066143655, -3.047499999999997655 ) ) ;
#21169=MECHANICAL_DESIGN_GEOMETRIC_PRESENTATION_REPRESENTATION('',(#72138),#44388);
#21172=CARTESIAN_POINT ( 'NONE',  ( 20.77540314143522338, -2.126176841940958351, -7.934999999999989839 ) ) ;
#21187=COLOUR_RGB ( '', 0.31764706, 0.68627451, 0.89019608) ;
#21226=COLOUR_RGB ( '', 0.66274510, 0.83137255, 0.94901961) ;
#21254=ADVANCED_FACE ( 'NONE', ( #42007 ), #74641, .F. ) ;
#21270=CARTESIAN_POINT ( 'NONE',  ( 2.999999999999999112, 1.194621026894846283, 17.40906030209848510 ) ) ;
#21280=ORIENTED_EDGE ( 'NONE', *, *, #48904, .F. ) ;
#21339=PRESENTATION_STYLE_ASSIGNMENT (( #53997 ) ) ;
#21350=CARTESIAN_POINT ( 'NONE',  ( 22.64997294953710139, -4.461849672132299105, 4.461849672132299993 ) ) ;
#21369=DIRECTION ( 'NONE',  ( 0.000000000000000000, -1.000000000000000000, 0.000000000000000000 ) ) ;
#21381=EDGE_CURVE ( 'NONE', #75731, #138987, #113759, .T. ) ;
#21398=CARTESIAN_POINT ( 'NONE',  ( 55.18164086290604331, -52.14999999999999147, 41.64499999999997470 ) ) ;
#21417=FILL_AREA_STYLE_COLOUR ( '', #13751 ) ;
#21424=UNCERTAINTY_MEASURE_WITH_UNIT (LENGTH_MEASURE( 1.000000000000000082E-05 ), #3737, 'distance_accuracy_value', 'NONE');
#21427=CARTESIAN_POINT ( 'NONE',  ( 15.79580628287043709, -5.278424836066144543, 3.047499999999995879 ) ) ;
#21431=ORIENTED_EDGE ( 'NONE', *, *, #33078, .F. ) ;
#21451=CARTESIAN_POINT ( 'NONE',  ( 55.18164086290604331, -52.14999999999999147, 41.64499999999997470 ) ) ;
#21476=EDGE_LOOP ( 'NONE', ( #11148, #78784, #120786, #38436 ) ) ;
#21478=COLOUR_RGB ( '', 0.08235294, 0.09019608, 0.10196078) ;
#21500=CARTESIAN_POINT ( 'NONE',  ( 180.9285571751892121, -48.88296141031990061, 39.14553452061912253 ) ) ;
#21524=CARTESIAN_POINT ( 'NONE',  ( 0.3374729495371057708, 6.094999999999989981, -1.119633336120465690E-15 ) ) ;
#21533=CARTESIAN_POINT ( 'NONE',  ( 152.4000000000000057, -17.48000000000005016, -12.70000000000043272 ) ) ;
#21546=VERTEX_POINT ( 'NONE', #74386 ) ;
#21552=CARTESIAN_POINT ( 'NONE',  ( 15.43706980810188512, 2.126176841940952134, -7.934999999999993392 ) ) ;
#21555=DIRECTION ( 'NONE',  ( -0.000000000000000000, 1.000000000000000000, -0.000000000000000000 ) ) ;
#21563=UNCERTAINTY_MEASURE_WITH_UNIT (LENGTH_MEASURE( 1.000000000000000082E-05 ), #129652, 'distance_accuracy_value', 'NONE');
#21581=CARTESIAN_POINT ( 'NONE',  ( 17.39997294953710494, 4.461849672132297329, -4.461849672132302658 ) ) ;
#21599=CARTESIAN_POINT ( 'NONE',  ( 16.77083333333333570, 6.094999999999991758, 1.633150327867687102 ) ) ;
#21600=CARTESIAN_POINT ( 'NONE',  ( 17.18706980810188867, -2.126176841940956130, 7.934999999999990727 ) ) ;
#21612=( NAMED_UNIT ( * ) PLANE_ANGLE_UNIT ( ) SI_UNIT ( $, .RADIAN. ) );
#21614=( NAMED_UNIT ( * ) PLANE_ANGLE_UNIT ( ) SI_UNIT ( $, .RADIAN. ) );
#21634=VECTOR ( 'NONE', #86657, 1000.000000000000000 ) ;
#21637=CARTESIAN_POINT ( 'NONE',  ( 131.5423521607622490, -49.05583548141699879, 39.86617647058824332 ) ) ;
#21647=VECTOR ( 'NONE', #48689, 1000.000000000000000 ) ;
#21656=EDGE_CURVE ( 'NONE', #66484, #119012, #121424, .T. ) ;
#21657=CARTESIAN_POINT ( 'NONE',  ( 15.52540314143521982, 2.126176841940962348, 7.934999999999988951 ) ) ;
#21660=CARTESIAN_POINT ( 'NONE',  ( 166.0564677593420981, 26.96999999999993847, 33.42388977641238057 ) ) ;
#21667=ORIENTED_EDGE ( 'NONE', *, *, #38988, .T. ) ;
#21700=MECHANICAL_DESIGN_GEOMETRIC_PRESENTATION_REPRESENTATION('',(#109659),#12478);
#21711=CARTESIAN_POINT ( 'NONE',  ( 14.19163961620377279, 6.094999999999988205, -1.633150327867694651 ) ) ;
#21720=ADVANCED_FACE ( 'NONE', ( #57633 ), #113310, .T. ) ;
#21722=CARTESIAN_POINT ( 'NONE',  ( 20.04623647476855197, -7.934999999999990727, 4.858786175617117713E-16 ) ) ;
#21728=CARTESIAN_POINT ( 'NONE',  ( 55.32830738432631534, -52.14999999996970814, -41.05175048930665582 ) ) ;
#21802=EDGE_LOOP ( 'NONE', ( #109164, #121829, #93633, #105213 ) ) ;
#21826=COLOUR_RGB ( '', 0.40784314, 0.44705882, 0.49803922) ;
#21837=VERTEX_POINT ( 'NONE', #3206 ) ;
#21850=DIRECTION ( 'NONE',  ( 0.000000000000000000, 0.000000000000000000, 1.000000000000000000 ) ) ;
#21857=VERTEX_POINT ( 'NONE', #62614 ) ;
#21874=CARTESIAN_POINT ( 'NONE',  ( 163.1938454491095456, 26.96999999999994557, -34.65286652761894715 ) ) ;
#21882=CARTESIAN_POINT ( 'NONE',  ( 28.79623647476855197, 7.934999999999990727, -1.457635852685135314E-15 ) ) ;
#21900=AXIS2_PLACEMENT_3D ( 'NONE', #32280, #3695, #43162 ) ;
#21948=LINE ( 'NONE', #110364, #77392 ) ;
#21979=CARTESIAN_POINT ( 'NONE',  ( 14.87500000000000178, -6.094999999999989981, 3.732111120401553285E-16 ) ) ;
#21987=STYLED_ITEM ( 'NONE', ( #79246 ), #90242 ) ;
#21988=CARTESIAN_POINT ( 'NONE',  ( 0.1600000000000009748, -7.113645484598424495, 3.515717980648092045 ) ) ;
#21989=CARTESIAN_POINT ( 'NONE',  ( 25.39999999999999858, -16.48000000000005016, -12.70000000000045404 ) ) ;
#21990=( LENGTH_UNIT ( ) NAMED_UNIT ( * ) SI_UNIT ( .MILLI., .METRE. ) );
#21997=ORIENTED_EDGE ( 'NONE', *, *, #60183, .T. ) ;
#22012=MECHANICAL_DESIGN_GEOMETRIC_PRESENTATION_REPRESENTATION('',(#103055),#24307);
#22040=CARTESIAN_POINT ( 'NONE',  ( 130.7379471109758242, -48.51956544822604656, -36.87500513592858198 ) ) ;
#22042=CARTESIAN_POINT ( 'NONE',  ( 23.96247294953710849, -7.464222240803106570E-16, -6.094999999999989981 ) ) ;
#22053=CARTESIAN_POINT ( 'NONE',  ( 25.39999999999999858, 0.000000000000000000, 6.094999999999989093 ) ) ;
#22075=FILL_AREA_STYLE_COLOUR ( '', #114528 ) ;
#22085=FILL_AREA_STYLE ('',( #121402 ) ) ;
#22088=SURFACE_SIDE_STYLE ('',( #121406 ) ) ;
#22173=ORIENTED_EDGE ( 'NONE', *, *, #97475, .F. ) ;
#22207=CARTESIAN_POINT ( 'NONE',  ( -0.5375270504628941737, -7.464222240803106570E-16, -6.094999999999989981 ) ) ;
#22210=AXIS2_PLACEMENT_3D ( 'NONE', #18931, #6582, #50857 ) ;
#22213=DIRECTION ( 'NONE',  ( -1.000000000000000000, -0.000000000000000000, -0.000000000000000000 ) ) ;
#22231=CARTESIAN_POINT ( 'NONE',  ( 10.04123647476855297, 0.000000000000000000, 7.934999999999990727 ) ) ;
#22245=DIRECTION ( 'NONE',  ( 0.000000000000000000, -1.000000000000000000, 0.000000000000000000 ) ) ;
#22265=FACE_OUTER_BOUND ( 'NONE', #34885, .T. ) ;
#22270=CARTESIAN_POINT ( 'NONE',  ( 14.87500000000000178, -6.094999999999989981, 3.732111120401553285E-16 ) ) ;
#22271=CARTESIAN_POINT ( 'NONE',  ( 17.33290314143522082, -3.967499999999994476, 6.871911579029513106 ) ) ;
#22287=DIRECTION ( 'NONE',  ( 0.000000000000000000, 0.000000000000000000, -1.000000000000000000 ) ) ;
#22324=CARTESIAN_POINT ( 'NONE',  ( 13.77540314143521982, -2.126176841940958351, -7.934999999999988951 ) ) ;
#22335=CARTESIAN_POINT ( 'NONE',  ( 0.000000000000000000, -4.600000000000055600, -28.92500000000000071 ) ) ;
#22338=ORIENTED_EDGE ( 'NONE', *, *, #24835, .F. ) ;
#22352=SURFACE_SIDE_STYLE ('',( #57909 ) ) ;
#22374=CARTESIAN_POINT ( 'NONE',  ( 0.000000000000000000, -30.18000000000009564, -12.70000000000045404 ) ) ;
#22381=ADVANCED_FACE ( 'NONE', ( #94337 ), #39268, .F. ) ;
#22390=( GEOMETRIC_REPRESENTATION_CONTEXT ( 3 ) GLOBAL_UNCERTAINTY_ASSIGNED_CONTEXT ( ( #101105 ) ) GLOBAL_UNIT_ASSIGNED_CONTEXT ( ( #21990, #108985, #142373 ) ) REPRESENTATION_CONTEXT ( 'NONE', 'WORKASPACE' ) );
#22401=CARTESIAN_POINT ( 'NONE',  ( 17.27540314143521627, -2.126176841940958351, -7.934999999999989839 ) ) ;
#22416=CARTESIAN_POINT ( 'NONE',  ( 55.56056557994607914, -57.14999999999999147, 39.86617647058822200 ) ) ;
#22419=DIRECTION ( 'NONE',  ( 0.000000000000000000, -1.000000000000000000, 0.000000000000000000 ) ) ;
#22445=CARTESIAN_POINT ( 'NONE',  ( 20.39540314143521726, 2.126176841940962348, 7.934999999999989839 ) ) ;
#22452=( BOUNDED_CURVE ( )  B_SPLINE_CURVE ( 2, ( #84748, #85436, #30360, #71753, #105066, #5727, #28942, #49995, #94178, #127534, #29630, #73183, #73873 ),
 .UNSPECIFIED., .F., .F. ) 
 B_SPLINE_CURVE_WITH_KNOTS ( ( 3, 2, 2, 2, 2, 2, 3 ),
 ( 0.2000000000000000666, 0.2083333333333333981, 0.2166666666666667018, 0.2250000000000000333, 0.2333333333333333648, 0.2416666666666666963, 0.2500000000000000000 ),
 .UNSPECIFIED. ) 
 CURVE ( )  GEOMETRIC_REPRESENTATION_ITEM ( )  RATIONAL_B_SPLINE_CURVE ( ( 0.9999999999999997780, 0.9659258262890685343, 1.000000000000000000, 0.9659258262890683122, 1.000000000000000000, 0.9659258262890683122, 1.000000000000000000, 0.9659258262890683122, 1.000000000000000000, 0.9659258262890683122, 1.000000000000000000, 0.9659258262890683122, 1.000000000000000000 ) ) 
 REPRESENTATION_ITEM ( '' )  );
#22520=SURFACE_STYLE_FILL_AREA ( #77668 ) ;
#22538=SURFACE_STYLE_USAGE ( .BOTH. , #121860 ) ;
#22542=DIRECTION ( 'NONE',  ( 1.000000000000000000, 0.000000000000000000, -0.000000000000000000 ) ) ;
#22562=CARTESIAN_POINT ( 'NONE',  ( 181.1500000000000057, 0.000000000000000000, 31.92499999999998295 ) ) ;
#22563=CARTESIAN_POINT ( 'NONE',  ( 31.56706980810188767, 2.126176841940952134, -7.934999999999993392 ) ) ;
#22567=MECHANICAL_DESIGN_GEOMETRIC_PRESENTATION_REPRESENTATION('',(#85107),#27242);
#22576=DIRECTION ( 'NONE',  ( 0.000000000000000000, -3.469446951953615372E-15, 1.000000000000000000 ) ) ;
#22614=ADVANCED_FACE ( 'NONE', ( #68885 ), #74217, .F. ) ;
#22657=AXIS2_PLACEMENT_3D ( 'NONE', #47583, #67912, #36647 ) ;
#22667=PRESENTATION_STYLE_ASSIGNMENT (( #30752 ) ) ;
#22688=EDGE_CURVE ( 'NONE', #53362, #116882, #30218, .T. ) ;
#22692=LINE ( 'NONE', #13971, #35260 ) ;
#22734=CARTESIAN_POINT ( 'NONE',  ( 0.06706980810188606368, 2.126176841940952134, -7.934999999999993392 ) ) ;
#22782=DIRECTION ( 'NONE',  ( 0.000000000000000000, 6.938893903907227589E-15, -1.000000000000000000 ) ) ;
#22802=CARTESIAN_POINT ( 'NONE',  ( 16.96247294953710849, -7.464222240803106570E-16, -6.094999999999989981 ) ) ;
#22858=ORIENTED_EDGE ( 'NONE', *, *, #76935, .T. ) ;
#22879=CARTESIAN_POINT ( 'NONE',  ( 3.691639616203772789, 6.094999999999988205, -1.633150327867694651 ) ) ;
#22886=PRESENTATION_STYLE_ASSIGNMENT (( #102648 ) ) ;
#22907=CARTESIAN_POINT ( 'NONE',  ( 7.191639616203771013, 6.094999999999988205, -1.633150327867694651 ) ) ;
#22934=CARTESIAN_POINT ( 'NONE',  ( 9.312069808101886892, 7.934999999999993392, 2.126176841940951689 ) ) ;
#22935=CARTESIAN_POINT ( 'NONE',  ( 0.000000000000000000, 0.000000000000000000, 8.094999999999991758 ) ) ;
#22938=EDGE_LOOP ( 'NONE', ( #93958, #2219, #9308, #81247 ) ) ;
#22942=PRESENTATION_STYLE_ASSIGNMENT (( #109983 ) ) ;
#22943=UNCERTAINTY_MEASURE_WITH_UNIT (LENGTH_MEASURE( 1.000000000000000082E-05 ), #114451, 'distance_accuracy_value', 'NONE');
#22944=MECHANICAL_DESIGN_GEOMETRIC_PRESENTATION_REPRESENTATION('',(#76294),#36844);
#22966=EDGE_CURVE ( 'NONE', #19025, #20435, #125229, .T. ) ;
#22967=CARTESIAN_POINT ( 'NONE',  ( 27.99999999999996803, -49.14999999999999147, 45.92499999999999005 ) ) ;
#22976=CARTESIAN_POINT ( 'NONE',  ( 156.1499999999997783, -49.14999999999999147, -34.92499999999975557 ) ) ;
#22979=CARTESIAN_POINT ( 'NONE',  ( 16.04166666666666785, 3.047499999999993214, -5.278424836066146320 ) ) ;
#23013=ORIENTED_EDGE ( 'NONE', *, *, #108616, .F. ) ;
#23018=ORIENTED_EDGE ( 'NONE', *, *, #36879, .F. ) ;
#23037=ADVANCED_FACE ( 'NONE', ( #134684 ), #111468, .F. ) ;
#23043=( NAMED_UNIT ( * ) SI_UNIT ( $, .STERADIAN. ) SOLID_ANGLE_UNIT ( ) );
#23046=CARTESIAN_POINT ( 'NONE',  ( 3.225639847634963697, -48.88932940808382455, -39.16623080367948972 ) ) ;
#23062=DIRECTION ( 'NONE',  ( 0.000000000000000000, -1.091707662666338270E-16, 1.000000000000000000 ) ) ;
#23064=FILL_AREA_STYLE_COLOUR ( '', #74259 ) ;
#23066=CARTESIAN_POINT ( 'NONE',  ( 26.40000000000000568, -17.48000000000005016, 34.92499999999998295 ) ) ;
#23107=CARTESIAN_POINT ( 'NONE',  ( 18.73373647476854842, 5.808823158059036373, 5.808823158059032821 ) ) ;
#23114=ORIENTED_EDGE ( 'NONE', *, *, #369, .F. ) ;
#23122=CARTESIAN_POINT ( 'NONE',  ( 25.39999999999999858, -18.48000000000005372, 33.92499999999998295 ) ) ;
#23123=AXIS2_PLACEMENT_3D ( 'NONE', #56804, #78517, #135754 ) ;
#23159=CARTESIAN_POINT ( 'NONE',  ( 24.18706980810188867, -2.126176841940956130, 7.934999999999991616 ) ) ;
#23161=CARTESIAN_POINT ( 'NONE',  ( 2.603736474768552966, 5.808823158059035485, 5.808823158059032821 ) ) ;
#23170=VERTEX_POINT ( 'NONE', #20711 ) ;
#23190=LINE ( 'NONE', #24641, #5849 ) ;
#23198=DIRECTION ( 'NONE',  ( 0.000000000000000000, -0.9976538855070753442, -0.06845965770171351383 ) ) ;
#23217=EDGE_LOOP ( 'NONE', ( #78449, #4011, #28326, #18829, #32888, #43917, #111614, #132500, #29513, #29326, #117246, #64612, #89420, #61446, #76501, #105657, #71211, #12917, #15098, #29704, #56676, #86288 ) ) ;
#23221=CARTESIAN_POINT ( 'NONE',  ( 1.087903141435219379, 6.871911579029515771, 3.967499999999989146 ) ) ;
#23240=( NAMED_UNIT ( * ) SI_UNIT ( $, .STERADIAN. ) SOLID_ANGLE_UNIT ( ) );
#23281=CARTESIAN_POINT ( 'NONE',  ( 159.7320121765528711, 26.96999999999993847, -34.92499999999998295 ) ) ;
#23287=AXIS2_PLACEMENT_3D ( 'NONE', #97102, #62402, #73977 ) ;
#23289=CARTESIAN_POINT ( 'NONE',  ( 24.56706980810189123, 2.126176841940952134, -7.934999999999993392 ) ) ;
#23290=FACE_OUTER_BOUND ( 'NONE', #120183, .T. ) ;
#23346=EDGE_LOOP ( 'NONE', ( #117946, #19477, #120978 ) ) ;
#23350=SURFACE_STYLE_USAGE ( .BOTH. , #31395 ) ;
#23356=CARTESIAN_POINT ( 'NONE',  ( 1.494327302228996235, -1.524194347291654372, -6.429405139856394946 ) ) ;
#23366=COLOUR_RGB ( '', 0.72549020, 0.75294118, 0.79215686) ;
#23446=ADVANCED_FACE ( 'NONE', ( #39291 ), #118969, .F. ) ;
#23471=( NAMED_UNIT ( * ) PLANE_ANGLE_UNIT ( ) SI_UNIT ( $, .RADIAN. ) );
#23482=CARTESIAN_POINT ( 'NONE',  ( 32.42080628287043709, 3.047499999999997655, 5.278424836066143655 ) ) ;
#23493=FACE_OUTER_BOUND ( 'NONE', #141649, .T. ) ;
#23516=EDGE_CURVE ( 'NONE', #66688, #40407, #136909, .T. ) ;
#23526=DIRECTION ( 'NONE',  ( 0.000000000000000000, -1.091707662666338270E-16, 1.000000000000000000 ) ) ;
#23557=CARTESIAN_POINT ( 'NONE',  ( 16.08747294953710849, -6.094999999999989981, 3.732111120401553285E-16 ) ) ;
#23573=EDGE_CURVE ( 'NONE', #73841, #65308, #97945, .T. ) ;
#23601=ORIENTED_EDGE ( 'NONE', *, *, #127305, .F. ) ;
#23628=( GEOMETRIC_REPRESENTATION_CONTEXT ( 3 ) GLOBAL_UNCERTAINTY_ASSIGNED_CONTEXT ( ( #14246 ) ) GLOBAL_UNIT_ASSIGNED_CONTEXT ( ( #5974, #84999, #29892 ) ) REPRESENTATION_CONTEXT ( 'NONE', 'WORKASPACE' ) );
#23646=DIRECTION ( 'NONE',  ( 0.000000000000000000, 0.000000000000000000, -1.000000000000000000 ) ) ;
#23658=CARTESIAN_POINT ( 'NONE',  ( 5.733306282870439752, -6.094999999999989981, -1.633150327867689100 ) ) ;
#23661=ORIENTED_EDGE ( 'NONE', *, *, #3010, .F. ) ;
#23663=CARTESIAN_POINT ( 'NONE',  ( 184.1500000000000057, -57.15000000000009095, 34.92499999999998295 ) ) ;
#23681=CARTESIAN_POINT ( 'NONE',  ( 152.4000000000000057, 7.919999999999947526, 16.57229999999999137 ) ) ;
#23686=CARTESIAN_POINT ( 'NONE',  ( 16.74956980810188867, 3.967499999999998916, 6.871911579029510442 ) ) ;
#23696=SURFACE_SIDE_STYLE ('',( #14244 ) ) ;
#23728=DIRECTION ( 'NONE',  ( 0.000000000000000000, -0.000000000000000000, -1.000000000000000000 ) ) ;
#23734=CARTESIAN_POINT ( 'NONE',  ( 10.35416666666666430, 1.633150327867695095, 6.094999999999988205 ) ) ;
#23735=CARTESIAN_POINT ( 'NONE',  ( 23.60373647476854941, 5.808823158059035485, 5.808823158059032821 ) ) ;
#23751=( GEOMETRIC_REPRESENTATION_CONTEXT ( 3 ) GLOBAL_UNCERTAINTY_ASSIGNED_CONTEXT ( ( #54918 ) ) GLOBAL_UNIT_ASSIGNED_CONTEXT ( ( #50873, #60342, #64599 ) ) REPRESENTATION_CONTEXT ( 'NONE', 'WORKASPACE' ) );
#23766=SURFACE_STYLE_USAGE ( .BOTH. , #10706 ) ;
#23790=( GEOMETRIC_REPRESENTATION_CONTEXT ( 3 ) GLOBAL_UNCERTAINTY_ASSIGNED_CONTEXT ( ( #98274 ) ) GLOBAL_UNIT_ASSIGNED_CONTEXT ( ( #2621, #4718, #3328 ) ) REPRESENTATION_CONTEXT ( 'NONE', 'WORKASPACE' ) );
#23798=CARTESIAN_POINT ( 'NONE',  ( 20.62956980810188412, -3.967499999999998028, -6.871911579029511330 ) ) ;
#23806=CARTESIAN_POINT ( 'NONE',  ( 10.35416666666666607, 1.633150327867685103, 6.094999999999992646 ) ) ;
#23816=B_SPLINE_CURVE_WITH_KNOTS ( 'NONE', 3,
 ( #105595, #59994, #92585, #136822 ),
 .UNSPECIFIED., .F., .F.,
 ( 4, 4 ),
 ( 0.000000000000000000, 0.001115544020566860712 ),
 .UNSPECIFIED. ) ;
#23825=ORIENTED_EDGE ( 'NONE', *, *, #38940, .T. ) ;
#23830=VERTEX_POINT ( 'NONE', #135584 ) ;
#23861=CARTESIAN_POINT ( 'NONE',  ( 13.46247294953710494, -7.464222240803106570E-16, -6.094999999999989981 ) ) ;
#23869=CARTESIAN_POINT ( 'NONE',  ( 21.21290314143522338, 3.967499999999992699, -6.871911579029513994 ) ) ;
#23897=( NAMED_UNIT ( * ) SI_UNIT ( $, .STERADIAN. ) SOLID_ANGLE_UNIT ( ) );
#23918=CARTESIAN_POINT ( 'NONE',  ( 21.41623647476855652, -7.934999999999990727, 4.858786175617117713E-16 ) ) ;
#23919=CARTESIAN_POINT ( 'NONE',  ( 0.4162364747685527444, -7.934999999999990727, 4.858786175617117713E-16 ) ) ;
#23970=SURFACE_STYLE_FILL_AREA ( #47892 ) ;
#23987=FILL_AREA_STYLE_COLOUR ( '', #120063 ) ;
#24011=EDGE_CURVE ( 'NONE', #138592, #672, #78340, .T. ) ;
#24014=STYLED_ITEM ( 'NONE', ( #76738 ), #32375 ) ;
#24018=DIRECTION ( 'NONE',  ( -0.000000000000000000, 1.000000000000000000, 0.000000000000000000 ) ) ;
#24033=LINE ( 'NONE', #45111, #34811 ) ;
#24036=CARTESIAN_POINT ( 'NONE',  ( 23.10873647476855552, -5.808823158059033709, 5.808823158059035485 ) ) ;
#24056=CARTESIAN_POINT ( 'NONE',  ( 56.09683561313698874, -51.20434817233912383, 36.87500513592860329 ) ) ;
#24088=ORIENTED_EDGE ( 'NONE', *, *, #82858, .F. ) ;
#24135=ORIENTED_EDGE ( 'NONE', *, *, #102451, .T. ) ;
#24157=FACE_OUTER_BOUND ( 'NONE', #45501, .T. ) ;
#24213=CARTESIAN_POINT ( 'NONE',  ( 3.275403141435220267, -2.126176841940958351, -7.934999999999989839 ) ) ;
#24232=DIRECTION ( 'NONE',  ( -1.000000000000000000, -0.000000000000000000, -0.000000000000000000 ) ) ;
#24244=CARTESIAN_POINT ( 'NONE',  ( -0.1670968585647805704, -3.967499999999994476, 6.871911579029513106 ) ) ;
#24260=VERTEX_POINT ( 'NONE', #107036 ) ;
#24283=STYLED_ITEM ( 'NONE', ( #106285 ), #90553 ) ;
#24296=SURFACE_SIDE_STYLE ('',( #79446 ) ) ;
#24307=( GEOMETRIC_REPRESENTATION_CONTEXT ( 3 ) GLOBAL_UNCERTAINTY_ASSIGNED_CONTEXT ( ( #37444 ) ) GLOBAL_UNIT_ASSIGNED_CONTEXT ( ( #33711, #79382, #122838 ) ) REPRESENTATION_CONTEXT ( 'NONE', 'WORKASPACE' ) );
#24308=ORIENTED_EDGE ( 'NONE', *, *, #105117, .T. ) ;
#24352=FILL_AREA_STYLE_COLOUR ( '', #82855 ) ;
#24370=CARTESIAN_POINT ( 'NONE',  ( 6.170806282870438864, -3.047499999999997211, -5.278424836066143655 ) ) ;
#24374=( GEOMETRIC_REPRESENTATION_CONTEXT ( 3 ) GLOBAL_UNCERTAINTY_ASSIGNED_CONTEXT ( ( #133064 ) ) GLOBAL_UNIT_ASSIGNED_CONTEXT ( ( #114168, #125045, #125781 ) ) REPRESENTATION_CONTEXT ( 'NONE', 'WORKASPACE' ) );
#24398=CARTESIAN_POINT ( 'NONE',  ( 26.22873647476855652, 5.808823158059031044, -5.808823158059038150 ) ) ;
#24408=( NAMED_UNIT ( * ) SI_UNIT ( $, .STERADIAN. ) SOLID_ANGLE_UNIT ( ) );
#24410=UNCERTAINTY_MEASURE_WITH_UNIT (LENGTH_MEASURE( 1.000000000000000082E-05 ), #34609, 'distance_accuracy_value', 'NONE');
#24419=LINE ( 'NONE', #68665, #62951 ) ;
#24443=CARTESIAN_POINT ( 'NONE',  ( 15.31250000000000000, -4.461849672132299993, -4.461849672132299105 ) ) ;
#24444=CARTESIAN_POINT ( 'NONE',  ( 25.06206980810188512, -7.934999999999990727, -2.126176841940955242 ) ) ;
#24455=CARTESIAN_POINT ( 'NONE',  ( 126.6671759105392567, -47.13357697190492246, -36.34567044387053869 ) ) ;
#24482=CARTESIAN_POINT ( 'NONE',  ( 25.39999999999999858, 0.000000000000000000, 6.094999999999989093 ) ) ;
#24495=DIRECTION ( 'NONE',  ( 0.000000000000000000, 0.000000000000000000, 1.000000000000000000 ) ) ;
#24508=( GEOMETRIC_REPRESENTATION_CONTEXT ( 3 ) GLOBAL_UNCERTAINTY_ASSIGNED_CONTEXT ( ( #24598 ) ) GLOBAL_UNIT_ASSIGNED_CONTEXT ( ( #71202, #7322, #127716 ) ) REPRESENTATION_CONTEXT ( 'NONE', 'WORKASPACE' ) );
#24568=CARTESIAN_POINT ( 'NONE',  ( 32.44206980810188412, 7.934999999999993392, 2.126176841940951689 ) ) ;
#24598=UNCERTAINTY_MEASURE_WITH_UNIT (LENGTH_MEASURE( 1.000000000000000082E-05 ), #71202, 'distance_accuracy_value', 'NONE');
#24612=CARTESIAN_POINT ( 'NONE',  ( 22.29123647476855652, -9.717572351234235426E-16, -7.934999999999990727 ) ) ;
#24613=CARTESIAN_POINT ( 'NONE',  ( 1.145403141435219263, -2.126176841940958351, -7.934999999999988951 ) ) ;
#24619=EDGE_LOOP ( 'NONE', ( #35962, #66651, #131137, #587 ) ) ;
#24641=CARTESIAN_POINT ( 'NONE',  ( 0.000000000000000000, -14.29000000000013593, 12.69999999999954632 ) ) ;
#24649=( GEOMETRIC_REPRESENTATION_CONTEXT ( 3 ) GLOBAL_UNCERTAINTY_ASSIGNED_CONTEXT ( ( #47480 ) ) GLOBAL_UNIT_ASSIGNED_CONTEXT ( ( #9837, #92205, #132378 ) ) REPRESENTATION_CONTEXT ( 'NONE', 'WORKASPACE' ) );
#24663=ORIENTED_EDGE ( 'NONE', *, *, #142448, .F. ) ;
#24665=CARTESIAN_POINT ( 'NONE',  ( 0.9420698081018860082, 7.934999999999992504, 2.126176841940951689 ) ) ;
#24670=AXIS2_PLACEMENT_3D ( 'NONE', #35422, #34680, #24495 ) ;
#24682=VERTEX_POINT ( 'NONE', #6088 ) ;
#24687=FACE_BOUND ( 'NONE', #54559, .T. ) ;
#24692=CARTESIAN_POINT ( 'NONE',  ( 184.1500000000000057, -43.14999999999999147, 40.92499999999998295 ) ) ;
#24693=CARTESIAN_POINT ( 'NONE',  ( 3.730677800976791136, -52.14999999999999147, 40.92499999999998295 ) ) ;
#24736=CARTESIAN_POINT ( 'NONE',  ( 26.17123647476855908, 0.000000000000000000, 7.934999999999990727 ) ) ;
#24790=CARTESIAN_POINT ( 'NONE',  ( 0.2168868938212059061, -7.334364015408722182, 2.940725648025187766 ) ) ;
#24835=EDGE_CURVE ( 'NONE', #98296, #5341, #143070, .T. ) ;
#24842=CARTESIAN_POINT ( 'NONE',  ( 0.000000000000000000, 9.913515839097813477E-16, -8.094999999999991758 ) ) ;
#24879=CIRCLE ( 'NONE', #98963, 9.000000000000001776 ) ;
#24893=AXIS2_PLACEMENT_3D ( 'NONE', #68112, #135481, #114414 ) ;
#24906=CARTESIAN_POINT ( 'NONE',  ( 0.3587364747685527488, 5.808823158059031044, -5.808823158059038150 ) ) ;
#24933=CARTESIAN_POINT ( 'NONE',  ( 52.26932219902319332, -49.14999999999999147, -40.92499999999998295 ) ) ;
#24993=CARTESIAN_POINT ( 'NONE',  ( 55.56056557994608625, -52.00875322212550600, 39.86617647058822200 ) ) ;
#25041=ORIENTED_EDGE ( 'NONE', *, *, #45473, .F. ) ;
#25050=CARTESIAN_POINT ( 'NONE',  ( 25.40000000000000568, 7.872929591417200612, 1.072287140687521179 ) ) ;
#25063=CARTESIAN_POINT ( 'NONE',  ( 2.670806282870439308, -3.047499999999997211, -5.278424836066143655 ) ) ;
#25074=FILL_AREA_STYLE_COLOUR ( '', #32882 ) ;
#25094=VECTOR ( 'NONE', #37023, 1000.000000000000000 ) ;
#25097=CARTESIAN_POINT ( 'NONE',  ( 25.06206980810188512, -7.934999999999991616, -2.126176841940955242 ) ) ;
#25104=DIRECTION ( 'NONE',  ( 0.000000000000000000, 0.000000000000000000, -1.000000000000000000 ) ) ;
#25110=STYLED_ITEM ( 'NONE', ( #99861 ), #95688 ) ;
#25111=CARTESIAN_POINT ( 'NONE',  ( 152.4000000000000057, 7.919999999999947526, -16.42230000000006029 ) ) ;
#25117=VECTOR ( 'NONE', #28907, 1000.000000000000000 ) ;
#25126=CARTESIAN_POINT ( 'NONE',  ( 2.999999999999999112, -43.14999999999999147, 40.92499999999998295 ) ) ;
#25139=FACE_OUTER_BOUND ( 'NONE', #102674, .T. ) ;
#25147=CARTESIAN_POINT ( 'NONE',  ( 21.87500000000000355, -6.094999999999989981, 3.732111120401553285E-16 ) ) ;
#25148=CARTESIAN_POINT ( 'NONE',  ( 25.20790314143522082, -6.871911579029513106, -3.967499999999993587 ) ) ;
#25192=EDGE_LOOP ( 'NONE', ( #34503, #42118, #95635, #37396 ) ) ;
#25197=COLOUR_RGB ( '', 0.40784314, 0.44705882, 0.49803922) ;
#25205=CARTESIAN_POINT ( 'NONE',  ( 25.39999999999999858, 7.796566843815467607, 1.475727091950665537 ) ) ;
#25215=CARTESIAN_POINT ( 'NONE',  ( 10.06250000000000000, 4.461849672132300881, 4.461849672132299105 ) ) ;
#25275=CARTESIAN_POINT ( 'NONE',  ( 28.35873647476855197, 5.808823158059031044, -5.808823158059038150 ) ) ;
#25298=CARTESIAN_POINT ( 'NONE',  ( 57.17148983090720549, -47.44491123044907965, -36.62621018406388629 ) ) ;
#25304=DIRECTION ( 'NONE',  ( -0.000000000000000000, 0.000000000000000000, 1.000000000000000000 ) ) ;
#25310=DIRECTION ( 'NONE',  ( 0.000000000000000000, 1.000000000000000000, 0.000000000000000000 ) ) ;
#25317=CARTESIAN_POINT ( 'NONE',  ( 22.14540314143522082, -2.126176841940958351, -7.934999999999989839 ) ) ;
#25338=DIRECTION ( 'NONE',  ( -1.000000000000000000, -0.000000000000000000, -0.000000000000000000 ) ) ;
#25374=FACE_OUTER_BOUND ( 'NONE', #3713, .T. ) ;
#25390=SURFACE_STYLE_USAGE ( .BOTH. , #68945 ) ;
#25407=FACE_OUTER_BOUND ( 'NONE', #11467, .T. ) ;
#25426=ORIENTED_EDGE ( 'NONE', *, *, #78762, .T. ) ;
#25428=ORIENTED_EDGE ( 'NONE', *, *, #96776, .T. ) ;
#25439=CARTESIAN_POINT ( 'NONE',  ( 33.17123647476855552, 0.000000000000000000, 7.934999999999990727 ) ) ;
#25440=CARTESIAN_POINT ( 'NONE',  ( 2.983736474768552860, -5.808823158059035485, -5.808823158059033709 ) ) ;
#25454=CARTESIAN_POINT ( 'NONE',  ( 183.4386084925502303, -49.19295221410152408, -41.21232802153173225 ) ) ;
#25469=DIRECTION ( 'NONE',  ( 0.000000000000000000, -1.000000000000000000, 0.000000000000000000 ) ) ;
#25473=FACE_OUTER_BOUND ( 'NONE', #14063, .T. ) ;
#25498=( GEOMETRIC_REPRESENTATION_CONTEXT ( 3 ) GLOBAL_UNCERTAINTY_ASSIGNED_CONTEXT ( ( #118579 ) ) GLOBAL_UNIT_ASSIGNED_CONTEXT ( ( #90180, #66318, #57592 ) ) REPRESENTATION_CONTEXT ( 'NONE', 'WORKASPACE' ) );
#25513=CARTESIAN_POINT ( 'NONE',  ( 1.153023801772934176, 3.242423929075685329, 6.152118276231695937 ) ) ;
#25529=ORIENTED_EDGE ( 'NONE', *, *, #111780, .T. ) ;
#25532=CARTESIAN_POINT ( 'NONE',  ( 26.40000000000000568, -18.48000000000005372, -34.92499999999998295 ) ) ;
#25577=CARTESIAN_POINT ( 'NONE',  ( 25.39999999999999858, 0.000000000000000000, 0.000000000000000000 ) ) ;
#25603=VECTOR ( 'NONE', #118238, 1000.000000000000000 ) ;
#25617=CARTESIAN_POINT ( 'NONE',  ( 30.67080628287044419, -3.047499999999997211, -5.278424836066143655 ) ) ;
#25646=CARTESIAN_POINT ( 'NONE',  ( 6.754139616203771901, 3.047499999999993214, -5.278424836066146320 ) ) ;
#25649=VERTEX_POINT ( 'NONE', #10427 ) ;
#25650=VECTOR ( 'NONE', #1035, 1000.000000000000000 ) ;
#25655=CARTESIAN_POINT ( 'NONE',  ( 8.291236474768552966, -9.717572351234235426E-16, -7.934999999999990727 ) ) ;
#25663=STYLED_ITEM ( 'NONE', ( #79620 ), #23037 ) ;
#25682=CARTESIAN_POINT ( 'NONE',  ( 11.37500000000000178, -6.094999999999989981, 3.732111120401553285E-16 ) ) ;
#25686=CARTESIAN_POINT ( 'NONE',  ( 28.00000000000002487, -49.14999999999999147, 34.92500000000003268 ) ) ;
#25763=CARTESIAN_POINT ( 'NONE',  ( 18.95833333333333570, -3.047499999999997211, -5.278424836066143655 ) ) ;
#25776=EDGE_LOOP ( 'NONE', ( #20644, #13038, #97053, #52202 ) ) ;
#25790=CARTESIAN_POINT ( 'NONE',  ( 9.524972949537108491, -4.461849672132299993, -4.461849672132299105 ) ) ;
#25799=ORIENTED_EDGE ( 'NONE', *, *, #57998, .T. ) ;
#25818=SURFACE_SIDE_STYLE ('',( #102686 ) ) ;
#25823=EDGE_CURVE ( 'NONE', #48102, #90432, #36484, .T. ) ;
#25825=CARTESIAN_POINT ( 'NONE',  ( 23.60373647476854941, 5.808823158059036373, 5.808823158059032821 ) ) ;
#25835=UNCERTAINTY_MEASURE_WITH_UNIT (LENGTH_MEASURE( 1.000000000000000082E-05 ), #68450, 'distance_accuracy_value', 'NONE');
#25840=COLOUR_RGB ( '', 0.08235294, 0.09019608, 0.10196078) ;
#25875=CARTESIAN_POINT ( 'NONE',  ( 24.50000000000000000, 0.000000000000000000, 6.094999999999989981 ) ) ;
#25877=CARTESIAN_POINT ( 'NONE',  ( 23.74956980810188867, 3.967499999999998916, 6.871911579029510442 ) ) ;
#25891=CARTESIAN_POINT ( 'NONE',  ( 127.5247579190697991, -47.99115898043766748, -37.22402166429520776 ) ) ;
#25939=SURFACE_SIDE_STYLE ('',( #123841 ) ) ;
#25942=( NAMED_UNIT ( * ) PLANE_ANGLE_UNIT ( ) SI_UNIT ( $, .RADIAN. ) );
#25947=CARTESIAN_POINT ( 'NONE',  ( 9.479166666666667851, 6.094999999999988205, -1.633150327867694651 ) ) ;
#25952=EDGE_LOOP ( 'NONE', ( #910, #48842, #79667, #134857 ) ) ;
#25975=ADVANCED_FACE ( 'NONE', ( #52345 ), #29867, .F. ) ;
#26005=SURFACE_SIDE_STYLE ('',( #93393 ) ) ;
#26010=CARTESIAN_POINT ( 'NONE',  ( 31.85873647476855552, 5.808823158059031044, -5.808823158059038150 ) ) ;
#26032=COLOUR_RGB ( '', 0.40784314, 0.44705882, 0.49803922) ;
#26055=CARTESIAN_POINT ( 'NONE',  ( 26.52040314143521726, 7.934999999999989839, -2.126176841940961904 ) ) ;
#26070=( GEOMETRIC_REPRESENTATION_CONTEXT ( 3 ) GLOBAL_UNCERTAINTY_ASSIGNED_CONTEXT ( ( #2461 ) ) GLOBAL_UNIT_ASSIGNED_CONTEXT ( ( #59794, #44099, #110729 ) ) REPRESENTATION_CONTEXT ( 'NONE', 'WORKASPACE' ) );
#26088=CARTESIAN_POINT ( 'NONE',  ( 55.71344734891374628, -51.77943056867389515, 39.18578444878559708 ) ) ;
#26115=DIRECTION ( 'NONE',  ( 0.000000000000000000, 0.000000000000000000, 1.000000000000000000 ) ) ;
#26128=( GEOMETRIC_REPRESENTATION_CONTEXT ( 3 ) GLOBAL_UNCERTAINTY_ASSIGNED_CONTEXT ( ( #34583 ) ) GLOBAL_UNIT_ASSIGNED_CONTEXT ( ( #71296, #14013, #48111 ) ) REPRESENTATION_CONTEXT ( 'NONE', 'WORKASPACE' ) );
#26183=CARTESIAN_POINT ( 'NONE',  ( 1.817069808101886341, -2.126176841940956130, 7.934999999999991616 ) ) ;
#26184=ORIENTED_EDGE ( 'NONE', *, *, #66179, .F. ) ;
#26205=MECHANICAL_DESIGN_GEOMETRIC_PRESENTATION_REPRESENTATION('',(#88724),#54072);
#26223=FILL_AREA_STYLE ('',( #13877 ) ) ;
#26226=CARTESIAN_POINT ( 'NONE',  ( 27.99999999999999645, -57.14999999999999147, -49.92499999999968452 ) ) ;
#26238=CYLINDRICAL_SURFACE ( 'NONE', #119628, 28.00000000000003197 ) ;
#26252=CARTESIAN_POINT ( 'NONE',  ( 0.8414140276721195910, 6.733540184995763234, 2.728539860749207513 ) ) ;
#26277=ORIENTED_EDGE ( 'NONE', *, *, #95567, .F. ) ;
#26303=DIRECTION ( 'NONE',  ( 0.000000000000000000, -1.000000000000000000, 0.000000000000000000 ) ) ;
#26335=CARTESIAN_POINT ( 'NONE',  ( 16.47916666666667140, 6.094999999999988205, -1.633150327867694651 ) ) ;
#26353=CARTESIAN_POINT ( 'NONE',  ( 9.108736474768550195, -5.808823158059033709, 5.808823158059035485 ) ) ;
#26361=ORIENTED_EDGE ( 'NONE', *, *, #92566, .T. ) ;
#26392=CARTESIAN_POINT ( 'NONE',  ( 3.041236474768552966, 0.000000000000000000, 7.934999999999990727 ) ) ;
#26399=FILL_AREA_STYLE_COLOUR ( '', #136796 ) ;
#26401=CIRCLE ( 'NONE', #95820, 0.9999999999999997780 ) ;
#26402=SURFACE_STYLE_FILL_AREA ( #70648 ) ;
#26416=CARTESIAN_POINT ( 'NONE',  ( 128.8635666761377934, -49.19207878844991200, 41.22112633375493829 ) ) ;
#26442=DIRECTION ( 'NONE',  ( 0.000000000000000000, -1.000000000000000000, 0.000000000000000000 ) ) ;
#26452=DIRECTION ( 'NONE',  ( -1.000000000000000000, -0.000000000000000000, -0.000000000000000000 ) ) ;
#26516=CARTESIAN_POINT ( 'NONE',  ( 12.87913961620377279, -5.278424836066145431, -3.047499999999993658 ) ) ;
#26548=CARTESIAN_POINT ( 'NONE',  ( 23.16623647476855652, 7.934999999999990727, -1.457635852685135314E-15 ) ) ;
#26561=FILL_AREA_STYLE_COLOUR ( '', #133829 ) ;
#26589=EDGE_LOOP ( 'NONE', ( #67349, #27245, #134217, #75892 ) ) ;
#26595=CARTESIAN_POINT ( 'NONE',  ( 26.39583333333333925, 1.633150327867687324, -6.094999999999991758 ) ) ;
#26616=SURFACE_SIDE_STYLE ('',( #70859 ) ) ;
#26646=PRESENTATION_STYLE_ASSIGNMENT (( #135436 ) ) ;
#26662=DIRECTION ( 'NONE',  ( 0.000000000000000000, 1.000000000000000000, -0.000000000000000000 ) ) ;
#26680=MECHANICAL_DESIGN_GEOMETRIC_PRESENTATION_REPRESENTATION('',(#10518),#33644);
#26683=VECTOR ( 'NONE', #33165, 1000.000000000000000 ) ;
#26712=CARTESIAN_POINT ( 'NONE',  ( 24.85873647476855908, 5.808823158059031044, -5.808823158059038150 ) ) ;
#26733=VERTEX_POINT ( 'NONE', #75045 ) ;
#26736=CARTESIAN_POINT ( 'NONE',  ( 59.37656097284387613, -44.54322672568201114, -35.04755940938199643 ) ) ;
#26755=CARTESIAN_POINT ( 'NONE',  ( 26.95790314143522437, 6.871911579029515771, 3.967499999999989146 ) ) ;
#26756=CARTESIAN_POINT ( 'NONE',  ( 10.77040314143521904, -7.934999999999988951, 2.126176841940957907 ) ) ;
#26757=CARTESIAN_POINT ( 'NONE',  ( 15.35830628287044064, -1.633150327867690210, 6.094999999999989981 ) ) ;
#26776=EDGE_CURVE ( 'NONE', #140063, #51562, #120332, .T. ) ;
#26779=SURFACE_STYLE_USAGE ( .BOTH. , #28220 ) ;
#26782=LINE ( 'NONE', #71032, #6246 ) ;
#26811=CARTESIAN_POINT ( 'NONE',  ( 9.983736474768551972, -5.808823158059035485, -5.808823158059033709 ) ) ;
#26827=EDGE_CURVE ( 'NONE', #99786, #68141, #143294, .T. ) ;
#26834=VERTEX_POINT ( 'NONE', #77874 ) ;
#26843=CIRCLE ( 'NONE', #82439, 28.00000000000002487 ) ;
#26856=CARTESIAN_POINT ( 'NONE',  ( 52.26932219902325727, -49.14999999999999147, 40.92499999999998295 ) ) ;
#26860=( GEOMETRIC_REPRESENTATION_CONTEXT ( 3 ) GLOBAL_UNCERTAINTY_ASSIGNED_CONTEXT ( ( #36211 ) ) GLOBAL_UNIT_ASSIGNED_CONTEXT ( ( #137323, #136578, #14810 ) ) REPRESENTATION_CONTEXT ( 'NONE', 'WORKASPACE' ) );
#26865=FILL_AREA_STYLE ('',( #4327 ) ) ;
#26876=CARTESIAN_POINT ( 'NONE',  ( 25.39999999999999858, 1.399999999999987699, -20.40202195861970580 ) ) ;
#26880=CARTESIAN_POINT ( 'NONE',  ( -0.6620968585647807325, -6.871911579029513106, -3.967499999999993587 ) ) ;
#26885=CARTESIAN_POINT ( 'NONE',  ( 55.47138350052868105, -49.14501756083436135, -40.36361034346621324 ) ) ;
#26893=CIRCLE ( 'NONE', #124178, 1.000000000000000000 ) ;
#26897=CARTESIAN_POINT ( 'NONE',  ( 183.6687791239651517, -49.11951764991120939, -40.13200514437819066 ) ) ;
#26901=EDGE_CURVE ( 'NONE', #122655, #119924, #111136, .T. ) ;
#26915=LINE ( 'NONE', #17456, #113667 ) ;
#26916=DIRECTION ( 'NONE',  ( 0.000000000000000000, 5.559056632600921604E-15, -1.000000000000000000 ) ) ;
#26922=PRESENTATION_STYLE_ASSIGNMENT (( #82749 ) ) ;
#26936=SURFACE_STYLE_FILL_AREA ( #105211 ) ;
#26967=SURFACE_STYLE_USAGE ( .BOTH. , #116111 ) ;
#27013=DIRECTION ( 'NONE',  ( 0.000000000000000000, -3.469446951953615372E-15, 1.000000000000000000 ) ) ;
#27028=EDGE_CURVE ( 'NONE', #142647, #67143, #93025, .T. ) ;
#27050=CARTESIAN_POINT ( 'NONE',  ( 6.046236474768552860, -7.934999999999990727, 4.858786175617117713E-16 ) ) ;
#27055=CARTESIAN_POINT ( 'NONE',  ( 24.93750000000000000, -4.461849672132299105, 4.461849672132299993 ) ) ;
#27058=CARTESIAN_POINT ( 'NONE',  ( 10.25413961620377457, 3.047499999999993214, -5.278424836066146320 ) ) ;
#27072=CARTESIAN_POINT ( 'NONE',  ( 20.75413961620377279, 3.047499999999993214, -5.278424836066146320 ) ) ;
#27075=SURFACE_STYLE_USAGE ( .BOTH. , #93772 ) ;
#27083=CARTESIAN_POINT ( 'NONE',  ( 0.7079031414352194851, -6.871911579029513106, -3.967499999999993587 ) ) ;
#27099=FILL_AREA_STYLE ('',( #14071 ) ) ;
#27107=CARTESIAN_POINT ( 'NONE',  ( 128.6956467655707854, -52.10358567239623540, 40.45860062937848767 ) ) ;
#27111=UNCERTAINTY_MEASURE_WITH_UNIT (LENGTH_MEASURE( 1.000000000000000082E-05 ), #49107, 'distance_accuracy_value', 'NONE');
#27117=EDGE_CURVE ( 'NONE', #75508, #104180, #29188, .T. ) ;
#27129=EDGE_LOOP ( 'NONE', ( #31397, #79534, #21667, #69449 ) ) ;
#27131=( BOUNDED_SURFACE ( )  B_SPLINE_SURFACE ( 3, 2, ( 
 ( #135519, #123226, #68159 ),
 ( #2835, #112332, #47129 ),
 ( #47817, #59403, #26736 ),
 ( #115134, #12984, #57261 ),
 ( #134823, #35519, #79751 ),
 ( #91313, #36202, #80431 ),
 ( #124623, #25298, #69564 ),
 ( #82552, #129609, #63679 ),
 ( #96242, #117988, #62967 ),
 ( #83268, #7820, #118735 ),
 ( #93427, #60847, #41175 ),
 ( #85385, #39788, #28173 ),
 ( #84014, #94119, #19428 ),
 ( #72435, #61547, #18691 ),
 ( #140484, #138360, #107839 ),
 ( #38336, #8504, #107144 ) ),
 .UNSPECIFIED., .F., .F., .F. ) 
 B_SPLINE_SURFACE_WITH_KNOTS ( ( 4, 2, 2, 2, 2, 2, 2, 4 ),
 ( 3, 3 ),
 ( 4.712388980384689674, 5.060738160973319744, 5.234912751267634334, 5.409087341561949813, 5.583261931856265292, 5.757436522150579883, 5.931611112444894474, 6.105785702739209952 ),
 ( 0.000000000000000000, 1.000000000000000000 ),
 .UNSPECIFIED. ) 
 GEOMETRIC_REPRESENTATION_ITEM ( )  RATIONAL_B_SPLINE_SURFACE ( (
 ( 1.000000000000000000, 1.000000000000000000, 1.000000000000000000),
 ( 1.000000000000000000, 1.000097732991066080, 1.000000000000000000),
 ( 1.000000000000000000, 0.9896287210066593287, 1.000000000000000000),
 ( 1.000000000000000000, 0.9608359430471657969, 1.000000000000000000),
 ( 1.000000000000000000, 0.9490805577171574914, 1.000000000000000000),
 ( 1.000000000000000000, 0.9222453908327415961, 1.000000000000000000),
 ( 1.000000000000000000, 0.9071649184813681543, 1.000000000000000000),
 ( 1.000000000000000000, 0.8751006588766465644, 1.000000000000000000),
 ( 1.000000000000000000, 0.8581174656085591712, 1.000000000000000000),
 ( 1.000000000000000000, 0.8241077986061765559, 1.000000000000000000),
 ( 1.000000000000000000, 0.8070860741947217809, 1.000000000000000000),
 ( 1.000000000000000000, 0.7752313834060545750, 1.000000000000000000),
 ( 1.000000000000000000, 0.7604116155351108297, 1.000000000000000000),
 ( 1.000000000000000000, 0.7353122387368615787, 1.000000000000000000),
 ( 1.000000000000000000, 0.7250426641248349791, 1.000000000000000000),
 ( 1.000000000000000000, 0.7180326832784534874, 1.000000000000000000) ) ) 
 REPRESENTATION_ITEM ( '' )  SURFACE ( )  );
#27158=FILL_AREA_STYLE ('',( #82288 ) ) ;
#27171=MECHANICAL_DESIGN_GEOMETRIC_PRESENTATION_REPRESENTATION('',(#89683),#124455);
#27177=AXIS2_PLACEMENT_3D ( 'NONE', #143443, #118841, #85483 ) ;
#27178=CIRCLE ( 'NONE', #135948, 2.999999999999999112 ) ;
#27184=ORIENTED_EDGE ( 'NONE', *, *, #63475, .T. ) ;
#27198=CARTESIAN_POINT ( 'NONE',  ( 181.0878408821075141, -48.47815212813053165, -38.14157743968407033 ) ) ;
#27210=VECTOR ( 'NONE', #22419, 1000.000000000000000 ) ;
#27211=CARTESIAN_POINT ( 'NONE',  ( 16.81663961620377634, -1.633150327867691987, -6.094999999999989093 ) ) ;
#27216=FACE_OUTER_BOUND ( 'NONE', #124598, .T. ) ;
#27226=EDGE_CURVE ( 'NONE', #19025, #9588, #24033, .T. ) ;
#27239=CARTESIAN_POINT ( 'NONE',  ( 18.93706980810188867, 2.126176841940952134, -7.934999999999993392 ) ) ;
#27242=( GEOMETRIC_REPRESENTATION_CONTEXT ( 3 ) GLOBAL_UNCERTAINTY_ASSIGNED_CONTEXT ( ( #60498 ) ) GLOBAL_UNIT_ASSIGNED_CONTEXT ( ( #69301, #112096, #3966 ) ) REPRESENTATION_CONTEXT ( 'NONE', 'WORKASPACE' ) );
#27245=ORIENTED_EDGE ( 'NONE', *, *, #65035, .T. ) ;
#27281=( NAMED_UNIT ( * ) PLANE_ANGLE_UNIT ( ) SI_UNIT ( $, .RADIAN. ) );
#27286=CARTESIAN_POINT ( 'NONE',  ( 23.18750000000000355, 4.461849672132297329, -4.461849672132302658 ) ) ;
#27307=CARTESIAN_POINT ( 'NONE',  ( 12.25000000000000000, -7.464222240803106570E-16, -6.094999999999989981 ) ) ;
#27340=CARTESIAN_POINT ( 'NONE',  ( 149.2199999999997999, -3.180000000000061444, -34.92499999999998295 ) ) ;
#27373=CARTESIAN_POINT ( 'NONE',  ( 27.99999999999999645, -49.14999999999999147, -45.92499999999969873 ) ) ;
#27379=VECTOR ( 'NONE', #77746, 1000.000000000000000 ) ;
#27384=AXIS2_PLACEMENT_3D ( 'NONE', #57104, #112185, #78128 ) ;
#27387=ORIENTED_EDGE ( 'NONE', *, *, #66984, .F. ) ;
#27400=( NAMED_UNIT ( * ) SI_UNIT ( $, .STERADIAN. ) SOLID_ANGLE_UNIT ( ) );
#27403=CARTESIAN_POINT ( 'NONE',  ( 24.12956980810188767, -3.967499999999998028, -6.871911579029511330 ) ) ;
#27409=B_SPLINE_CURVE_WITH_KNOTS ( 'NONE', 3,
 ( #76781, #9295, #142719, #87623, #45583, #78188, #53579, #12192, #97782, #55727, #99930, #42718, #21660, #122371, #592, #44891, #131132, #131853, #109370, #120208 ),
 .UNSPECIFIED., .F., .F.,
 ( 4, 2, 2, 2, 2, 2, 2, 2, 2, 4 ),
 ( 0.000000000000000000, 0.002083055955866117918, 0.003124583933799176226, 0.004166111911732234101, 0.005207639889665291975, 0.006249167867598350717, 0.006769931856564878787, 0.007290695845531407725, 0.007811459834497935795, 0.008332223823464464732 ),
 .UNSPECIFIED. ) ;
#27447=CARTESIAN_POINT ( 'NONE',  ( 34.10373647476854586, 5.808823158059036373, 5.808823158059032821 ) ) ;
#27448=CARTESIAN_POINT ( 'NONE',  ( 10.91623647476855297, -7.934999999999990727, 4.858786175617117713E-16 ) ) ;
#27457=CARTESIAN_POINT ( 'NONE',  ( 122.6835989386367345, -43.14999999999999147, 34.92499999999998295 ) ) ;
#27475=PRESENTATION_STYLE_ASSIGNMENT (( #26779 ) ) ;
#27509=CARTESIAN_POINT ( 'NONE',  ( 8.379569808101887674, 3.967499999999998916, 6.871911579029510442 ) ) ;
#27529=FILL_AREA_STYLE_COLOUR ( '', #25840 ) ;
#27545=SURFACE_STYLE_USAGE ( .BOTH. , #81262 ) ;
#27582=CARTESIAN_POINT ( 'NONE',  ( -0.2245968585647807325, -2.126176841940958351, -7.934999999999989839 ) ) ;
#27593=CIRCLE ( 'NONE', #85537, 5.999999999999998224 ) ;
#27595=FACE_OUTER_BOUND ( 'NONE', #32719, .T. ) ;
#27598=PRESENTATION_STYLE_ASSIGNMENT (( #58878 ) ) ;
#27621=MECHANICAL_DESIGN_GEOMETRIC_PRESENTATION_REPRESENTATION('',(#134140),#48434);
#27642=( NAMED_UNIT ( * ) SI_UNIT ( $, .STERADIAN. ) SOLID_ANGLE_UNIT ( ) );
#27656=FILL_AREA_STYLE ('',( #93651 ) ) ;
#27662=FILL_AREA_STYLE ('',( #5887 ) ) ;
#27680=AXIS2_PLACEMENT_3D ( 'NONE', #55766, #131164, #130471 ) ;
#27710=AXIS2_PLACEMENT_3D ( 'NONE', #15335, #71206, #59622 ) ;
#27714=CARTESIAN_POINT ( 'NONE',  ( 2.999999999999999112, -43.14999999999999147, -40.92499999999998295 ) ) ;
#27765=CARTESIAN_POINT ( 'NONE',  ( 11.87956980810188767, 3.967499999999998916, 6.871911579029510442 ) ) ;
#27778=CARTESIAN_POINT ( 'NONE',  ( 28.00000000000002487, -57.14999999999999147, -34.92499999999976978 ) ) ;
#27789=COLOUR_RGB ( '', 0.40784314, 0.44705882, 0.49803922) ;
#27794=ADVANCED_FACE ( 'NONE', ( #81114 ), #135493, .F. ) ;
#27802=CARTESIAN_POINT ( 'NONE',  ( 3.332903141435219929, -3.967499999999994476, 6.871911579029513106 ) ) ;
#27813=DIRECTION ( 'NONE',  ( 0.000000000000000000, 1.000000000000000000, -4.625929269271485322E-15 ) ) ;
#27829=CARTESIAN_POINT ( 'NONE',  ( 12.10416666666666785, -1.633150327867681995, -6.094999999999993534 ) ) ;
#27870=ORIENTED_EDGE ( 'NONE', *, *, #109684, .F. ) ;
#27895=AXIS2_PLACEMENT_3D ( 'NONE', #33160, #22213, #77371 ) ;
#27897=EDGE_CURVE ( 'NONE', #42914, #5341, #94092, .T. ) ;
#27925=ADVANCED_FACE ( 'NONE', ( #51332 ), #1819, .T. ) ;
#27938=CARTESIAN_POINT ( 'NONE',  ( 11.27497294953710671, 4.461849672132300881, 4.461849672132299105 ) ) ;
#27951=ORIENTED_EDGE ( 'NONE', *, *, #64635, .F. ) ;
#27975=CARTESIAN_POINT ( 'NONE',  ( 28.99956980810188867, -3.967499999999998028, -6.871911579029511330 ) ) ;
#27987=CARTESIAN_POINT ( 'NONE',  ( 0.01167931549069694576, -50.55966373067267483, -35.89041033429499095 ) ) ;
#28016=EDGE_CURVE ( 'NONE', #93928, #68985, #138626, .T. ) ;
#28025=CARTESIAN_POINT ( 'NONE',  ( 24.35416666666666785, 1.633150327867695095, 6.094999999999988205 ) ) ;
#28038=DIRECTION ( 'NONE',  ( 0.000000000000000000, 0.000000000000000000, 1.000000000000000000 ) ) ;
#28148=CARTESIAN_POINT ( 'NONE',  ( 4.353736474768552966, -5.808823158059035485, -5.808823158059033709 ) ) ;
#28154=VECTOR ( 'NONE', #53745, 1000.000000000000000 ) ;
#28156=LINE ( 'NONE', #127455, #107418 ) ;
#28165=CARTESIAN_POINT ( 'NONE',  ( 3.000000000000000000, -47.62213595499959951, 36.92500000000000426 ) ) ;
#28167=DIRECTION ( 'NONE',  ( 0.000000000000000000, 0.6666666666666631880, -0.7453559924999331177 ) ) ;
#28173=CARTESIAN_POINT ( 'NONE',  ( 53.41963127661841781, -48.51451318982912397, -38.21513923099966092 ) ) ;
#28192=CARTESIAN_POINT ( 'NONE',  ( 29.87456980810189222, 6.871911579029510442, -3.967499999999998916 ) ) ;
#28193=CARTESIAN_POINT ( 'NONE',  ( 10.33290314143522082, -3.967499999999994476, 6.871911579029513106 ) ) ;
#28206=CARTESIAN_POINT ( 'NONE',  ( 22.94163961620376924, -6.094999999999989093, 1.633150327867691542 ) ) ;
#28216=CARTESIAN_POINT ( 'NONE',  ( 55.32809448528696095, -52.14999999999999147, -41.05261164187028555 ) ) ;
#28220=SURFACE_SIDE_STYLE ('',( #17327 ) ) ;
#28225=CARTESIAN_POINT ( 'NONE',  ( 55.86145213702157264, -48.75494892434544880, 38.51155878621108286 ) ) ;
#28230=CARTESIAN_POINT ( 'NONE',  ( 122.6835989386367345, -43.14999999999999147, 34.92499999999998295 ) ) ;
#28236=AXIS2_PLACEMENT_3D ( 'NONE', #141663, #1645, #101706 ) ;
#28254=CARTESIAN_POINT ( 'NONE',  ( 12.31706980810188590, -2.126176841940956130, 7.934999999999990727 ) ) ;
#28304=AXIS2_PLACEMENT_3D ( 'NONE', #92804, #81978, #3620 ) ;
#28326=ORIENTED_EDGE ( 'NONE', *, *, #116500, .F. ) ;
#28329=CARTESIAN_POINT ( 'NONE',  ( 5.462903141435219823, -3.967499999999994476, 6.871911579029513106 ) ) ;
#28344=DIRECTION ( 'NONE',  ( 0.000000000000000000, 1.000000000000000000, -0.000000000000000000 ) ) ;
#28350=MECHANICAL_DESIGN_GEOMETRIC_PRESENTATION_REPRESENTATION('',(#65415),#127912);
#28379=ORIENTED_EDGE ( 'NONE', *, *, #39957, .F. ) ;
#28388=SURFACE_SIDE_STYLE ('',( #127704 ) ) ;
#28392=ORIENTED_EDGE ( 'NONE', *, *, #131571, .T. ) ;
#28395=CARTESIAN_POINT ( 'NONE',  ( 24.39999999999999858, -7.600000000000061817, 34.92499999999998295 ) ) ;
#28397=SURFACE_STYLE_USAGE ( .BOTH. , #127714 ) ;
#28414=FILL_AREA_STYLE_COLOUR ( '', #62848 ) ;
#28418=VERTEX_POINT ( 'NONE', #33704 ) ;
#28500=DIRECTION ( 'NONE',  ( -0.000000000000000000, -0.000000000000000000, 1.000000000000000000 ) ) ;
#28502=CARTESIAN_POINT ( 'NONE',  ( 12.60873647476855197, -5.808823158059033709, 5.808823158059035485 ) ) ;
#28503=CARTESIAN_POINT ( 'NONE',  ( 1.666965064704732269, -1.287028696899377367E-11, -6.428034935295263708 ) ) ;
#28533=ORIENTED_EDGE ( 'NONE', *, *, #67653, .F. ) ;
#28536=CARTESIAN_POINT ( 'NONE',  ( 7.707903141435220817, -6.871911579029513106, -3.967499999999993587 ) ) ;
#28545=CARTESIAN_POINT ( 'NONE',  ( 5.295806282870439752, -5.278424836066144543, 3.047499999999995879 ) ) ;
#28551=EDGE_CURVE ( 'NONE', #50573, #26834, #116119, .T. ) ;
#28563=CARTESIAN_POINT ( 'NONE',  ( 131.5423521607622490, -49.05583548141700589, 39.86617647058822911 ) ) ;
#28567=UNCERTAINTY_MEASURE_WITH_UNIT (LENGTH_MEASURE( 1.000000000000000082E-05 ), #62873, 'distance_accuracy_value', 'NONE');
#28594=DIRECTION ( 'NONE',  ( 0.000000000000000000, -0.000000000000000000, 1.000000000000000000 ) ) ;
#28662=CARTESIAN_POINT ( 'NONE',  ( 181.1499999999998067, -47.87246431468548735, -37.20487561447684044 ) ) ;
#28676=CARTESIAN_POINT ( 'NONE',  ( 11.71247294953710671, 0.000000000000000000, 6.094999999999989981 ) ) ;
#28678=ORIENTED_EDGE ( 'NONE', *, *, #20774, .F. ) ;
#28707=CARTESIAN_POINT ( 'NONE',  ( 34.24956980810188156, 3.967499999999998916, 6.871911579029510442 ) ) ;
#28720=CARTESIAN_POINT ( 'NONE',  ( 2.999999999999999112, -47.62213595499957108, -36.92499999999996874 ) ) ;
#28748=SURFACE_STYLE_USAGE ( .BOTH. , #6214 ) ;
#28750=CARTESIAN_POINT ( 'NONE',  ( 0.000000000000000000, 1.399999999999986366, 20.40202195861970580 ) ) ;
#28752=CARTESIAN_POINT ( 'NONE',  ( 32.81250000000000000, -4.461849672132299993, -4.461849672132299105 ) ) ;
#28773=CARTESIAN_POINT ( 'NONE',  ( 1.432180847299084014, -0.9397650347787239733, 6.598882878417470010 ) ) ;
#28784=EDGE_CURVE ( 'NONE', #104180, #62156, #110849, .T. ) ;
#28804=( NAMED_UNIT ( * ) SI_UNIT ( $, .STERADIAN. ) SOLID_ANGLE_UNIT ( ) );
#28806=EDGE_CURVE ( 'NONE', #111873, #81702, #62962, .T. ) ;
#28807=DIRECTION ( 'NONE',  ( 0.2400000000000087064, -1.734723475976868478E-16, -0.9707728879609257566 ) ) ;
#28813=SURFACE_STYLE_FILL_AREA ( #116523 ) ;
#28818=ADVANCED_FACE ( 'NONE', ( #112329 ), #67535, .T. ) ;
#28860=CARTESIAN_POINT ( 'NONE',  ( 0.4812208760381984640, -49.11951764990644165, 40.13200514437900068 ) ) ;
#28863=VECTOR ( 'NONE', #110770, 1000.000000000000000 ) ;
#28864=CARTESIAN_POINT ( 'NONE',  ( 7.707903141435219929, -6.871911579029513106, -3.967499999999993587 ) ) ;
#28868=STYLED_ITEM ( 'NONE', ( #5594 ), #7398 ) ;
#28874=( NAMED_UNIT ( * ) PLANE_ANGLE_UNIT ( ) SI_UNIT ( $, .RADIAN. ) );
#28905=CARTESIAN_POINT ( 'NONE',  ( 27.10373647476855652, 5.808823158059036373, 5.808823158059032821 ) ) ;
#28906=CARTESIAN_POINT ( 'NONE',  ( 8.437069808101885116, 2.126176841940952134, -7.934999999999992504 ) ) ;
#28907=DIRECTION ( 'NONE',  ( -1.000000000000000000, -0.000000000000000000, -0.000000000000000000 ) ) ;
#28926=PLANE ( 'NONE',  #119745 ) ;
#28942=CARTESIAN_POINT ( 'NONE',  ( 7.875000000000000000, -6.094999999999989981, 3.732111120401553285E-16 ) ) ;
#28963=CARTESIAN_POINT ( 'NONE',  ( 4.442069808101886785, 7.934999999999992504, 2.126176841940951689 ) ) ;
#28968=VECTOR ( 'NONE', #117238, 1000.000000000000000 ) ;
#28980=CARTESIAN_POINT ( 'NONE',  ( 6.416666666666666963, 5.278424836066147208, 3.047499999999990550 ) ) ;
#28993=EDGE_CURVE ( 'NONE', #15118, #23170, #44446, .T. ) ;
#29000=B_SPLINE_CURVE_WITH_KNOTS ( 'NONE', 3,
 ( #117250, #65635, #49912, #84664 ),
 .UNSPECIFIED., .F., .F.,
 ( 4, 4 ),
 ( 0.000000000000000000, 0.001824211539880447918 ),
 .UNSPECIFIED. ) ;
#29003=DIRECTION ( 'NONE',  ( 0.000000000000000000, -1.000000000000000000, 0.000000000000000000 ) ) ;
#29026=( BOUNDED_CURVE ( )  B_SPLINE_CURVE ( 2, ( #3832, #94448, #127078, #27055, #70616, #103878, #104619, #92298, #17590 ),
 .UNSPECIFIED., .F., .T. ) 
 B_SPLINE_CURVE_WITH_KNOTS ( ( 3, 2, 2, 2, 3 ),
 ( 0.7000000000000000666, 0.7083333333333334814, 0.7166666666666666741, 0.7249999999999999778, 0.7257331639278409297 ),
 .UNSPECIFIED. ) 
 CURVE ( )  GEOMETRIC_REPRESENTATION_ITEM ( )  RATIONAL_B_SPLINE_CURVE ( ( 0.9999999999999995559, 0.9659258262890687563, 1.000000000000000000, 0.9659258262890683122, 1.000000000000000000, 0.9659258262890683122, 1.000000000000000000, 0.9970021653956989693, 0.9945318277978396626 ) ) 
 REPRESENTATION_ITEM ( '' )  );
#29030=CARTESIAN_POINT ( 'NONE',  ( 13.04623647476855375, -7.934999999999990727, 4.858786175617117713E-16 ) ) ;
#29033=TOROIDAL_SURFACE ( 'NONE', #128592, 4.000000000000000000, 1.000000000000000000 ) ;
#29034=FACE_OUTER_BOUND ( 'NONE', #70638, .T. ) ;
#29038=LINE ( 'NONE', #119581, #81974 ) ;
#29040=( NAMED_UNIT ( * ) PLANE_ANGLE_UNIT ( ) SI_UNIT ( $, .RADIAN. ) );
#29042=CARTESIAN_POINT ( 'NONE',  ( 0.000000000000000000, -30.18000000000009564, -15.92500000000064375 ) ) ;
#29091=FILL_AREA_STYLE_COLOUR ( '', #34904 ) ;
#29154=( NAMED_UNIT ( * ) SI_UNIT ( $, .STERADIAN. ) SOLID_ANGLE_UNIT ( ) );
#29167=AXIS2_PLACEMENT_3D ( 'NONE', #69613, #114493, #125400 ) ;
#29188=LINE ( 'NONE', #84998, #50948 ) ;
#29190=CARTESIAN_POINT ( 'NONE',  ( 13.62956980810188767, -3.967499999999998028, -6.871911579029511330 ) ) ;
#29200=CARTESIAN_POINT ( 'NONE',  ( 10.54580628287044064, 5.278424836066143655, -3.047499999999997655 ) ) ;
#29214=FACE_OUTER_BOUND ( 'NONE', #79830, .T. ) ;
#29216=ORIENTED_EDGE ( 'NONE', *, *, #114038, .T. ) ;
#29223=CARTESIAN_POINT ( 'NONE',  ( 14.85373647476855474, -5.808823158059035485, -5.808823158059033709 ) ) ;
#29224=AXIS2_PLACEMENT_3D ( 'NONE', #77172, #130832, #63443 ) ;
#29240=STYLED_ITEM ( 'NONE', ( #16645 ), #33681 ) ;
#29255=DIRECTION ( 'NONE',  ( -1.000000000000000000, -0.000000000000000000, -0.000000000000000000 ) ) ;
#29326=ORIENTED_EDGE ( 'NONE', *, *, #116199, .F. ) ;
#29350=CARTESIAN_POINT ( 'NONE',  ( 16.96247294953710849, -7.464222240803106570E-16, -6.094999999999989981 ) ) ;
#29403=CARTESIAN_POINT ( 'NONE',  ( 0.3252437201535152145, -48.93522302958430004, -39.28544916627528494 ) ) ;
#29411=COLOUR_RGB ( '', 0.08235294, 0.09019608, 0.10196078) ;
#29419=DIRECTION ( 'NONE',  ( -1.000000000000000000, -0.000000000000000000, -0.000000000000000000 ) ) ;
#29432=CARTESIAN_POINT ( 'NONE',  ( 32.08333333333333570, -5.278424836066144543, 3.047499999999995879 ) ) ;
#29452=CARTESIAN_POINT ( 'NONE',  ( 13.56250000000000178, 4.461849672132300881, 4.461849672132299105 ) ) ;
#29457=( NAMED_UNIT ( * ) PLANE_ANGLE_UNIT ( ) SI_UNIT ( $, .RADIAN. ) );
#29459=ORIENTED_EDGE ( 'NONE', *, *, #104302, .T. ) ;
#29484=DIRECTION ( 'NONE',  ( 0.000000000000000000, -1.000000000000000000, 0.000000000000000000 ) ) ;
#29490=ORIENTED_EDGE ( 'NONE', *, *, #106636, .F. ) ;
#29492=CARTESIAN_POINT ( 'NONE',  ( 183.4813685602585167, -52.14999999947626463, 41.03936837847149377 ) ) ;
#29495=( LENGTH_UNIT ( ) NAMED_UNIT ( * ) SI_UNIT ( .MILLI., .METRE. ) );
#29513=ORIENTED_EDGE ( 'NONE', *, *, #107815, .F. ) ;
#29518=CARTESIAN_POINT ( 'NONE',  ( 8.212472949537106715, 0.000000000000000000, 6.094999999999989981 ) ) ;
#29536=COLOUR_RGB ( '', 0.40784314, 0.44705882, 0.49803922) ;
#29544=CARTESIAN_POINT ( 'NONE',  ( -2.554855379167821863E-16, -50.22575108204303973, 35.38524182944719598 ) ) ;
#29550=CARTESIAN_POINT ( 'NONE',  ( 1.291236474768552966, -9.717572351234235426E-16, -7.934999999999990727 ) ) ;
#29588=FILL_AREA_STYLE_COLOUR ( '', #8106 ) ;
#29595=CARTESIAN_POINT ( 'NONE',  ( 2.916666666666666963, 5.278424836066147208, 3.047499999999990550 ) ) ;
#29596=CARTESIAN_POINT ( 'NONE',  ( 5.082903141435219041, 3.967499999999992699, -6.871911579029513994 ) ) ;
#29617=( NAMED_UNIT ( * ) PLANE_ANGLE_UNIT ( ) SI_UNIT ( $, .RADIAN. ) );
#29622=CARTESIAN_POINT ( 'NONE',  ( 60.07317433568704246, -45.23984008851418537, 35.04755940937982217 ) ) ;
#29630=CARTESIAN_POINT ( 'NONE',  ( 8.458333333333333925, -3.047499999999997211, -5.278424836066143655 ) ) ;
#29650=CARTESIAN_POINT ( 'NONE',  ( 13.33790314143522160, -6.871911579029513106, -3.967499999999993587 ) ) ;
#29666=CARTESIAN_POINT ( 'NONE',  ( 5.833333333333333925, 5.278424836066143655, -3.047499999999997655 ) ) ;
#29704=ORIENTED_EDGE ( 'NONE', *, *, #124796, .T. ) ;
#29716=CARTESIAN_POINT ( 'NONE',  ( 14.06706980810188412, 2.126176841940952134, -7.934999999999993392 ) ) ;
#29721=DIRECTION ( 'NONE',  ( 0.000000000000000000, 0.000000000000000000, -1.000000000000000000 ) ) ;
#29726=CARTESIAN_POINT ( 'NONE',  ( 131.5423521607622774, -49.05583548141699168, -39.86617647058817226 ) ) ;
#29753=STYLED_ITEM ( 'NONE', ( #57379 ), #124337 ) ;
#29759=CARTESIAN_POINT ( 'NONE',  ( 0.1600000000000011691, -7.097592117162074388, -3.612066091894396092 ) ) ;
#29799=CARTESIAN_POINT ( 'NONE',  ( 28.00000000000002487, -52.14999999999999147, 34.92500000000003268 ) ) ;
#29802=FACE_OUTER_BOUND ( 'NONE', #110504, .T. ) ;
#29848=TOROIDAL_SURFACE ( 'NONE', #62278, 5.000000000000000000, 1.000000000000000000 ) ;
#29852=DIRECTION ( 'NONE',  ( -0.000000000000000000, 1.000000000000000000, -0.000000000000000000 ) ) ;
#29858=VERTEX_POINT ( 'NONE', #28165 ) ;
#29867=CYLINDRICAL_SURFACE ( 'NONE', #137113, 1.000000000000000888 ) ;
#29892=( NAMED_UNIT ( * ) SI_UNIT ( $, .STERADIAN. ) SOLID_ANGLE_UNIT ( ) );
#29894=CARTESIAN_POINT ( 'NONE',  ( 21.06706980810188412, 2.126176841940952134, -7.934999999999993392 ) ) ;
#29902=( GEOMETRIC_REPRESENTATION_CONTEXT ( 3 ) GLOBAL_UNCERTAINTY_ASSIGNED_CONTEXT ( ( #69573 ) ) GLOBAL_UNIT_ASSIGNED_CONTEXT ( ( #63765, #142046, #31830 ) ) REPRESENTATION_CONTEXT ( 'NONE', 'WORKASPACE' ) );
#29908=LINE ( 'NONE', #19756, #77062 ) ;
#29928=CARTESIAN_POINT ( 'NONE',  ( 12.37456980810188512, 6.871911579029510442, -3.967499999999998916 ) ) ;
#29959=DIRECTION ( 'NONE',  ( -0.000000000000000000, -5.782411586589356455E-15, -1.000000000000000000 ) ) ;
#29981=( GEOMETRIC_REPRESENTATION_CONTEXT ( 3 ) GLOBAL_UNCERTAINTY_ASSIGNED_CONTEXT ( ( #109849 ) ) GLOBAL_UNIT_ASSIGNED_CONTEXT ( ( #121620, #140029, #77457 ) ) REPRESENTATION_CONTEXT ( 'NONE', 'WORKASPACE' ) );
#29990=DIRECTION ( 'NONE',  ( -0.000000000000000000, 1.000000000000000000, 0.000000000000000000 ) ) ;
#29993=SURFACE_SIDE_STYLE ('',( #19827 ) ) ;
#30031=CARTESIAN_POINT ( 'NONE',  ( 26.40000000000000568, -16.48000000000005016, 33.92499999999998295 ) ) ;
#30047=CARTESIAN_POINT ( 'NONE',  ( 180.9587832221919257, -48.83231052142030393, -38.98973348322097365 ) ) ;
#30066=CARTESIAN_POINT ( 'NONE',  ( 28.48330628287044064, 6.094999999999991758, 1.633150327867687102 ) ) ;
#30083=COLOUR_RGB ( '', 0.31764706, 0.68627451, 0.89019608) ;
#30095=CARTESIAN_POINT ( 'NONE',  ( 152.4000000000000057, 7.919999999999947526, 19.12499999999998224 ) ) ;
#30098=EDGE_CURVE ( 'NONE', #5240, #113523, #143452, .T. ) ;
#30103=CARTESIAN_POINT ( 'NONE',  ( 31.04123647476855297, 0.000000000000000000, 7.934999999999990727 ) ) ;
#30116=CARTESIAN_POINT ( 'NONE',  ( 0.06788206741517728571, -51.13011358081256219, -36.94363806876511802 ) ) ;
#30121=CARTESIAN_POINT ( 'NONE',  ( 184.1500000000000057, -57.15000000000003411, -15.92500000000064730 ) ) ;
#30139=UNCERTAINTY_MEASURE_WITH_UNIT (LENGTH_MEASURE( 1.000000000000000082E-05 ), #121693, 'distance_accuracy_value', 'NONE');
#30150=CARTESIAN_POINT ( 'NONE',  ( 31.64583333333333925, -1.633150327867689988, 6.094999999999989981 ) ) ;
#30165=( GEOMETRIC_REPRESENTATION_CONTEXT ( 3 ) GLOBAL_UNCERTAINTY_ASSIGNED_CONTEXT ( ( #121592 ) ) GLOBAL_UNIT_ASSIGNED_CONTEXT ( ( #83434, #29040, #4355 ) ) REPRESENTATION_CONTEXT ( 'NONE', 'WORKASPACE' ) );
#30173=( NAMED_UNIT ( * ) SI_UNIT ( $, .STERADIAN. ) SOLID_ANGLE_UNIT ( ) );
#30202=EDGE_CURVE ( 'NONE', #50573, #93784, #24419, .T. ) ;
#30204=COLOUR_RGB ( '', 0.66274510, 0.83137255, 0.94901961) ;
#30207=( LENGTH_UNIT ( ) NAMED_UNIT ( * ) SI_UNIT ( .MILLI., .METRE. ) );
#30218=CIRCLE ( 'NONE', #53402, 1.000000000000000000 ) ;
#30219=CARTESIAN_POINT ( 'NONE',  ( 180.9625229943972613, -48.82538788374357352, 38.96958855984509995 ) ) ;
#30255=MECHANICAL_DESIGN_GEOMETRIC_PRESENTATION_REPRESENTATION('',(#97283),#60405);
#30275=CARTESIAN_POINT ( 'NONE',  ( 3.596992905810010743, -49.14999999999999147, 40.56450646617209799 ) ) ;
#30278=CARTESIAN_POINT ( 'NONE',  ( 6.832903141435220817, -3.967499999999994476, 6.871911579029513106 ) ) ;
#30317=FACE_OUTER_BOUND ( 'NONE', #55606, .T. ) ;
#30321=AXIS2_PLACEMENT_3D ( 'NONE', #48397, #28807, #61461 ) ;
#30326=CARTESIAN_POINT ( 'NONE',  ( 8.750000000000000000, -7.464222240803106570E-16, -6.094999999999989981 ) ) ;
#30328=CARTESIAN_POINT ( 'NONE',  ( 19.22873647476855297, 5.808823158059031044, -5.808823158059037262 ) ) ;
#30359=CARTESIAN_POINT ( 'NONE',  ( 128.6723146206077502, -49.13871568196919526, 40.16438383193056438 ) ) ;
#30360=CARTESIAN_POINT ( 'NONE',  ( 7.291666666666667851, -3.047499999999994547, 5.278424836066145431 ) ) ;
#30362=MECHANICAL_DESIGN_GEOMETRIC_PRESENTATION_REPRESENTATION('',(#127648),#44255);
#30406=FILL_AREA_STYLE ('',( #10757 ) ) ;
#30410=AXIS2_PLACEMENT_3D ( 'NONE', #46978, #124478, #123062 ) ;
#30417=CARTESIAN_POINT ( 'NONE',  ( 25.40000000000001634, 3.638354173706144667, -7.063344996420134692 ) ) ;
#30433=CARTESIAN_POINT ( 'NONE',  ( 149.2199999999997999, -3.180000000000061444, -31.92499999999998295 ) ) ;
#30461=CARTESIAN_POINT ( 'NONE',  ( 7.796236474768553748, 7.934999999999990727, -1.457635852685135314E-15 ) ) ;
#30482=EDGE_CURVE ( 'NONE', #3140, #121198, #16761, .T. ) ;
#30493=ORIENTED_EDGE ( 'NONE', *, *, #129266, .T. ) ;
#30502=UNCERTAINTY_MEASURE_WITH_UNIT (LENGTH_MEASURE( 1.000000000000000082E-05 ), #103757, 'distance_accuracy_value', 'NONE');
#30507=CARTESIAN_POINT ( 'NONE',  ( 0.1600000000000023348, -7.836308044950259344, 1.291832889770243353 ) ) ;
#30539=SURFACE_SIDE_STYLE ('',( #75469 ) ) ;
#30544=DIRECTION ( 'NONE',  ( 0.000000000000000000, -1.000000000000000000, 0.000000000000000000 ) ) ;
#30557=CARTESIAN_POINT ( 'NONE',  ( 25.39999999999999858, -30.18000000000009564, -15.92500000000064375 ) ) ;
#30568=( BOUNDED_CURVE ( )  B_SPLINE_CURVE ( 3, ( #67075, #142500, #109851, #143196 ),
 .UNSPECIFIED., .F., .T. ) 
 B_SPLINE_CURVE_WITH_KNOTS ( ( 4, 4 ),
 ( 0.1773996044403691741, 1.570796326794896558 ),
 .UNSPECIFIED. ) 
 CURVE ( )  GEOMETRIC_REPRESENTATION_ITEM ( )  RATIONAL_B_SPLINE_CURVE ( ( 1.000000000000000000, 0.8446433258982466441, 0.8446433258982466441, 1.000000000000000000 ) ) 
 REPRESENTATION_ITEM ( '' )  );
#30587=AXIS2_PLACEMENT_3D ( 'NONE', #22562, #132827, #86451 ) ;
#30591=STYLED_ITEM ( 'NONE', ( #51313 ), #118172 ) ;
#30607=CARTESIAN_POINT ( 'NONE',  ( 3.600192512601675610, -49.14999999999999858, 40.57313449935462302 ) ) ;
#30632=EDGE_CURVE ( 'NONE', #140063, #26733, #12868, .T. ) ;
#30644=CARTESIAN_POINT ( 'NONE',  ( 0.000000000000000000, 9.913515839097813477E-16, -8.094999999999991758 ) ) ;
#30647=CARTESIAN_POINT ( 'NONE',  ( 17.85873647476854842, 5.808823158059031044, -5.808823158059038150 ) ) ;
#30654=DIRECTION ( 'NONE',  ( 0.000000000000000000, 0.000000000000000000, 1.000000000000000000 ) ) ;
#30665=DIRECTION ( 'NONE',  ( 0.000000000000000000, 5.782411586589356455E-15, -1.000000000000000000 ) ) ;
#30680=CARTESIAN_POINT ( 'NONE',  ( 12.95790314143521904, 6.871911579029515771, 3.967499999999989146 ) ) ;
#30747=CARTESIAN_POINT ( 'NONE',  ( 9.962472949537104938, -7.464222240803106570E-16, -6.094999999999989981 ) ) ;
#30752=SURFACE_STYLE_USAGE ( .BOTH. , #100279 ) ;
#30818=ORIENTED_EDGE ( 'NONE', *, *, #83119, .T. ) ;
#30822=CARTESIAN_POINT ( 'NONE',  ( 26.58747294953710494, -6.094999999999989981, 3.732111120401553285E-16 ) ) ;
#30897=CARTESIAN_POINT ( 'NONE',  ( 34.85416666666666430, 1.633150327867695095, 6.094999999999988205 ) ) ;
#30920=LINE ( 'NONE', #72316, #72468 ) ;
#30952=FILL_AREA_STYLE_COLOUR ( '', #94338 ) ;
#30963=CARTESIAN_POINT ( 'NONE',  ( 184.1173099067358123, -47.89015928896270680, 37.22465919495247988 ) ) ;
#30983=( GEOMETRIC_REPRESENTATION_CONTEXT ( 3 ) GLOBAL_UNCERTAINTY_ASSIGNED_CONTEXT ( ( #121432 ) ) GLOBAL_UNIT_ASSIGNED_CONTEXT ( ( #1627, #38405, #77812 ) ) REPRESENTATION_CONTEXT ( 'NONE', 'WORKASPACE' ) );
#31013=SURFACE_STYLE_FILL_AREA ( #95520 ) ;
#31017=CARTESIAN_POINT ( 'NONE',  ( 3.332903141435219929, -3.967499999999994476, 6.871911579029513106 ) ) ;
#31019=DIRECTION ( 'NONE',  ( 0.000000000000000000, -1.000000000000000000, 0.000000000000000000 ) ) ;
#31044=VECTOR ( 'NONE', #89990, 1000.000000000000000 ) ;
#31054=( LENGTH_UNIT ( ) NAMED_UNIT ( * ) SI_UNIT ( .MILLI., .METRE. ) );
#31057=MECHANICAL_DESIGN_GEOMETRIC_PRESENTATION_REPRESENTATION('',(#95913),#56647);
#31063=CARTESIAN_POINT ( 'NONE',  ( 5.541666666666666963, 3.047499999999993214, -5.278424836066146320 ) ) ;
#31064=CARTESIAN_POINT ( 'NONE',  ( 21.56206980810188867, -7.934999999999990727, -2.126176841940955242 ) ) ;
#31076=CARTESIAN_POINT ( 'NONE',  ( 127.4973405139118228, -50.37061236291009436, -37.32649486623493829 ) ) ;
#31089=CARTESIAN_POINT ( 'NONE',  ( 58.77385498567259958, -47.18881911353556546, 35.55177538329026277 ) ) ;
#31096=CARTESIAN_POINT ( 'NONE',  ( 128.5065401839287631, -48.97294124528377779, 39.12804664298170820 ) ) ;
#31107=CARTESIAN_POINT ( 'NONE',  ( 28.00000000000002487, -49.14999999999999147, 40.92499999999998295 ) ) ;
#31112=ORIENTED_EDGE ( 'NONE', *, *, #81751, .T. ) ;
#31116=CARTESIAN_POINT ( 'NONE',  ( 19.75456980810189123, -6.871911579029512218, 3.967499999999996252 ) ) ;
#31135=PRESENTATION_STYLE_ASSIGNMENT (( #120967 ) ) ;
#31141=FILL_AREA_STYLE ('',( #63770 ) ) ;
#31144=CARTESIAN_POINT ( 'NONE',  ( 25.39999999999999147, 4.335470510665683896, -6.649025316336889091 ) ) ;
#31146=VERTEX_POINT ( 'NONE', #53512 ) ;
#31157=MECHANICAL_DESIGN_GEOMETRIC_PRESENTATION_REPRESENTATION('',(#119088),#130717);
#31183=CARTESIAN_POINT ( 'NONE',  ( 10.71290314143521982, 3.967499999999992699, -6.871911579029513994 ) ) ;
#31239=EDGE_LOOP ( 'NONE', ( #5840, #125113, #91338, #128733 ) ) ;
#31270=DIRECTION ( 'NONE',  ( 0.000000000000000000, -1.000000000000000000, 0.000000000000000000 ) ) ;
#31273=ADVANCED_FACE ( 'NONE', ( #89698 ), #98437, .T. ) ;
#31291=DIRECTION ( 'NONE',  ( 0.000000000000000000, 0.000000000000000000, -1.000000000000000000 ) ) ;
#31296=ORIENTED_EDGE ( 'NONE', *, *, #110303, .F. ) ;
#31324=( NAMED_UNIT ( * ) SI_UNIT ( $, .STERADIAN. ) SOLID_ANGLE_UNIT ( ) );
#31334=ORIENTED_EDGE ( 'NONE', *, *, #21381, .F. ) ;
#31335=ORIENTED_EDGE ( 'NONE', *, *, #90529, .T. ) ;
#31336=CARTESIAN_POINT ( 'NONE',  ( 19.00413961620377279, -3.047499999999994547, 5.278424836066145431 ) ) ;
#31351=CARTESIAN_POINT ( 'NONE',  ( 18.58790314143521982, 6.871911579029515771, 3.967499999999989146 ) ) ;
#31369=DIRECTION ( 'NONE',  ( 1.000000000000000000, 0.000000000000000000, 0.000000000000000000 ) ) ;
#31385=DIRECTION ( 'NONE',  ( 0.000000000000000000, 0.000000000000000000, 1.000000000000000000 ) ) ;
#31388=CARTESIAN_POINT ( 'NONE',  ( 5.587472949537105826, -6.094999999999989981, 3.732111120401553285E-16 ) ) ;
#31395=SURFACE_SIDE_STYLE ('',( #140841 ) ) ;
#31397=ORIENTED_EDGE ( 'NONE', *, *, #63475, .F. ) ;
#31418=CARTESIAN_POINT ( 'NONE',  ( 153.4000000000000057, -1.600000000000086020, -33.92499999999998295 ) ) ;
#31446=ORIENTED_EDGE ( 'NONE', *, *, #137756, .T. ) ;
#31452=( NAMED_UNIT ( * ) PLANE_ANGLE_UNIT ( ) SI_UNIT ( $, .RADIAN. ) );
#31479=LINE ( 'NONE', #19165, #120685 ) ;
#31515=CARTESIAN_POINT ( 'NONE',  ( 24.98330628287043709, 6.094999999999991758, 1.633150327867687102 ) ) ;
#31544=DIRECTION ( 'NONE',  ( 0.000000000000000000, -1.000000000000000000, 0.000000000000000000 ) ) ;
#31548=CARTESIAN_POINT ( 'NONE',  ( 25.39999999999999858, 7.464222240803104598E-16, -6.094999999999989093 ) ) ;
#31578=CARTESIAN_POINT ( 'NONE',  ( 184.1500000000000057, -43.14999999999999147, 31.92499999999998295 ) ) ;
#31585=DIRECTION ( 'NONE',  ( 1.000000000000000000, 0.000000000000000000, 0.000000000000000000 ) ) ;
#31591=EDGE_CURVE ( 'NONE', #134245, #61213, #109380, .T. ) ;
#31597=VERTEX_POINT ( 'NONE', #62097 ) ;
#31607=SURFACE_STYLE_USAGE ( .BOTH. , #130938 ) ;
#31609=CIRCLE ( 'NONE', #91811, 1.000000000000000888 ) ;
#31663=( NAMED_UNIT ( * ) SI_UNIT ( $, .STERADIAN. ) SOLID_ANGLE_UNIT ( ) );
#31711=CARTESIAN_POINT ( 'NONE',  ( 10.62456980810188689, -6.871911579029512218, 3.967499999999996252 ) ) ;
#31722=PRESENTATION_STYLE_ASSIGNMENT (( #97684 ) ) ;
#31740=STYLED_ITEM ( 'NONE', ( #26646 ), #111891 ) ;
#31748=ORIENTED_EDGE ( 'NONE', *, *, #67089, .F. ) ;
#31751=( NAMED_UNIT ( * ) SI_UNIT ( $, .STERADIAN. ) SOLID_ANGLE_UNIT ( ) );
#31760=CARTESIAN_POINT ( 'NONE',  ( 1.750000000000000222, -7.464222240803106570E-16, -6.094999999999989981 ) ) ;
#31761=CARTESIAN_POINT ( 'NONE',  ( 12.81206980810188334, 7.934999999999992504, 2.126176841940951689 ) ) ;
#31774=CARTESIAN_POINT ( 'NONE',  ( 130.2059003229214227, -48.16486758952284930, -37.61253110040706105 ) ) ;
#31779=( LENGTH_UNIT ( ) NAMED_UNIT ( * ) SI_UNIT ( .MILLI., .METRE. ) );
#31788=DIRECTION ( 'NONE',  ( 0.000000000000000000, -1.000000000000000000, 0.000000000000000000 ) ) ;
#31796=CARTESIAN_POINT ( 'NONE',  ( 128.5740698622001901, -49.04047092357102855, 39.41690992498948987 ) ) ;
#31801=CARTESIAN_POINT ( 'NONE',  ( 183.7627343495647665, -51.96230815476840803, 39.57541490114646621 ) ) ;
#31803=( BOUNDED_CURVE ( )  B_SPLINE_CURVE ( 3, ( #27457, #101642, #132885, #90798 ),
 .UNSPECIFIED., .F., .F. ) 
 B_SPLINE_CURVE_WITH_KNOTS ( ( 4, 4 ),
 ( 4.712388980384689674, 6.105785702739217946 ),
 .UNSPECIFIED. ) 
 CURVE ( )  GEOMETRIC_REPRESENTATION_ITEM ( )  RATIONAL_B_SPLINE_CURVE ( ( 1.000000000000000000, 0.8446433258982464221, 0.8446433258982464221, 1.000000000000000000 ) ) 
 REPRESENTATION_ITEM ( '' )  );
#31814=CARTESIAN_POINT ( 'NONE',  ( 17.56706980810188767, 2.126176841940952134, -7.934999999999992504 ) ) ;
#31830=( NAMED_UNIT ( * ) SI_UNIT ( $, .STERADIAN. ) SOLID_ANGLE_UNIT ( ) );
#31836=( NAMED_UNIT ( * ) SI_UNIT ( $, .STERADIAN. ) SOLID_ANGLE_UNIT ( ) );
#31842=ORIENTED_EDGE ( 'NONE', *, *, #30632, .F. ) ;
#31856=FACE_OUTER_BOUND ( 'NONE', #72305, .T. ) ;
#31866=EDGE_LOOP ( 'NONE', ( #102173, #53537, #31112, #58674, #4807, #58060, #143398, #126352 ) ) ;
#31874=FILL_AREA_STYLE ('',( #54376 ) ) ;
#31884=CARTESIAN_POINT ( 'NONE',  ( 18.15040314143522338, 7.934999999999989839, -2.126176841940961904 ) ) ;
#31928=SURFACE_STYLE_USAGE ( .BOTH. , #120316 ) ;
#31953=PRESENTATION_STYLE_ASSIGNMENT (( #142165 ) ) ;
#31985=SURFACE_STYLE_FILL_AREA ( #98659 ) ;
#32055=CARTESIAN_POINT ( 'NONE',  ( 19.31706980810189123, -2.126176841940956130, 7.934999999999991616 ) ) ;
#32165=B_SPLINE_CURVE_WITH_KNOTS ( 'NONE', 3,
 ( #126700, #49189, #60799, #5627 ),
 .UNSPECIFIED., .F., .F.,
 ( 4, 4 ),
 ( 0.000000000000000000, 0.001115544020566805418 ),
 .UNSPECIFIED. ) ;
#32175=STYLED_ITEM ( 'NONE', ( #93974 ), #95871 ) ;
#32182=AXIS2_PLACEMENT_3D ( 'NONE', #65679, #77254, #54767 ) ;
#32192=COLOUR_RGB ( '', 0.40784314, 0.44705882, 0.49803922) ;
#32211=CARTESIAN_POINT ( 'NONE',  ( 2.999999999999999112, -7.600000000000061817, 28.92499999999998650 ) ) ;
#32217=FILL_AREA_STYLE ('',( #131527 ) ) ;
#32229=CARTESIAN_POINT ( 'NONE',  ( 20.60830628287043709, 1.633150327867687324, -6.094999999999991758 ) ) ;
#32250=STYLED_ITEM ( 'NONE', ( #38454 ), #70028 ) ;
#32273=EDGE_LOOP ( 'NONE', ( #48181, #112492, #117656, #44344 ) ) ;
#32280=CARTESIAN_POINT ( 'NONE',  ( 28.00000000000002487, -52.14999999999999147, -34.92499999999976978 ) ) ;
#32300=CARTESIAN_POINT ( 'NONE',  ( 152.4000000000000057, 25.96999999999993847, 33.92499999999998295 ) ) ;
#32303=VECTOR ( 'NONE', #29255, 1000.000000000000000 ) ;
#32319=( GEOMETRIC_REPRESENTATION_CONTEXT ( 3 ) GLOBAL_UNCERTAINTY_ASSIGNED_CONTEXT ( ( #115862 ) ) GLOBAL_UNIT_ASSIGNED_CONTEXT ( ( #13359, #112004, #142491 ) ) REPRESENTATION_CONTEXT ( 'NONE', 'WORKASPACE' ) );
#32332=CARTESIAN_POINT ( 'NONE',  ( 55.56056557994608625, -52.00875322212550600, 39.86617647058822200 ) ) ;
#32375=ADVANCED_FACE ( 'NONE', ( #97746 ), #119466, .F. ) ;
#32380=EDGE_CURVE ( 'NONE', #74861, #63837, #42708, .T. ) ;
#32387=EDGE_CURVE ( 'NONE', #5277, #79775, #86531, .T. ) ;
#32408=FILL_AREA_STYLE ('',( #75214 ) ) ;
#32435=CARTESIAN_POINT ( 'NONE',  ( 17.33290314143522082, -3.967499999999994476, 6.871911579029513106 ) ) ;
#32442=CARTESIAN_POINT ( 'NONE',  ( 20.70833333333333570, 3.047499999999997655, 5.278424836066143655 ) ) ;
#32476=SURFACE_SIDE_STYLE ('',( #53511 ) ) ;
#32480=CARTESIAN_POINT ( 'NONE',  ( 1.312499999999999778, -4.461849672132299993, -4.461849672132299105 ) ) ;
#32481=CARTESIAN_POINT ( 'NONE',  ( 21.27040314143522082, -7.934999999999988951, 2.126176841940957907 ) ) ;
#32496=FILL_AREA_STYLE ('',( #55682 ) ) ;
#32503=CYLINDRICAL_SURFACE ( 'NONE', #71719, 3.999999999999996447 ) ;
#32508=SURFACE_STYLE_USAGE ( .BOTH. , #98461 ) ;
#32538=CARTESIAN_POINT ( 'NONE',  ( 3.730677800976855973, -49.14999999999999147, -40.92499999999998295 ) ) ;
#32562=DIRECTION ( 'NONE',  ( 0.000000000000000000, -1.000000000000000000, -1.091707662666338270E-16 ) ) ;
#32570=PRESENTATION_STYLE_ASSIGNMENT (( #131876 ) ) ;
#32606=STYLED_ITEM ( 'NONE', ( #45323 ), #82293 ) ;
#32613=ORIENTED_EDGE ( 'NONE', *, *, #92748, .F. ) ;
#32616=CARTESIAN_POINT ( 'NONE',  ( 15.81706980810188767, -2.126176841940956130, 7.934999999999991616 ) ) ;
#32636=DIRECTION ( 'NONE',  ( 0.000000000000000000, 0.000000000000000000, -1.000000000000000000 ) ) ;
#32644=DIRECTION ( 'NONE',  ( -1.000000000000000000, -0.000000000000000000, -0.000000000000000000 ) ) ;
#32675=VECTOR ( 'NONE', #129667, 1000.000000000000000 ) ;
#32690=CARTESIAN_POINT ( 'NONE',  ( 24.50000000000000000, 0.000000000000000000, 6.094999999999989981 ) ) ;
#32719=EDGE_LOOP ( 'NONE', ( #65005, #118252, #25426 ) ) ;
#32733=SURFACE_STYLE_USAGE ( .BOTH. , #89930 ) ;
#32751=VERTEX_POINT ( 'NONE', #77899 ) ;
#32783=AXIS2_PLACEMENT_3D ( 'NONE', #142101, #76852, #42788 ) ;
#32785=CARTESIAN_POINT ( 'NONE',  ( 166.8575281714868481, 26.96999999999994557, -32.10255624693994747 ) ) ;
#32794=CARTESIAN_POINT ( 'NONE',  ( 19.02540314143521982, 2.126176841940962348, 7.934999999999989839 ) ) ;
#32815=CARTESIAN_POINT ( 'NONE',  ( 151.4000000000000057, -16.48000000000005016, -33.92499999999998295 ) ) ;
#32882=COLOUR_RGB ( '', 0.40784314, 0.44705882, 0.49803922) ;
#32887=SURFACE_STYLE_FILL_AREA ( #65524 ) ;
#32888=ORIENTED_EDGE ( 'NONE', *, *, #119476, .F. ) ;
#32953=LINE ( 'NONE', #47930, #50663 ) ;
#32964=PRESENTATION_STYLE_ASSIGNMENT (( #112629 ) ) ;
#32974=CARTESIAN_POINT ( 'NONE',  ( 27.89997294953710494, 4.461849672132297329, -4.461849672132302658 ) ) ;
#33006=EDGE_CURVE ( 'NONE', #75731, #134905, #139839, .T. ) ;
#33011=CARTESIAN_POINT ( 'NONE',  ( -0.4587635252314472556, 0.000000000000000000, 7.934999999999990727 ) ) ;
#33030=STYLED_ITEM ( 'NONE', ( #57767 ), #86018 ) ;
#33038=VECTOR ( 'NONE', #31788, 1000.000000000000000 ) ;
#33052=CARTESIAN_POINT ( 'NONE',  ( 16.52497294953710849, -4.461849672132299993, -4.461849672132299105 ) ) ;
#33058=ORIENTED_EDGE ( 'NONE', *, *, #100819, .T. ) ;
#33062=EDGE_CURVE ( 'NONE', #121198, #96033, #26401, .T. ) ;
#33078=EDGE_CURVE ( 'NONE', #121198, #11327, #70423, .T. ) ;
#33116=CARTESIAN_POINT ( 'NONE',  ( 180.8471172286433841, -48.98543874033772738, 39.51758185027075143 ) ) ;
#33132=ORIENTED_EDGE ( 'NONE', *, *, #39622, .T. ) ;
#33147=ADVANCED_FACE ( 'NONE', ( #141036 ), #112085, .F. ) ;
#33149=ORIENTED_EDGE ( 'NONE', *, *, #77719, .F. ) ;
#33155=CARTESIAN_POINT ( 'NONE',  ( 0.4833062828704390301, 6.094999999999991758, 1.633150327867687102 ) ) ;
#33160=CARTESIAN_POINT ( 'NONE',  ( 2.000000000000008882, 0.000000000000000000, 0.000000000000000000 ) ) ;
#33165=DIRECTION ( 'NONE',  ( -1.000000000000000000, -0.000000000000000000, -0.000000000000000000 ) ) ;
#33168=SURFACE_STYLE_USAGE ( .BOTH. , #54893 ) ;
#33181=CARTESIAN_POINT ( 'NONE',  ( 12.95790314143521904, 6.871911579029515771, 3.967499999999989146 ) ) ;
#33206=VERTEX_POINT ( 'NONE', #32300 ) ;
#33207=( GEOMETRIC_REPRESENTATION_CONTEXT ( 3 ) GLOBAL_UNCERTAINTY_ASSIGNED_CONTEXT ( ( #1393 ) ) GLOBAL_UNIT_ASSIGNED_CONTEXT ( ( #82010, #126190, #82692 ) ) REPRESENTATION_CONTEXT ( 'NONE', 'WORKASPACE' ) );
#33208=CARTESIAN_POINT ( 'NONE',  ( 17.54580628287044064, 5.278424836066143655, -3.047499999999997655 ) ) ;
#33224=EDGE_CURVE ( 'NONE', #91232, #111908, #63929, .T. ) ;
#33229=CARTESIAN_POINT ( 'NONE',  ( 11.81250000000000355, -4.461849672132299993, -4.461849672132299105 ) ) ;
#33230=CARTESIAN_POINT ( 'NONE',  ( 18.49956980810188867, -3.967499999999998028, -6.871911579029511330 ) ) ;
#33244=CARTESIAN_POINT ( 'NONE',  ( 128.6577301979894798, -49.12413125935659508, -39.93743342457428724 ) ) ;
#33251=CARTESIAN_POINT ( 'NONE',  ( 156.1500000000000057, -49.14999999999999147, -49.92499999999968452 ) ) ;
#33260=LINE ( 'NONE', #12162, #33038 ) ;
#33286=CARTESIAN_POINT ( 'NONE',  ( 15.67123647476855552, 0.000000000000000000, 7.934999999999990727 ) ) ;
#33295=ORIENTED_EDGE ( 'NONE', *, *, #27117, .T. ) ;
#33357=CARTESIAN_POINT ( 'NONE',  ( 14.50456980810188767, 6.871911579029510442, -3.967499999999998916 ) ) ;
#33373=DIRECTION ( 'NONE',  ( -1.000000000000000000, 0.000000000000000000, 0.000000000000000000 ) ) ;
#33382=ORIENTED_EDGE ( 'NONE', *, *, #72932, .T. ) ;
#33385=DIRECTION ( 'NONE',  ( -0.000000000000000000, 1.000000000000000000, -0.000000000000000000 ) ) ;
#33398=CARTESIAN_POINT ( 'NONE',  ( 16.74956980810188867, 3.967499999999998916, 6.871911579029510442 ) ) ;
#33420=EDGE_CURVE ( 'NONE', #96438, #105463, #3537, .T. ) ;
#33428=ADVANCED_FACE ( 'NONE', ( #115508 ), #130618, .T. ) ;
#33477=CARTESIAN_POINT ( 'NONE',  ( 23.96247294953710849, -7.464222240803106570E-16, -6.094999999999989981 ) ) ;
#33494=CARTESIAN_POINT ( 'NONE',  ( 152.4000000000000057, -14.29000000000013593, -12.70000000000045404 ) ) ;
#33513=CARTESIAN_POINT ( 'NONE',  ( 30.98373647476855552, -5.808823158059035485, -5.808823158059033709 ) ) ;
#33522=ORIENTED_EDGE ( 'NONE', *, *, #121896, .T. ) ;
#33621=AXIS2_PLACEMENT_3D ( 'NONE', #78872, #111467, #67269 ) ;
#33644=( GEOMETRIC_REPRESENTATION_CONTEXT ( 3 ) GLOBAL_UNCERTAINTY_ASSIGNED_CONTEXT ( ( #21563 ) ) GLOBAL_UNIT_ASSIGNED_CONTEXT ( ( #129652, #29617, #86170 ) ) REPRESENTATION_CONTEXT ( 'NONE', 'WORKASPACE' ) );
#33671=EDGE_CURVE ( 'NONE', #122655, #40407, #117184, .T. ) ;
#33678=CARTESIAN_POINT ( 'NONE',  ( 4.296236474768552860, 7.934999999999990727, -1.457635852685135314E-15 ) ) ;
#33681=ADVANCED_FACE ( 'NONE', ( #126827 ), #47895, .F. ) ;
#33687=FILL_AREA_STYLE_COLOUR ( '', #105124 ) ;
#33704=CARTESIAN_POINT ( 'NONE',  ( 1.369639479247480862, 4.811953009385816285E-13, 6.725360520752516891 ) ) ;
#33707=ADVANCED_FACE ( 'NONE', ( #128133 ), #52415, .T. ) ;
#33711=( LENGTH_UNIT ( ) NAMED_UNIT ( * ) SI_UNIT ( .MILLI., .METRE. ) );
#33781=DIRECTION ( 'NONE',  ( 0.000000000000000000, 0.000000000000000000, 1.000000000000000000 ) ) ;
#33797=CARTESIAN_POINT ( 'NONE',  ( 24.39999999999999858, -1.600000000000094458, 34.92499999999998295 ) ) ;
#33799=VERTEX_POINT ( 'NONE', #43970 ) ;
#33804=( LENGTH_UNIT ( ) NAMED_UNIT ( * ) SI_UNIT ( .MILLI., .METRE. ) );
#33816=CARTESIAN_POINT ( 'NONE',  ( 3.399972949537105826, 4.461849672132297329, -4.461849672132302658 ) ) ;
#33843=CARTESIAN_POINT ( 'NONE',  ( -2.287527050462894618, 0.000000000000000000, 6.094999999999989981 ) ) ;
#33846=COLOUR_RGB ( '', 0.66274510, 0.83137255, 0.94901961) ;
#33867=CARTESIAN_POINT ( 'NONE',  ( 16.89540314143521726, 2.126176841940962348, 7.934999999999989839 ) ) ;
#33875=SURFACE_SIDE_STYLE ('',( #77402 ) ) ;
#33909=STYLED_ITEM ( 'NONE', ( #112239 ), #91558 ) ;
#33913=CARTESIAN_POINT ( 'NONE',  ( 16.62500000000000000, 6.094999999999989981, -1.119633336120465690E-15 ) ) ;
#33927=CARTESIAN_POINT ( 'NONE',  ( 125.6094186379952902, -46.07581969935851163, -35.63601533998082260 ) ) ;
#33938=DIRECTION ( 'NONE',  ( 0.000000000000000000, -1.000000000000000000, 0.000000000000000000 ) ) ;
#34017=EDGE_CURVE ( 'NONE', #79053, #137006, #52678, .T. ) ;
#34043=AXIS2_PLACEMENT_3D ( 'NONE', #93288, #103426, #28038 ) ;
#34044=CARTESIAN_POINT ( 'NONE',  ( 19.02540314143521982, 2.126176841940962348, 7.934999999999989839 ) ) ;
#34055=DIRECTION ( 'NONE',  ( 0.000000000000000000, -1.000000000000000000, 0.000000000000000000 ) ) ;
#34060=LINE ( 'NONE', #58709, #27210 ) ;
#34088=CARTESIAN_POINT ( 'NONE',  ( 17.33290314143522082, -3.967499999999994476, 6.871911579029513106 ) ) ;
#34089=CARTESIAN_POINT ( 'NONE',  ( 1.437069808101886004, 2.126176841940952134, -7.934999999999992504 ) ) ;
#34116=CARTESIAN_POINT ( 'NONE',  ( 27.99999999999996803, -49.14999999999999147, 53.92499999999996874 ) ) ;
#34120=VECTOR ( 'NONE', #132958, 1000.000000000000000 ) ;
#34160=ORIENTED_EDGE ( 'NONE', *, *, #38752, .F. ) ;
#34177=( NAMED_UNIT ( * ) PLANE_ANGLE_UNIT ( ) SI_UNIT ( $, .RADIAN. ) );
#34194=CARTESIAN_POINT ( 'NONE',  ( 166.8266634454907660, 26.96999999999994557, -32.27463857217006904 ) ) ;
#34197=EDGE_CURVE ( 'NONE', #62041, #105140, #133229, .T. ) ;
#34203=CARTESIAN_POINT ( 'NONE',  ( 26.46290314143521982, -3.967499999999994476, 6.871911579029513106 ) ) ;
#34298=EDGE_CURVE ( 'NONE', #94899, #53957, #114606, .T. ) ;
#34371=CARTESIAN_POINT ( 'NONE',  ( -0.3704301918981141029, -3.967499999999998028, -6.871911579029511330 ) ) ;
#34391=DIRECTION ( 'NONE',  ( -1.000000000000000000, -0.000000000000000000, -0.000000000000000000 ) ) ;
#34403=SURFACE_STYLE_FILL_AREA ( #100382 ) ;
#34422=STYLED_ITEM ( 'NONE', ( #127390 ), #69272 ) ;
#34438=CARTESIAN_POINT ( 'NONE',  ( 15.94163961620377279, -6.094999999999989093, 1.633150327867691542 ) ) ;
#34471=DIRECTION ( 'NONE',  ( 0.000000000000000000, 0.7453559924999330066, 0.6666666666666630769 ) ) ;
#34503=ORIENTED_EDGE ( 'NONE', *, *, #123118, .T. ) ;
#34518=DIRECTION ( 'NONE',  ( 0.000000000000000000, 0.000000000000000000, 1.000000000000000000 ) ) ;
#34534=EDGE_LOOP ( 'NONE', ( #33058, #142917, #7618, #134042 ) ) ;
#34541=CARTESIAN_POINT ( 'NONE',  ( 4.858306282870439752, -1.633150327867689988, 6.094999999999989981 ) ) ;
#34566=VECTOR ( 'NONE', #25310, 1000.000000000000000 ) ;
#34575=CARTESIAN_POINT ( 'NONE',  ( 9.603736474768549414, 5.808823158059036373, 5.808823158059032821 ) ) ;
#34583=UNCERTAINTY_MEASURE_WITH_UNIT (LENGTH_MEASURE( 1.000000000000000082E-05 ), #71296, 'distance_accuracy_value', 'NONE');
#34609=( LENGTH_UNIT ( ) NAMED_UNIT ( * ) SI_UNIT ( .MILLI., .METRE. ) );
#34615=CARTESIAN_POINT ( 'NONE',  ( 11.95833333333333393, -3.047499999999997211, -5.278424836066143655 ) ) ;
#34616=CARTESIAN_POINT ( 'NONE',  ( 21.85373647476855297, -5.808823158059035485, -5.808823158059033709 ) ) ;
#34634=FILL_AREA_STYLE_COLOUR ( '', #99756 ) ;
#34638=CARTESIAN_POINT ( 'NONE',  ( 153.4000000000000057, 26.96999999999993847, -34.92499999999998295 ) ) ;
#34639=ADVANCED_FACE ( 'NONE', ( #66681 ), #100022, .T. ) ;
#34650=EDGE_CURVE ( 'NONE', #111873, #65837, #34060, .T. ) ;
#34663=VERTEX_POINT ( 'NONE', #88442 ) ;
#34680=DIRECTION ( 'NONE',  ( -1.000000000000000000, -0.000000000000000000, -0.000000000000000000 ) ) ;
#34751=CARTESIAN_POINT ( 'NONE',  ( 23.40040314143521982, -7.934999999999989839, 2.126176841940957907 ) ) ;
#34777=SURFACE_STYLE_USAGE ( .BOTH. , #136928 ) ;
#34779=VERTEX_POINT ( 'NONE', #81131 ) ;
#34796=CARTESIAN_POINT ( 'NONE',  ( 25.20790314143522082, -6.871911579029513106, -3.967499999999993587 ) ) ;
#34798=CARTESIAN_POINT ( 'NONE',  ( 2.312069808101886004, 7.934999999999992504, 2.126176841940951689 ) ) ;
#34811=VECTOR ( 'NONE', #10972, 1000.000000000000000 ) ;
#34861=CARTESIAN_POINT ( 'NONE',  ( 4.150403141435219823, 7.934999999999988951, -2.126176841940961904 ) ) ;
#34874=FILL_AREA_STYLE_COLOUR ( '', #116920 ) ;
#34885=EDGE_LOOP ( 'NONE', ( #102413, #96004, #100945, #68585 ) ) ;
#34898=STYLED_ITEM ( 'NONE', ( #120687 ), #40939 ) ;
#34904=COLOUR_RGB ( '', 0.66274510, 0.83137255, 0.94901961) ;
#34905=DIRECTION ( 'NONE',  ( 0.000000000000000000, 0.000000000000000000, 1.000000000000000000 ) ) ;
#34926=CARTESIAN_POINT ( 'NONE',  ( 27.04623647476855197, -7.934999999999990727, 4.858786175617117713E-16 ) ) ;
#34948=ADVANCED_FACE ( 'NONE', ( #107964 ), #63807, .T. ) ;
#34958=VERTEX_POINT ( 'NONE', #131911 ) ;
#34991=AXIS2_PLACEMENT_3D ( 'NONE', #21035, #109490, #54428 ) ;
#34994=CARTESIAN_POINT ( 'NONE',  ( 25.40000000000000213, 6.668511817681099352, 3.138890638869527461 ) ) ;
#34998=MECHANICAL_DESIGN_GEOMETRIC_PRESENTATION_REPRESENTATION('',(#69668),#44199);
#35001=SURFACE_STYLE_FILL_AREA ( #98781 ) ;
#35003=CARTESIAN_POINT ( 'NONE',  ( 0.4921764442864913769, 7.017265639291151658, -2.933287722884923898 ) ) ;
#35050=ORIENTED_EDGE ( 'NONE', *, *, #28016, .T. ) ;
#35064=STYLED_ITEM ( 'NONE', ( #46406 ), #65185 ) ;
#35081=EDGE_CURVE ( 'NONE', #32751, #98192, #119216, .T. ) ;
#35107=CARTESIAN_POINT ( 'NONE',  ( 2.983736474768552860, -5.808823158059035485, -5.808823158059033709 ) ) ;
#35118=DIRECTION ( 'NONE',  ( 0.000000000000000000, 0.000000000000000000, 1.000000000000000000 ) ) ;
#35138=ORIENTED_EDGE ( 'NONE', *, *, #100972, .F. ) ;
#35140=SURFACE_STYLE_FILL_AREA ( #58351 ) ;
#35159=DIRECTION ( 'NONE',  ( 0.000000000000000000, -1.000000000000000000, 0.000000000000000000 ) ) ;
#35162=LINE ( 'NONE', #44632, #120603 ) ;
#35258=CARTESIAN_POINT ( 'NONE',  ( 3.837472949537105826, 6.094999999999989981, -1.119633336120465690E-15 ) ) ;
#35259=( GEOMETRIC_REPRESENTATION_CONTEXT ( 3 ) GLOBAL_UNCERTAINTY_ASSIGNED_CONTEXT ( ( #93945 ) ) GLOBAL_UNIT_ASSIGNED_CONTEXT ( ( #44005, #46170, #45455 ) ) REPRESENTATION_CONTEXT ( 'NONE', 'WORKASPACE' ) );
#35260=VECTOR ( 'NONE', #102463, 1000.000000000000000 ) ;
#35266=SURFACE_SIDE_STYLE ('',( #80196 ) ) ;
#35284=CARTESIAN_POINT ( 'NONE',  ( 7.483306282870440640, 6.094999999999991758, 1.633150327867687102 ) ) ;
#35290=DIRECTION ( 'NONE',  ( 0.000000000000000000, 0.000000000000000000, -1.000000000000000000 ) ) ;
#35313=CARTESIAN_POINT ( 'NONE',  ( 21.56206980810188512, -7.934999999999991616, -2.126176841940955242 ) ) ;
#35335=COLOUR_RGB ( '', 0.40784314, 0.44705882, 0.49803922) ;
#35357=CARTESIAN_POINT ( 'NONE',  ( 15.02083333333333570, -6.094999999999989981, -1.633150327867689100 ) ) ;
#35380=SURFACE_SIDE_STYLE ('',( #78873 ) ) ;
#35422=CARTESIAN_POINT ( 'NONE',  ( 25.39999999999999858, 0.000000000000000000, 0.000000000000000000 ) ) ;
#35458=DIRECTION ( 'NONE',  ( 1.000000000000000000, -0.000000000000000000, -0.000000000000000000 ) ) ;
#35472=SURFACE_STYLE_FILL_AREA ( #134780 ) ;
#35494=CARTESIAN_POINT ( 'NONE',  ( 31.27540314143522693, -2.126176841940958351, -7.934999999999989839 ) ) ;
#35511=AXIS2_PLACEMENT_3D ( 'NONE', #124947, #14765, #67766 ) ;
#35519=CARTESIAN_POINT ( 'NONE',  ( 58.16711163708656329, -46.44928942427644358, -35.85226645763125219 ) ) ;
#35539=CARTESIAN_POINT ( 'NONE',  ( 21.56206980810188512, -7.934999999999991616, -2.126176841940955242 ) ) ;
#35587=ORIENTED_EDGE ( 'NONE', *, *, #785, .T. ) ;
#35597=CARTESIAN_POINT ( 'NONE',  ( 1.817069808101886341, -2.126176841940956130, 7.934999999999990727 ) ) ;
#35660=DIRECTION ( 'NONE',  ( 0.000000000000000000, -1.000000000000000000, 0.000000000000000000 ) ) ;
#35663=CARTESIAN_POINT ( 'NONE',  ( 27.48373647476854842, -5.808823158059035485, -5.808823158059033709 ) ) ;
#35707=DIRECTION ( 'NONE',  ( 0.000000000000000000, 0.000000000000000000, 1.000000000000000000 ) ) ;
#35722=CARTESIAN_POINT ( 'NONE',  ( 0.8453006047648484733, -6.493492593015893100, -3.237972208483580694 ) ) ;
#35726=CARTESIAN_POINT ( 'NONE',  ( 25.39999999999998792, 5.550253899293828397, 4.161426631299068646 ) ) ;
#35736=CARTESIAN_POINT ( 'NONE',  ( 1.315494349410903485, 0.8306144699724272717, 6.741090620970949132 ) ) ;
#35764=ORIENTED_EDGE ( 'NONE', *, *, #114337, .F. ) ;
#35828=PRESENTATION_STYLE_ASSIGNMENT (( #115446 ) ) ;
#35832=CARTESIAN_POINT ( 'NONE',  ( 30.37913961620377634, -5.278424836066145431, -3.047499999999993658 ) ) ;
#35896=DIRECTION ( 'NONE',  ( 0.000000000000000000, 0.000000000000000000, 1.000000000000000000 ) ) ;
#35962=ORIENTED_EDGE ( 'NONE', *, *, #99577, .T. ) ;
#35985=CARTESIAN_POINT ( 'NONE',  ( 9.233306282870437087, -6.094999999999989981, -1.633150327867689100 ) ) ;
#36018=CARTESIAN_POINT ( 'NONE',  ( 19.81206980810188156, 7.934999999999993392, 2.126176841940951689 ) ) ;
#36026=ORIENTED_EDGE ( 'NONE', *, *, #36653, .T. ) ;
#36029=UNCERTAINTY_MEASURE_WITH_UNIT (LENGTH_MEASURE( 1.000000000000000082E-05 ), #89960, 'distance_accuracy_value', 'NONE');
#36041=VERTEX_POINT ( 'NONE', #88557 ) ;
#36047=FACE_OUTER_BOUND ( 'NONE', #131310, .T. ) ;
#36062=CARTESIAN_POINT ( 'NONE',  ( 11.52083333333333393, -6.094999999999989981, -1.633150327867689100 ) ) ;
#36075=EDGE_LOOP ( 'NONE', ( #58018, #138690, #19871, #130948, #12366, #28392, #79437, #68239, #119767, #74514, #19024, #141863, #33295, #79184 ) ) ;
#36116=CARTESIAN_POINT ( 'NONE',  ( 24.42123647476855552, -9.717572351234235426E-16, -7.934999999999990727 ) ) ;
#36118=( LENGTH_UNIT ( ) NAMED_UNIT ( * ) SI_UNIT ( .MILLI., .METRE. ) );
#36127=CARTESIAN_POINT ( 'NONE',  ( 9.625000000000001776, 6.094999999999989981, -1.119633336120465690E-15 ) ) ;
#36155=CARTESIAN_POINT ( 'NONE',  ( 55.56056557994608625, -49.14999999999999147, 39.86617647058822200 ) ) ;
#36176=( LENGTH_UNIT ( ) NAMED_UNIT ( * ) SI_UNIT ( .MILLI., .METRE. ) );
#36179=CIRCLE ( 'NONE', #119534, 5.999999999999998224 ) ;
#36180=CARTESIAN_POINT ( 'NONE',  ( 30.98373647476855552, -5.808823158059035485, -5.808823158059033709 ) ) ;
#36202=CARTESIAN_POINT ( 'NONE',  ( 57.48282408946054289, -47.13357697190244266, -36.34567044386321299 ) ) ;
#36211=UNCERTAINTY_MEASURE_WITH_UNIT (LENGTH_MEASURE( 1.000000000000000082E-05 ), #137323, 'distance_accuracy_value', 'NONE');
#36224=CARTESIAN_POINT ( 'NONE',  ( 20.10373647476854941, 5.808823158059036373, 5.808823158059032821 ) ) ;
#36252=CARTESIAN_POINT ( 'NONE',  ( 153.4000000000000057, 26.96999999999993847, 34.92499999999998295 ) ) ;
#36278=( NAMED_UNIT ( * ) SI_UNIT ( $, .STERADIAN. ) SOLID_ANGLE_UNIT ( ) );
#36296=SURFACE_STYLE_FILL_AREA ( #36989 ) ;
#36305=ORIENTED_EDGE ( 'NONE', *, *, #65291, .T. ) ;
#36322=ADVANCED_FACE ( 'NONE', ( #101304 ), #1941, .F. ) ;
#36328=ORIENTED_EDGE ( 'NONE', *, *, #62528, .T. ) ;
#36330=ORIENTED_EDGE ( 'NONE', *, *, #114337, .T. ) ;
#36344=CARTESIAN_POINT ( 'NONE',  ( 26.90040314143521627, -7.934999999999989839, 2.126176841940957907 ) ) ;
#36346=CARTESIAN_POINT ( 'NONE',  ( -0.07876352523144723727, -9.717572351234235426E-16, -7.934999999999990727 ) ) ;
#36349=EDGE_CURVE ( 'NONE', #56532, #23830, #110882, .T. ) ;
#36357=FACE_BOUND ( 'NONE', #59109, .T. ) ;
#36396=CARTESIAN_POINT ( 'NONE',  ( 0.1600000000000009748, -7.113645484598424495, 3.515717980648092045 ) ) ;
#36400=CARTESIAN_POINT ( 'NONE',  ( 25.40000000000002345, 4.454858951346302831, 4.767764854533462326 ) ) ;
#36409=CARTESIAN_POINT ( 'NONE',  ( 1.369639479247480862, 4.811953009385816285E-13, 6.725360520752516891 ) ) ;
#36410=( NAMED_UNIT ( * ) PLANE_ANGLE_UNIT ( ) SI_UNIT ( $, .RADIAN. ) );
#36418=SURFACE_STYLE_FILL_AREA ( #27662 ) ;
#36484=LINE ( 'NONE', #38629, #118789 ) ;
#36508=CARTESIAN_POINT ( 'NONE',  ( -0.9537635252314473622, -7.934999999999990727, 4.858786175617117713E-16 ) ) ;
#36517=EDGE_LOOP ( 'NONE', ( #26361, #16947, #127076, #56074 ) ) ;
#36533=EDGE_CURVE ( 'NONE', #14111, #86570, #27593, .T. ) ;
#36540=CARTESIAN_POINT ( 'NONE',  ( 1.874569808101886226, 6.871911579029510442, -3.967499999999998916 ) ) ;
#36542=STYLED_ITEM ( 'NONE', ( #85514 ), #34948 ) ;
#36562=CARTESIAN_POINT ( 'NONE',  ( 128.6786164994711044, -49.14501756083437556, 40.36361034346624166 ) ) ;
#36565=DIRECTION ( 'NONE',  ( -0.000000000000000000, 1.000000000000000000, -0.000000000000000000 ) ) ;
#36587=VECTOR ( 'NONE', #139390, 1000.000000000000000 ) ;
#36601=ORIENTED_EDGE ( 'NONE', *, *, #13040, .T. ) ;
#36604=DIRECTION ( 'NONE',  ( 0.000000000000000000, 0.000000000000000000, -1.000000000000000000 ) ) ;
#36643=LINE ( 'NONE', #61317, #11297 ) ;
#36647=DIRECTION ( 'NONE',  ( 0.000000000000000000, 0.000000000000000000, 1.000000000000000000 ) ) ;
#36653=EDGE_CURVE ( 'NONE', #65837, #14111, #134111, .T. ) ;
#36661=CARTESIAN_POINT ( 'NONE',  ( 2.379139616203772789, -5.278424836066145431, -3.047499999999993658 ) ) ;
#36695=CARTESIAN_POINT ( 'NONE',  ( 26.95790314143522437, 6.871911579029515771, 3.967499999999989146 ) ) ;
#36705=AXIS2_PLACEMENT_3D ( 'NONE', #94473, #39412, #117629 ) ;
#36739=( NAMED_UNIT ( * ) PLANE_ANGLE_UNIT ( ) SI_UNIT ( $, .RADIAN. ) );
#36744=CARTESIAN_POINT ( 'NONE',  ( 21.00000000000000000, 0.000000000000000000, 6.094999999999989981 ) ) ;
#36768=ORIENTED_EDGE ( 'NONE', *, *, #127323, .F. ) ;
#36797=( GEOMETRIC_REPRESENTATION_CONTEXT ( 3 ) GLOBAL_UNCERTAINTY_ASSIGNED_CONTEXT ( ( #16965 ) ) GLOBAL_UNIT_ASSIGNED_CONTEXT ( ( #43590, #55921, #23240 ) ) REPRESENTATION_CONTEXT ( 'NONE', 'WORKASPACE' ) );
#36804=DIRECTION ( 'NONE',  ( 0.000000000000000000, -1.000000000000000000, 0.000000000000000000 ) ) ;
#36844=( GEOMETRIC_REPRESENTATION_CONTEXT ( 3 ) GLOBAL_UNCERTAINTY_ASSIGNED_CONTEXT ( ( #44989 ) ) GLOBAL_UNIT_ASSIGNED_CONTEXT ( ( #81499, #61198, #120471 ) ) REPRESENTATION_CONTEXT ( 'NONE', 'WORKASPACE' ) );
#36864=CARTESIAN_POINT ( 'NONE',  ( 28.94206980810188767, 7.934999999999993392, 2.126176841940951689 ) ) ;
#36879=EDGE_CURVE ( 'NONE', #117911, #143396, #101780, .T. ) ;
#36898=CARTESIAN_POINT ( 'NONE',  ( 25.39999999999999858, 7.464222240803104598E-16, -6.094999999999989093 ) ) ;
#36910=CARTESIAN_POINT ( 'NONE',  ( 31.47873647476854941, -5.808823158059033709, 5.808823158059035485 ) ) ;
#36911=CARTESIAN_POINT ( 'NONE',  ( 0.9995698081018860037, -3.967499999999998028, -6.871911579029511330 ) ) ;
#36924=SURFACE_STYLE_USAGE ( .BOTH. , #47854 ) ;
#36937=DIRECTION ( 'NONE',  ( -1.000000000000000000, 0.000000000000000000, 0.000000000000000000 ) ) ;
#36989=FILL_AREA_STYLE ('',( #58083 ) ) ;
#36996=CARTESIAN_POINT ( 'NONE',  ( 25.39999999999999858, -14.29000000000013593, -12.70000000000045404 ) ) ;
#37002=ORIENTED_EDGE ( 'NONE', *, *, #7969, .T. ) ;
#37011=SURFACE_STYLE_FILL_AREA ( #58833 ) ;
#37016=PLANE ( 'NONE',  #8749 ) ;
#37020=MECHANICAL_DESIGN_GEOMETRIC_PRESENTATION_REPRESENTATION('',(#4466),#29981);
#37023=DIRECTION ( 'NONE',  ( 0.000000000000000000, 1.000000000000000000, -0.000000000000000000 ) ) ;
#37042=DIRECTION ( 'NONE',  ( -1.000000000000000000, -0.000000000000000000, -0.000000000000000000 ) ) ;
#37044=CARTESIAN_POINT ( 'NONE',  ( 3.275403141435220267, -2.126176841940958351, -7.934999999999989839 ) ) ;
#37048=PRESENTATION_STYLE_ASSIGNMENT (( #92129 ) ) ;
#37071=ORIENTED_EDGE ( 'NONE', *, *, #92566, .F. ) ;
#37102=MECHANICAL_DESIGN_GEOMETRIC_PRESENTATION_REPRESENTATION('',(#108784),#30165);
#37113=CARTESIAN_POINT ( 'NONE',  ( 1.233494112018948430, 2.059985402953470324, 6.548285138816920536 ) ) ;
#37132=EDGE_CURVE ( 'NONE', #65560, #17549, #81023, .T. ) ;
#37178=FILL_AREA_STYLE ('',( #136484 ) ) ;
#37182=CONICAL_SURFACE ( 'NONE', #23287, 2.552699999999928693, 1.029744258676634772 ) ;
#37206=STYLED_ITEM ( 'NONE', ( #31722 ), #64289 ) ;
#37219=CARTESIAN_POINT ( 'NONE',  ( 6.192069808101887674, -7.934999999999991616, -2.126176841940955242 ) ) ;
#37222=VECTOR ( 'NONE', #43586, 1000.000000000000000 ) ;
#37260=CARTESIAN_POINT ( 'NONE',  ( 7.416236474768552966, -7.934999999999990727, 4.858786175617117713E-16 ) ) ;
#37288=CARTESIAN_POINT ( 'NONE',  ( 131.6371832251699914, -49.11905619111313115, 40.21880474160069241 ) ) ;
#37291=UNCERTAINTY_MEASURE_WITH_UNIT (LENGTH_MEASURE( 1.000000000000000082E-05 ), #132329, 'distance_accuracy_value', 'NONE');
#37319=VECTOR ( 'NONE', #52234, 1000.000000000000000 ) ;
#37361=DIRECTION ( 'NONE',  ( -1.000000000000000000, -0.000000000000000000, -0.000000000000000000 ) ) ;
#37377=DIRECTION ( 'NONE',  ( 0.000000000000000000, 0.000000000000000000, -1.000000000000000000 ) ) ;
#37393=VERTEX_POINT ( 'NONE', #103548 ) ;
#37394=CARTESIAN_POINT ( 'NONE',  ( 6.608306282870438864, 1.633150327867687324, -6.094999999999991758 ) ) ;
#37396=ORIENTED_EDGE ( 'NONE', *, *, #24835, .T. ) ;
#37405=DIRECTION ( 'NONE',  ( 0.000000000000000000, 0.000000000000000000, 1.000000000000000000 ) ) ;
#37420=CIRCLE ( 'NONE', #72235, 2.999999999999999112 ) ;
#37421=COLOUR_RGB ( '', 0.40784314, 0.44705882, 0.49803922) ;
#37422=FILL_AREA_STYLE ('',( #104063 ) ) ;
#37428=COLOUR_RGB ( '', 0.66274510, 0.83137255, 0.94901961) ;
#37433=CARTESIAN_POINT ( 'NONE',  ( 21.70790314143522082, -6.871911579029513106, -3.967499999999993587 ) ) ;
#37444=UNCERTAINTY_MEASURE_WITH_UNIT (LENGTH_MEASURE( 1.000000000000000082E-05 ), #33711, 'distance_accuracy_value', 'NONE');
#37485=CARTESIAN_POINT ( 'NONE',  ( 23.77083333333333925, 6.094999999999991758, 1.633150327867687102 ) ) ;
#37565=EDGE_LOOP ( 'NONE', ( #77871, #91436, #57026, #123124 ) ) ;
#37601=ORIENTED_EDGE ( 'NONE', *, *, #66058, .T. ) ;
#37602=CIRCLE ( 'NONE', #5165, 3.000000000000002665 ) ;
#37605=CARTESIAN_POINT ( 'NONE',  ( 27.19206980810188767, -7.934999999999991616, -2.126176841940955242 ) ) ;
#37638=FILL_AREA_STYLE ('',( #4197 ) ) ;
#37646=CARTESIAN_POINT ( 'NONE',  ( 180.4193221990229574, -49.14999999999999147, -40.92499999999998295 ) ) ;
#37647=UNCERTAINTY_MEASURE_WITH_UNIT (LENGTH_MEASURE( 1.000000000000000082E-05 ), #108752, 'distance_accuracy_value', 'NONE');
#37659=CARTESIAN_POINT ( 'NONE',  ( 28.70790314143522437, -6.871911579029513106, -3.967499999999993587 ) ) ;
#37660=CARTESIAN_POINT ( 'NONE',  ( 9.603736474768551190, 5.808823158059035485, 5.808823158059032821 ) ) ;
#37661=CARTESIAN_POINT ( 'NONE',  ( 25.39999999999999858, 0.000000000000000000, 6.094999999999989093 ) ) ;
#37665=MECHANICAL_DESIGN_GEOMETRIC_PRESENTATION_REPRESENTATION('',(#49265),#83931);
#37674=TOROIDAL_SURFACE ( 'NONE', #109463, 25.00000000000002487, 3.000000000000000000 ) ;
#37700=ORIENTED_EDGE ( 'NONE', *, *, #43639, .F. ) ;
#37716=CARTESIAN_POINT ( 'NONE',  ( 0.5045698081018860082, 6.871911579029510442, -3.967499999999998916 ) ) ;
#37717=( LENGTH_UNIT ( ) NAMED_UNIT ( * ) SI_UNIT ( .MILLI., .METRE. ) );
#37726=TOROIDAL_SURFACE ( 'NONE', #51602, 14.45000000000002238, 3.000000000000000000 ) ;
#37741=DIRECTION ( 'NONE',  ( -1.000000000000000000, -0.000000000000000000, -0.000000000000000000 ) ) ;
#37749=PRODUCT_DEFINITION ( 'UNKNOWN', '', #102710, #125624 ) ;
#37765=CIRCLE ( 'NONE', #60976, 3.000000000000000444 ) ;
#37783=CARTESIAN_POINT ( 'NONE',  ( 2.108736474768552860, -5.808823158059033709, 5.808823158059035485 ) ) ;
#37788=SURFACE_SIDE_STYLE ('',( #16722 ) ) ;
#37792=ORIENTED_EDGE ( 'NONE', *, *, #30098, .F. ) ;
#37802=CARTESIAN_POINT ( 'NONE',  ( 183.9019840361162323, -51.74944211519454029, -38.65549799471444459 ) ) ;
#37824=EDGE_LOOP ( 'NONE', ( #39319, #141033, #120352 ) ) ;
#37829=ADVANCED_FACE ( 'NONE', ( #81686 ), #112868, .T. ) ;
#37845=SURFACE_STYLE_USAGE ( .BOTH. , #93636 ) ;
#37857=SURFACE_SIDE_STYLE ('',( #48720 ) ) ;
#37903=EDGE_LOOP ( 'NONE', ( #94816, #61046, #104550, #28533 ) ) ;
#37904=AXIS2_PLACEMENT_3D ( 'NONE', #18000, #75997, #63713 ) ;
#37906=ORIENTED_EDGE ( 'NONE', *, *, #27028, .T. ) ;
#37932=ORIENTED_EDGE ( 'NONE', *, *, #105372, .F. ) ;
#37951=AXIS2_PLACEMENT_3D ( 'NONE', #121153, #47064, #21850 ) ;
#37953=CARTESIAN_POINT ( 'NONE',  ( 7.942069808101886785, 7.934999999999993392, 2.126176841940951689 ) ) ;
#37963=CARTESIAN_POINT ( 'NONE',  ( 11.42080628287044064, 3.047499999999997655, 5.278424836066143655 ) ) ;
#37992=CARTESIAN_POINT ( 'NONE',  ( 5.082903141435219929, 3.967499999999992699, -6.871911579029513994 ) ) ;
#38016=DIRECTION ( 'NONE',  ( -1.000000000000000000, -0.000000000000000000, -0.000000000000000000 ) ) ;
#38077=VECTOR ( 'NONE', #73973, 1000.000000000000227 ) ;
#38087=FILL_AREA_STYLE_COLOUR ( '', #88075 ) ;
#38101=DIRECTION ( 'NONE',  ( -0.000000000000000000, -1.000000000000000000, 0.000000000000000000 ) ) ;
#38107=CARTESIAN_POINT ( 'NONE',  ( 181.1499999999998067, -47.62213595499955687, -36.92499999999996163 ) ) ;
#38119=CARTESIAN_POINT ( 'NONE',  ( 15.50413961620377279, -3.047499999999994547, 5.278424836066145431 ) ) ;
#38125=CYLINDRICAL_SURFACE ( 'NONE', #92768, 3.999999999999996447 ) ;
#38134=ADVANCED_FACE ( 'NONE', ( #124985 ), #136561, .T. ) ;
#38143=DIRECTION ( 'NONE',  ( 0.000000000000000000, 1.000000000000000000, -2.556434596176436916E-15 ) ) ;
#38152=CARTESIAN_POINT ( 'NONE',  ( 18.06206980810188867, -7.934999999999991616, -2.126176841940955242 ) ) ;
#38156=LINE ( 'NONE', #104817, #92973 ) ;
#38168=( BOUNDED_SURFACE ( )  B_SPLINE_SURFACE ( 1, 2, ( 
 ( #33011, #12632, #24244, #68488, #101792, #2455, #50287, #60467, #27083, #115482, #94474, #3863, #6008, #104643, #103906, #81505, #36540, #106046, #61887, #72794, #59059, #93065, #5315, #17615, #26392, #4554, #27802, #116241, #92323, #82918, #138004, #49595, #137295, #72067, #16177, #93778, #80776, #38689, #37992, #47469, #127101, #103210, #16932, #48143, #138724, #61207, #105352, #39413, #91637, #48860, #82222, #124973, #83647, #135859, #37260, #127855, #28536, #116949, #70641, #125711, #25655, #69930, #114102, #14786, #136550, #114783, #15458, #59746, #126393, #71324, #140152, #86484, #74911, #40827, #85741, #42273, #6713, #74173, #50997, #95189, #40148, #141575, #107499, #96585, #139463, #85035, #140826, #129240, #29928, #41519, #118364, #19065, #30680, #63327, #119083, #8161, #129978, #108179, #19773, #51718, #84362, #52398, #62589, #8842, #128552, #29223, #73465, #64010, #117630, #18315, #53103, #97304, #106773, #7452, #95911, #132709, #79769, #123951, #33398, #134844, #102195, #77599, #34088, #68866, #101456, #68179, #44252, #113037, #110878, #11564, #57282, #56590, #89862, #112352, #78298, #89173, #79039, #69584, #58002, #122483, #123244, #36224, #133399, #22445, #88467, #702, #46418, #55844, #90601, #121769, #23918, #35539, #100050, #1407, #113767, #25317, #24612, #12304, #143538, #67437, #13709, #13007, #2104, #2852, #66704, #47152, #44998, #14457, #58736, #23159, #111634, #100755, #91330, #135540, #45692, #134107, #34796, #80451, #124642, #73145, #60864, #126088, #81898, #105714, #72452, #26055, #128228, #15144, #26755, #28905, #117309, #139104, #94840, #17981, #71004, #61565, #94139, #49958, #39807, #49258, #37659, #138377, #105024, #38357, #70317, #114466, #115154, #15828, #28192, #102905, #6374, #4218, #3545, #47842, #92008, #59425, #136225, #103584, #60124, #36910, #81160, #84032, #125366, #48511, #104291, #50650, #39063, #83286, #92713, #93448, #4954, #127497, #5691, #82572, #136948, #137683, #126765, #27447, #116620, #71708, #115874 ),
 ( #16573, #17303, #41192, #108555, #52771, #64384, #131072, #9235, #62986, #32480, #19447, #128920, #31760, #142663, #106412, #109311, #18707, #76720, #87566, #107161, #29595, #20861, #96259, #118005, #7840, #40508, #8522, #53515, #41932, #62257, #129624, #65125, #119447, #74562, #73833, #120148, #131791, #63696, #31063, #75977, #9996, #139837, #96965, #75282, #54260, #120891, #98440, #20144, #86142, #130371, #43355, #52083, #7102, #97720, #118753, #140504, #51378, #95575, #84710, #85399, #30326, #107857, #141972, #141214, #42662, #86863, #1930, #90417, #66537, #57112, #112190, #23734, #67247, #46235, #133927, #89701, #10682, #68006, #111447, #36062, #78851, #33229, #34615, #77438, #123788, #101291, #134664, #12835, #135383, #122304, #12128, #54955, #57821, #80286, #11384, #79603, #99865, #100597, #102011, #55664, #44070, #65860, #22270, #35357, #121602, #24443, #143364, #1240, #68691, #132538, #22979, #91162, #46974, #112880, #33913, #21599, #89017, #13542, #45523, #123059, #2675, #110015, #99119, #88291, #110705, #528, #44827, #133236, #78132, #56414, #82413, #94680, #3383, #50494, #48345, #115695, #138938, #126596, #4061, #103414, #127321, #93979, #47675, #6219, #36744, #92535, #39639, #124475, #17148, #116456, #25147, #136772, #83121, #16395, #71539, #61413, #70836, #59261, #60696, #27286, #59954, #91837, #136061, #37485, #81720, #49806, #69399, #28025, #25875, #113584, #14281, #58567, #102736, #138214, #70146, #125920, #104860, #80985, #137506, #105555, #125191, #26595, #114308, #14985, #114986, #93271, #15665, #104115, #72291, #38899, #5525, #4779, #49082, #38201, #109143, #7676, #85972, #117148, #130931, #107710, #72999, #19981, #64227, #17828, #75128, #42499, #62099, #117848, #9072, #41756, #8366, #128070, #53329, #51214, #95410, #141051, #140349, #30150, #52618, #18534, #29432, #19287, #9829, #54100, #98288, #28752, #142513, #97549, #128756, #51933, #130207, #106257, #96804, #119986, #83866, #129464, #6930, #139674, #20701, #30897, #40354 ) ),
 .UNSPECIFIED., .F., .F., .F. ) 
 B_SPLINE_SURFACE_WITH_KNOTS ( ( 2, 2 ),
 ( 3, 2, 2, 2, 2, 2, 2, 2, 2, 2, 2, 2, 2, 2, 2, 2, 2, 2, 2, 2, 2, 2, 2, 2, 2, 2, 2, 2, 2, 2, 2, 2, 2, 2, 2, 2, 2, 2, 2, 2, 2, 2, 2, 2, 2, 2, 2, 2, 2, 2, 2, 2, 2, 2, 2, 2, 2, 2, 2, 2, 2, 2, 2, 2, 2, 2, 2, 2, 2, 2, 2, 2, 2, 2, 2, 2, 2, 2, 2, 2, 2, 2, 2, 2, 2, 2, 2, 2, 2, 2, 2, 2, 2, 2, 2, 2, 2, 2, 2, 2, 2, 2, 2, 2, 2, 2, 2, 2, 2, 2, 2, 2, 2, 2, 2, 2, 2, 2, 2, 2, 3 ),
 ( 0.000000000000000000, 1.000000000000000000 ),
 ( 0.000000000000000000, 0.008333333333333333218, 0.01666666666666666644, 0.02500000000000000139, 0.03333333333333333287, 0.04166666666666666435, 0.05000000000000000278, 0.05833333333333333426, 0.06666666666666666574, 0.07499999999999999722, 0.08333333333333332871, 0.09166666666666666019, 0.1000000000000000056, 0.1083333333333333370, 0.1166666666666666685, 0.1250000000000000000, 0.1333333333333333315, 0.1416666666666666630, 0.1499999999999999944, 0.1583333333333333259, 0.1666666666666666574, 0.1749999999999999889, 0.1833333333333333204, 0.1916666666666666796, 0.2000000000000000111, 0.2083333333333333426, 0.2166666666666666741, 0.2250000000000000056, 0.2333333333333333370, 0.2416666666666666685, 0.2500000000000000000, 0.2583333333333333592, 0.2666666666666666630, 0.2750000000000000222, 0.2833333333333333259, 0.2916666666666666852, 0.2999999999999999889, 0.3083333333333333481, 0.3166666666666666519, 0.3250000000000000111, 0.3333333333333333148, 0.3416666666666666741, 0.3499999999999999778, 0.3583333333333333370, 0.3666666666666666408, 0.3750000000000000000, 0.3833333333333333592, 0.3916666666666666630, 0.4000000000000000222, 0.4083333333333333259, 0.4166666666666666852, 0.4249999999999999889, 0.4333333333333333481, 0.4416666666666666519, 0.4500000000000000111, 0.4583333333333333148, 0.4666666666666666741, 0.4749999999999999778, 0.4833333333333333370, 0.4916666666666666408, 0.5000000000000000000, 0.5083333333333333037, 0.5166666666666667185, 0.5250000000000000222, 0.5333333333333333259, 0.5416666666666666297, 0.5500000000000000444, 0.5583333333333333481, 0.5666666666666666519, 0.5749999999999999556, 0.5833333333333333703, 0.5916666666666666741, 0.5999999999999999778, 0.6083333333333332815, 0.6166666666666666963, 0.6250000000000000000, 0.6333333333333333037, 0.6416666666666667185, 0.6500000000000000222, 0.6583333333333333259, 0.6666666666666666297, 0.6750000000000000444, 0.6833333333333333481, 0.6916666666666666519, 0.6999999999999999556, 0.7083333333333333703, 0.7166666666666666741, 0.7249999999999999778, 0.7333333333333332815, 0.7416666666666666963, 0.7500000000000000000, 0.7583333333333333037, 0.7666666666666667185, 0.7750000000000000222, 0.7833333333333333259, 0.7916666666666666297, 0.8000000000000000444, 0.8083333333333333481, 0.8166666666666666519, 0.8249999999999999556, 0.8333333333333333703, 0.8416666666666666741, 0.8499999999999999778, 0.8583333333333332815, 0.8666666666666666963, 0.8750000000000000000, 0.8833333333333333037, 0.8916666666666667185, 0.9000000000000000222, 0.9083333333333333259, 0.9166666666666666297, 0.9250000000000000444, 0.9333333333333333481, 0.9416666666666666519, 0.9499999999999999556, 0.9583333333333333703, 0.9666666666666666741, 0.9749999999999999778, 0.9833333333333332815, 0.9916666666666666963, 1.000000000000000000 ),
 .UNSPECIFIED. ) 
 GEOMETRIC_REPRESENTATION_ITEM ( )  RATIONAL_B_SPLINE_SURFACE ( (
 ( 1.000000000000000000, 0.9659258262890683122, 1.000000000000000000, 0.9659258262890683122, 1.000000000000000000, 0.9659258262890683122, 1.000000000000000000, 0.9659258262890683122, 1.000000000000000000, 0.9659258262890683122, 1.000000000000000000, 0.9659258262890683122, 1.000000000000000000, 0.9659258262890683122, 1.000000000000000000, 0.9659258262890683122, 1.000000000000000000, 0.9659258262890683122, 1.000000000000000000, 0.9659258262890683122, 1.000000000000000000, 0.9659258262890683122, 1.000000000000000000, 0.9659258262890683122, 1.000000000000000000, 0.9659258262890683122, 1.000000000000000000, 0.9659258262890683122, 1.000000000000000000, 0.9659258262890683122, 1.000000000000000000, 0.9659258262890683122, 1.000000000000000000, 0.9659258262890683122, 1.000000000000000000, 0.9659258262890683122, 1.000000000000000000, 0.9659258262890683122, 1.000000000000000000, 0.9659258262890683122, 1.000000000000000000, 0.9659258262890683122, 1.000000000000000000, 0.9659258262890683122, 1.000000000000000000, 0.9659258262890683122, 1.000000000000000000, 0.9659258262890683122, 1.000000000000000000, 0.9659258262890683122, 1.000000000000000000, 0.9659258262890683122, 1.000000000000000000, 0.9659258262890683122, 1.000000000000000000, 0.9659258262890683122, 1.000000000000000000, 0.9659258262890683122, 1.000000000000000000, 0.9659258262890683122, 1.000000000000000000, 0.9659258262890683122, 1.000000000000000000, 0.9659258262890683122, 1.000000000000000000, 0.9659258262890683122, 1.000000000000000000, 0.9659258262890683122, 1.000000000000000000, 0.9659258262890683122, 1.000000000000000000, 0.9659258262890683122, 1.000000000000000000, 0.9659258262890683122, 1.000000000000000000, 0.9659258262890683122, 1.000000000000000000, 0.9659258262890683122, 1.000000000000000000, 0.9659258262890683122, 1.000000000000000000, 0.9659258262890683122, 1.000000000000000000, 0.9659258262890683122, 1.000000000000000000, 0.9659258262890683122, 1.000000000000000000, 0.9659258262890683122, 1.000000000000000000, 0.9659258262890683122, 1.000000000000000000, 0.9659258262890683122, 1.000000000000000000, 0.9659258262890683122, 1.000000000000000000, 0.9659258262890683122, 1.000000000000000000, 0.9659258262890683122, 1.000000000000000000, 0.9659258262890683122, 1.000000000000000000, 0.9659258262890683122, 1.000000000000000000, 0.9659258262890683122, 1.000000000000000000, 0.9659258262890683122, 1.000000000000000000, 0.9659258262890683122, 1.000000000000000000, 0.9659258262890683122, 1.000000000000000000, 0.9659258262890683122, 1.000000000000000000, 0.9659258262890683122, 1.000000000000000000, 0.9659258262890683122, 1.000000000000000000, 0.9659258262890683122, 1.000000000000000000, 0.9659258262890683122, 1.000000000000000000, 0.9659258262890683122, 1.000000000000000000, 0.9659258262890683122, 1.000000000000000000, 0.9659258262890683122, 1.000000000000000000, 0.9659258262890683122, 1.000000000000000000, 0.9659258262890683122, 1.000000000000000000, 0.9659258262890683122, 1.000000000000000000, 0.9659258262890683122, 1.000000000000000000, 0.9659258262890683122, 1.000000000000000000, 0.9659258262890683122, 1.000000000000000000, 0.9659258262890683122, 1.000000000000000000, 0.9659258262890683122, 1.000000000000000000, 0.9659258262890683122, 1.000000000000000000, 0.9659258262890683122, 1.000000000000000000, 0.9659258262890683122, 1.000000000000000000, 0.9659258262890683122, 1.000000000000000000, 0.9659258262890683122, 1.000000000000000000, 0.9659258262890683122, 1.000000000000000000, 0.9659258262890683122, 1.000000000000000000, 0.9659258262890683122, 1.000000000000000000, 0.9659258262890683122, 1.000000000000000000, 0.9659258262890683122, 1.000000000000000000, 0.9659258262890683122, 1.000000000000000000, 0.9659258262890683122, 1.000000000000000000, 0.9659258262890683122, 1.000000000000000000, 0.9659258262890683122, 1.000000000000000000, 0.9659258262890683122, 1.000000000000000000, 0.9659258262890683122, 1.000000000000000000, 0.9659258262890683122, 1.000000000000000000, 0.9659258262890683122, 1.000000000000000000, 0.9659258262890683122, 1.000000000000000000, 0.9659258262890683122, 1.000000000000000000, 0.9659258262890683122, 1.000000000000000000, 0.9659258262890683122, 1.000000000000000000, 0.9659258262890683122, 1.000000000000000000, 0.9659258262890683122, 1.000000000000000000, 0.9659258262890683122, 1.000000000000000000, 0.9659258262890683122, 1.000000000000000000, 0.9659258262890683122, 1.000000000000000000, 0.9659258262890683122, 1.000000000000000000, 0.9659258262890683122, 1.000000000000000000, 0.9659258262890683122, 1.000000000000000000, 0.9659258262890683122, 1.000000000000000000, 0.9659258262890683122, 1.000000000000000000, 0.9659258262890683122, 1.000000000000000000, 0.9659258262890683122, 1.000000000000000000, 0.9659258262890683122, 1.000000000000000000, 0.9659258262890683122, 1.000000000000000000, 0.9659258262890683122, 1.000000000000000000, 0.9659258262890683122, 1.000000000000000000, 0.9659258262890683122, 1.000000000000000000, 0.9659258262890683122, 1.000000000000000000, 0.9659258262890683122, 1.000000000000000000, 0.9659258262890683122, 1.000000000000000000, 0.9659258262890683122, 1.000000000000000000, 0.9659258262890683122, 1.000000000000000000, 0.9659258262890683122, 1.000000000000000000, 0.9659258262890683122, 1.000000000000000000, 0.9659258262890683122, 1.000000000000000000, 0.9659258262890683122, 1.000000000000000000, 0.9659258262890683122, 1.000000000000000000),
 ( 1.000000000000000000, 0.9659258262890683122, 1.000000000000000000, 0.9659258262890683122, 1.000000000000000000, 0.9659258262890683122, 1.000000000000000000, 0.9659258262890683122, 1.000000000000000000, 0.9659258262890683122, 1.000000000000000000, 0.9659258262890683122, 1.000000000000000000, 0.9659258262890683122, 1.000000000000000000, 0.9659258262890683122, 1.000000000000000000, 0.9659258262890683122, 1.000000000000000000, 0.9659258262890683122, 1.000000000000000000, 0.9659258262890683122, 1.000000000000000000, 0.9659258262890683122, 1.000000000000000000, 0.9659258262890683122, 1.000000000000000000, 0.9659258262890683122, 1.000000000000000000, 0.9659258262890683122, 1.000000000000000000, 0.9659258262890683122, 1.000000000000000000, 0.9659258262890683122, 1.000000000000000000, 0.9659258262890683122, 1.000000000000000000, 0.9659258262890683122, 1.000000000000000000, 0.9659258262890683122, 1.000000000000000000, 0.9659258262890683122, 1.000000000000000000, 0.9659258262890683122, 1.000000000000000000, 0.9659258262890683122, 1.000000000000000000, 0.9659258262890683122, 1.000000000000000000, 0.9659258262890683122, 1.000000000000000000, 0.9659258262890683122, 1.000000000000000000, 0.9659258262890683122, 1.000000000000000000, 0.9659258262890683122, 1.000000000000000000, 0.9659258262890683122, 1.000000000000000000, 0.9659258262890683122, 1.000000000000000000, 0.9659258262890683122, 1.000000000000000000, 0.9659258262890683122, 1.000000000000000000, 0.9659258262890683122, 1.000000000000000000, 0.9659258262890683122, 1.000000000000000000, 0.9659258262890683122, 1.000000000000000000, 0.9659258262890683122, 1.000000000000000000, 0.9659258262890683122, 1.000000000000000000, 0.9659258262890683122, 1.000000000000000000, 0.9659258262890683122, 1.000000000000000000, 0.9659258262890683122, 1.000000000000000000, 0.9659258262890683122, 1.000000000000000000, 0.9659258262890683122, 1.000000000000000000, 0.9659258262890683122, 1.000000000000000000, 0.9659258262890683122, 1.000000000000000000, 0.9659258262890683122, 1.000000000000000000, 0.9659258262890683122, 1.000000000000000000, 0.9659258262890683122, 1.000000000000000000, 0.9659258262890683122, 1.000000000000000000, 0.9659258262890683122, 1.000000000000000000, 0.9659258262890683122, 1.000000000000000000, 0.9659258262890683122, 1.000000000000000000, 0.9659258262890683122, 1.000000000000000000, 0.9659258262890683122, 1.000000000000000000, 0.9659258262890683122, 1.000000000000000000, 0.9659258262890683122, 1.000000000000000000, 0.9659258262890683122, 1.000000000000000000, 0.9659258262890683122, 1.000000000000000000, 0.9659258262890683122, 1.000000000000000000, 0.9659258262890683122, 1.000000000000000000, 0.9659258262890683122, 1.000000000000000000, 0.9659258262890683122, 1.000000000000000000, 0.9659258262890683122, 1.000000000000000000, 0.9659258262890683122, 1.000000000000000000, 0.9659258262890683122, 1.000000000000000000, 0.9659258262890683122, 1.000000000000000000, 0.9659258262890683122, 1.000000000000000000, 0.9659258262890683122, 1.000000000000000000, 0.9659258262890683122, 1.000000000000000000, 0.9659258262890683122, 1.000000000000000000, 0.9659258262890683122, 1.000000000000000000, 0.9659258262890683122, 1.000000000000000000, 0.9659258262890683122, 1.000000000000000000, 0.9659258262890683122, 1.000000000000000000, 0.9659258262890683122, 1.000000000000000000, 0.9659258262890683122, 1.000000000000000000, 0.9659258262890683122, 1.000000000000000000, 0.9659258262890683122, 1.000000000000000000, 0.9659258262890683122, 1.000000000000000000, 0.9659258262890683122, 1.000000000000000000, 0.9659258262890683122, 1.000000000000000000, 0.9659258262890683122, 1.000000000000000000, 0.9659258262890683122, 1.000000000000000000, 0.9659258262890683122, 1.000000000000000000, 0.9659258262890683122, 1.000000000000000000, 0.9659258262890683122, 1.000000000000000000, 0.9659258262890683122, 1.000000000000000000, 0.9659258262890683122, 1.000000000000000000, 0.9659258262890683122, 1.000000000000000000, 0.9659258262890683122, 1.000000000000000000, 0.9659258262890683122, 1.000000000000000000, 0.9659258262890683122, 1.000000000000000000, 0.9659258262890683122, 1.000000000000000000, 0.9659258262890683122, 1.000000000000000000, 0.9659258262890683122, 1.000000000000000000, 0.9659258262890683122, 1.000000000000000000, 0.9659258262890683122, 1.000000000000000000, 0.9659258262890683122, 1.000000000000000000, 0.9659258262890683122, 1.000000000000000000, 0.9659258262890683122, 1.000000000000000000, 0.9659258262890683122, 1.000000000000000000, 0.9659258262890683122, 1.000000000000000000, 0.9659258262890683122, 1.000000000000000000, 0.9659258262890683122, 1.000000000000000000, 0.9659258262890683122, 1.000000000000000000, 0.9659258262890683122, 1.000000000000000000, 0.9659258262890683122, 1.000000000000000000, 0.9659258262890683122, 1.000000000000000000, 0.9659258262890683122, 1.000000000000000000, 0.9659258262890683122, 1.000000000000000000, 0.9659258262890683122, 1.000000000000000000, 0.9659258262890683122, 1.000000000000000000, 0.9659258262890683122, 1.000000000000000000, 0.9659258262890683122, 1.000000000000000000, 0.9659258262890683122, 1.000000000000000000, 0.9659258262890683122, 1.000000000000000000, 0.9659258262890683122, 1.000000000000000000, 0.9659258262890683122, 1.000000000000000000, 0.9659258262890683122, 1.000000000000000000, 0.9659258262890683122, 1.000000000000000000, 0.9659258262890683122, 1.000000000000000000) ) ) 
 REPRESENTATION_ITEM ( '' )  SURFACE ( )  );
#38187=FILL_AREA_STYLE_COLOUR ( '', #42092 ) ;
#38201=CARTESIAN_POINT ( 'NONE',  ( 28.14583333333333570, -1.633150327867689988, 6.094999999999989981 ) ) ;
#38216=ORIENTED_EDGE ( 'NONE', *, *, #121722, .F. ) ;
#38218=CARTESIAN_POINT ( 'NONE',  ( 1.783126656679975719, -5.054327988459295540, 3.799291974498469227 ) ) ;
#38236=LINE ( 'NONE', #6255, #10808 ) ;
#38247=DIRECTION ( 'NONE',  ( 0.000000000000000000, 0.000000000000000000, 1.000000000000000000 ) ) ;
#38314=CARTESIAN_POINT ( 'NONE',  ( 31.42123647476855552, -9.717572351234235426E-16, -7.934999999999990727 ) ) ;
#38336=CARTESIAN_POINT ( 'NONE',  ( 55.56056557994602940, -52.00875322212549889, -39.86617647058820069 ) ) ;
#38357=CARTESIAN_POINT ( 'NONE',  ( 29.14540314143522437, -2.126176841940958351, -7.934999999999989839 ) ) ;
#38358=CARTESIAN_POINT ( 'NONE',  ( 7.124569808101886892, -6.871911579029512218, 3.967499999999996252 ) ) ;
#38370=CARTESIAN_POINT ( 'NONE',  ( 22.35830628287043709, -1.633150327867709528, 6.094999999999979323 ) ) ;
#38386=SURFACE_STYLE_USAGE ( .BOTH. , #136258 ) ;
#38405=( NAMED_UNIT ( * ) PLANE_ANGLE_UNIT ( ) SI_UNIT ( $, .RADIAN. ) );
#38407=EDGE_CURVE ( 'NONE', #91284, #9588, #13548, .T. ) ;
#38414=CARTESIAN_POINT ( 'NONE',  ( 4.879569808101885897, 3.967499999999998916, 6.871911579029510442 ) ) ;
#38425=ORIENTED_EDGE ( 'NONE', *, *, #116212, .F. ) ;
#38434=( NAMED_UNIT ( * ) PLANE_ANGLE_UNIT ( ) SI_UNIT ( $, .RADIAN. ) );
#38435=FACE_OUTER_BOUND ( 'NONE', #141260, .T. ) ;
#38436=ORIENTED_EDGE ( 'NONE', *, *, #91940, .T. ) ;
#38443=PRESENTATION_STYLE_ASSIGNMENT (( #15917 ) ) ;
#38454=PRESENTATION_STYLE_ASSIGNMENT (( #27545 ) ) ;
#38457=DIRECTION ( 'NONE',  ( 0.000000000000000000, -1.000000000000000000, 0.000000000000000000 ) ) ;
#38462=STYLED_ITEM ( 'NONE', ( #49625 ), #33428 ) ;
#38483=CARTESIAN_POINT ( 'NONE',  ( 1.525403141435219379, 2.126176841940962348, 7.934999999999989839 ) ) ;
#38495=SURFACE_STYLE_USAGE ( .BOTH. , #137819 ) ;
#38499=CARTESIAN_POINT ( 'NONE',  ( 184.0378153480262711, -51.37040454773214293, -37.49526731630776055 ) ) ;
#38516=( NAMED_UNIT ( * ) SI_UNIT ( $, .STERADIAN. ) SOLID_ANGLE_UNIT ( ) );
#38522=CARTESIAN_POINT ( 'NONE',  ( 2.021013337047029346, 2.847195794450450457, -5.394070523059989242 ) ) ;
#38540=DIRECTION ( 'NONE',  ( 0.000000000000000000, 0.000000000000000000, -1.000000000000000000 ) ) ;
#38548=ORIENTED_EDGE ( 'NONE', *, *, #123410, .T. ) ;
#38611=EDGE_CURVE ( 'NONE', #56532, #143089, #98603, .T. ) ;
#38615=( NAMED_UNIT ( * ) SI_UNIT ( $, .STERADIAN. ) SOLID_ANGLE_UNIT ( ) );
#38629=CARTESIAN_POINT ( 'NONE',  ( 174.7500000000000000, 7.919999999999947526, -16.42230000000009227 ) ) ;
#38632=CARTESIAN_POINT ( 'NONE',  ( 25.39999999999999858, 7.796566843815467607, 1.475727091950665537 ) ) ;
#38635=CARTESIAN_POINT ( 'NONE',  ( 16.77083333333333570, 6.094999999999991758, 1.633150327867686880 ) ) ;
#38639=MECHANICAL_DESIGN_GEOMETRIC_PRESENTATION_REPRESENTATION('',(#101126),#3809);
#38654=CARTESIAN_POINT ( 'NONE',  ( 7.504569808101886785, 6.871911579029510442, -3.967499999999998916 ) ) ;
#38664=CARTESIAN_POINT ( 'NONE',  ( 10.39997294953710494, 4.461849672132297329, -4.461849672132302658 ) ) ;
#38679=COLOUR_RGB ( '', 0.66274510, 0.83137255, 0.94901961) ;
#38689=CARTESIAN_POINT ( 'NONE',  ( 4.937069808101886892, 2.126176841940952134, -7.934999999999993392 ) ) ;
#38703=( LENGTH_UNIT ( ) NAMED_UNIT ( * ) SI_UNIT ( .MILLI., .METRE. ) );
#38716=CARTESIAN_POINT ( 'NONE',  ( 1.720058664033062845, 0.4644975210628944362, -6.362334081593164825 ) ) ;
#38718=UNCERTAINTY_MEASURE_WITH_UNIT (LENGTH_MEASURE( 1.000000000000000082E-05 ), #75788, 'distance_accuracy_value', 'NONE');
#38732=( GEOMETRIC_REPRESENTATION_CONTEXT ( 3 ) GLOBAL_UNCERTAINTY_ASSIGNED_CONTEXT ( ( #94307 ) ) GLOBAL_UNIT_ASSIGNED_CONTEXT ( ( #16617, #117343, #106455 ) ) REPRESENTATION_CONTEXT ( 'NONE', 'WORKASPACE' ) );
#38752=EDGE_CURVE ( 'NONE', #125982, #56501, #113091, .T. ) ;
#38776=CARTESIAN_POINT ( 'NONE',  ( 27.99999999999999645, -57.14999999999999147, -49.92499999999968452 ) ) ;
#38777=( GEOMETRIC_REPRESENTATION_CONTEXT ( 3 ) GLOBAL_UNCERTAINTY_ASSIGNED_CONTEXT ( ( #127284 ) ) GLOBAL_UNIT_ASSIGNED_CONTEXT ( ( #7776, #41865, #109958 ) ) REPRESENTATION_CONTEXT ( 'NONE', 'WORKASPACE' ) );
#38783=DIRECTION ( 'NONE',  ( 0.000000000000000000, -0.000000000000000000, 1.000000000000000000 ) ) ;
#38787=FACE_OUTER_BOUND ( 'NONE', #132131, .T. ) ;
#38806=DIRECTION ( 'NONE',  ( -1.000000000000000000, -0.000000000000000000, 0.000000000000000000 ) ) ;
#38824=CARTESIAN_POINT ( 'NONE',  ( 20.02497294953710849, -4.461849672132299993, -4.461849672132299105 ) ) ;
#38852=CARTESIAN_POINT ( 'NONE',  ( 27.68706980810188867, -2.126176841940956130, 7.934999999999991616 ) ) ;
#38866=CARTESIAN_POINT ( 'NONE',  ( 3.100164867289006754, -48.63026969829200397, -38.45492102172624271 ) ) ;
#38870=AXIS2_PLACEMENT_3D ( 'NONE', #126274, #1597, #67646 ) ;
#38877=AXIS2_PLACEMENT_3D ( 'NONE', #130141, #21369, #19917 ) ;
#38894=CYLINDRICAL_SURFACE ( 'NONE', #138668, 5.999999999999998224 ) ;
#38899=CARTESIAN_POINT ( 'NONE',  ( 27.56249999999999645, 4.461849672132300881, 4.461849672132299105 ) ) ;
#38923=CARTESIAN_POINT ( 'NONE',  ( 1.703100290951983453, -4.351279483125353842, 4.685986356884224158 ) ) ;
#38934=ORIENTED_EDGE ( 'NONE', *, *, #46934, .F. ) ;
#38940=EDGE_CURVE ( 'NONE', #63172, #2777, #60127, .T. ) ;
#38963=( LENGTH_UNIT ( ) NAMED_UNIT ( * ) SI_UNIT ( .MILLI., .METRE. ) );
#38984=ORIENTED_EDGE ( 'NONE', *, *, #112952, .F. ) ;
#38988=EDGE_CURVE ( 'NONE', #98192, #112966, #128231, .T. ) ;
#39003=FACE_OUTER_BOUND ( 'NONE', #124386, .T. ) ;
#39018=CARTESIAN_POINT ( 'NONE',  ( 0.5620698081018861147, -7.934999999999991616, -2.126176841940955242 ) ) ;
#39020=CARTESIAN_POINT ( 'NONE',  ( 152.4000000000000057, -16.48000000000005016, 33.92499999999998295 ) ) ;
#39029=( LENGTH_UNIT ( ) NAMED_UNIT ( * ) SI_UNIT ( .MILLI., .METRE. ) );
#39040=EDGE_CURVE ( 'NONE', #98192, #121495, #77748, .T. ) ;
#39050=UNCERTAINTY_MEASURE_WITH_UNIT (LENGTH_MEASURE( 1.000000000000000082E-05 ), #19662, 'distance_accuracy_value', 'NONE');
#39063=CARTESIAN_POINT ( 'NONE',  ( 32.49956980810188867, -3.967499999999998028, -6.871911579029511330 ) ) ;
#39064=CARTESIAN_POINT ( 'NONE',  ( 9.020403141435219041, 7.934999999999988951, -2.126176841940961904 ) ) ;
#39082=( GEOMETRIC_REPRESENTATION_CONTEXT ( 3 ) GLOBAL_UNCERTAINTY_ASSIGNED_CONTEXT ( ( #107151 ) ) GLOBAL_UNIT_ASSIGNED_CONTEXT ( ( #51634, #127765, #140075 ) ) REPRESENTATION_CONTEXT ( 'NONE', 'WORKASPACE' ) );
#39084=DIRECTION ( 'NONE',  ( -1.504632769052527134E-30, -3.469446951953615372E-15, -1.000000000000000000 ) ) ;
#39130=CARTESIAN_POINT ( 'NONE',  ( 8.087903141435219823, 6.871911579029515771, 3.967499999999989146 ) ) ;
#39178=STYLED_ITEM ( 'NONE', ( #79101 ), #975 ) ;
#39197=CARTESIAN_POINT ( 'NONE',  ( 1.233736474768552860, 5.808823158059036373, 5.808823158059032821 ) ) ;
#39201=FILL_AREA_STYLE ('',( #117437 ) ) ;
#39202=( NAMED_UNIT ( * ) SI_UNIT ( $, .STERADIAN. ) SOLID_ANGLE_UNIT ( ) );
#39208=PRESENTATION_STYLE_ASSIGNMENT (( #38495 ) ) ;
#39210=CARTESIAN_POINT ( 'NONE',  ( 52.60764783923754351, -49.05583548141699168, -39.86617647058817937 ) ) ;
#39247=CARTESIAN_POINT ( 'NONE',  ( 2.041666666666666963, 3.047499999999993214, -5.278424836066146320 ) ) ;
#39249=MECHANICAL_DESIGN_GEOMETRIC_PRESENTATION_REPRESENTATION('',(#64698),#29902);
#39268=CYLINDRICAL_SURFACE ( 'NONE', #65020, 5.999999999999998224 ) ;
#39291=FACE_OUTER_BOUND ( 'NONE', #20761, .T. ) ;
#39319=ORIENTED_EDGE ( 'NONE', *, *, #129266, .F. ) ;
#39328=ORIENTED_EDGE ( 'NONE', *, *, #102135, .F. ) ;
#39358=SURFACE_STYLE_FILL_AREA ( #140098 ) ;
#39365=CARTESIAN_POINT ( 'NONE',  ( 16.33333333333333570, 5.278424836066143655, -3.047499999999997655 ) ) ;
#39379=DIRECTION ( 'NONE',  ( -1.000000000000000000, -8.828454896530885185E-16, 0.000000000000000000 ) ) ;
#39381=CARTESIAN_POINT ( 'NONE',  ( 11.73373647476855197, 5.808823158059036373, 5.808823158059032821 ) ) ;
#39412=DIRECTION ( 'NONE',  ( -1.000000000000000000, -0.000000000000000000, -0.000000000000000000 ) ) ;
#39413=CARTESIAN_POINT ( 'NONE',  ( 6.395403141435219929, 2.126176841940962348, 7.934999999999989839 ) ) ;
#39420=ORIENTED_EDGE ( 'NONE', *, *, #27117, .F. ) ;
#39430=CARTESIAN_POINT ( 'NONE',  ( 184.1499999999998636, -50.24077216217758490, -35.40405119785167898 ) ) ;
#39446=SURFACE_SIDE_STYLE ('',( #5340 ) ) ;
#39459=ORIENTED_EDGE ( 'NONE', *, *, #50219, .T. ) ;
#39499=ORIENTED_EDGE ( 'NONE', *, *, #47686, .F. ) ;
#39501=CIRCLE ( 'NONE', #111276, 3.999999999999996447 ) ;
#39539=CARTESIAN_POINT ( 'NONE',  ( 180.6620941962882227, -49.11927476322659203, -40.22110306067541075 ) ) ;
#39554=CARTESIAN_POINT ( 'NONE',  ( 14.33747294953710494, 6.094999999999989981, -1.119633336120465690E-15 ) ) ;
#39585=CARTESIAN_POINT ( 'NONE',  ( 27.83290314143522437, -3.967499999999994476, 6.871911579029513106 ) ) ;
#39599=CARTESIAN_POINT ( 'NONE',  ( 0.3339215173231541711, -51.89584459748878942, -39.24672819827818415 ) ) ;
#39622=EDGE_CURVE ( 'NONE', #70428, #62641, #105989, .T. ) ;
#39628=CYLINDRICAL_SURFACE ( 'NONE', #12040, 1.000000000000000888 ) ;
#39630=CARTESIAN_POINT ( 'NONE',  ( 176.2838169021916599, 7.919999999999943086, 19.12499999999998224 ) ) ;
#39639=CARTESIAN_POINT ( 'NONE',  ( 21.29166666666666785, -3.047499999999994547, 5.278424836066145431 ) ) ;
#39652=CARTESIAN_POINT ( 'NONE',  ( 122.6835989386367771, -57.15000000000008384, -34.92499999999998295 ) ) ;
#39706=CARTESIAN_POINT ( 'NONE',  ( 26.40000000000000568, -18.48000000000005372, 33.92499999999998295 ) ) ;
#39716=CARTESIAN_POINT ( 'NONE',  ( 25.39999999999999858, -2.600000000000012523, -20.40202195861969159 ) ) ;
#39731=ADVANCED_FACE ( 'NONE', ( #62458 ), #74038, .T. ) ;
#39759=CARTESIAN_POINT ( 'NONE',  ( 0.1245698081018860176, -6.871911579029512218, 3.967499999999996252 ) ) ;
#39768=DIRECTION ( 'NONE',  ( -0.000000000000000000, 1.000000000000000000, -0.000000000000000000 ) ) ;
#39786=EDGE_LOOP ( 'NONE', ( #112421, #141220, #63614 ) ) ;
#39788=CARTESIAN_POINT ( 'NONE',  ( 55.64345981607718983, -48.97294124528584547, -39.12804664298375457 ) ) ;
#39796=CARTESIAN_POINT ( 'NONE',  ( 149.2199999999997999, -3.180000000000061444, 31.92499999999998295 ) ) ;
#39807=CARTESIAN_POINT ( 'NONE',  ( 28.41623647476855652, -7.934999999999990727, 4.858786175617117713E-16 ) ) ;
#39808=CARTESIAN_POINT ( 'NONE',  ( 12.37456980810188512, 6.871911579029510442, -3.967499999999998916 ) ) ;
#39826=MECHANICAL_DESIGN_GEOMETRIC_PRESENTATION_REPRESENTATION('',(#90725),#14333);
#39830=DIRECTION ( 'NONE',  ( 0.000000000000000000, 1.000000000000000000, -3.469446951953614189E-15 ) ) ;
#39840=CARTESIAN_POINT ( 'NONE',  ( 60.76962477604072177, -44.19516442796815170, 34.92499999999998295 ) ) ;
#39867=CARTESIAN_POINT ( 'NONE',  ( 6.046236474768552860, -7.934999999999990727, 4.858786175617117713E-16 ) ) ;
#39892=CARTESIAN_POINT ( 'NONE',  ( 25.40000000000000568, 1.328209827113943309, -7.833578357555276206 ) ) ;
#39905=( NAMED_UNIT ( * ) PLANE_ANGLE_UNIT ( ) SI_UNIT ( $, .RADIAN. ) );
#39940=CARTESIAN_POINT ( 'NONE',  ( 8.671236474768553748, 0.000000000000000000, 7.934999999999990727 ) ) ;
#39943=CARTESIAN_POINT ( 'NONE',  ( 25.39999999999999858, -14.29000000000013593, -12.70000000000045404 ) ) ;
#39953=CARTESIAN_POINT ( 'NONE',  ( 183.8160784826766587, -51.89584459748878942, -39.24672819827820547 ) ) ;
#39957=EDGE_CURVE ( 'NONE', #65885, #29858, #3666, .T. ) ;
#40037=STYLED_ITEM ( 'NONE', ( #51677 ), #131194 ) ;
#40052=EDGE_LOOP ( 'NONE', ( #134540, #105259, #97671, #72977, #73560, #2168, #64447 ) ) ;
#40112=CARTESIAN_POINT ( 'NONE',  ( 13.48373647476855375, -5.808823158059035485, -5.808823158059033709 ) ) ;
#40121=ORIENTED_EDGE ( 'NONE', *, *, #3601, .T. ) ;
#40148=CARTESIAN_POINT ( 'NONE',  ( 11.20790314143521904, -6.871911579029513106, -3.967499999999993587 ) ) ;
#40169=DIRECTION ( 'NONE',  ( 0.000000000000000000, 1.000000000000000000, 1.365923996832126925E-16 ) ) ;
#40204=PRESENTATION_STYLE_ASSIGNMENT (( #116296 ) ) ;
#40207=EDGE_CURVE ( 'NONE', #15118, #134245, #26782, .T. ) ;
#40262=( NAMED_UNIT ( * ) PLANE_ANGLE_UNIT ( ) SI_UNIT ( $, .RADIAN. ) );
#40279=CARTESIAN_POINT ( 'NONE',  ( 18.42080628287044064, 3.047499999999997655, 5.278424836066143655 ) ) ;
#40289=SHAPE_REPRESENTATION ( '1.0 Base', ( #127880 ), #141741 ) ;
#40354=CARTESIAN_POINT ( 'NONE',  ( 35.00000000000000000, 0.000000000000000000, 6.094999999999989981 ) ) ;
#40376=CARTESIAN_POINT ( 'NONE',  ( 12.54166666666666785, 3.047499999999993214, -5.278424836066146320 ) ) ;
#40378=CARTESIAN_POINT ( 'NONE',  ( 1.624181887823187953, -3.508773871178531234, 5.449882146574780428 ) ) ;
#40400=CARTESIAN_POINT ( 'NONE',  ( 25.40000000000000568, -5.651140751524227568, -5.186583730001445680 ) ) ;
#40402=CARTESIAN_POINT ( 'NONE',  ( 181.1499999999998067, -47.62213595499955687, -36.92499999999996163 ) ) ;
#40407=VERTEX_POINT ( 'NONE', #1268 ) ;
#40411=CARTESIAN_POINT ( 'NONE',  ( 180.5530070941967438, -49.14999999999999147, 40.56450646617377487 ) ) ;
#40414=DIRECTION ( 'NONE',  ( 0.000000000000000000, 0.000000000000000000, -1.000000000000000000 ) ) ;
#40415=DIRECTION ( 'NONE',  ( -1.000000000000000000, -0.000000000000000000, -0.000000000000000000 ) ) ;
#40417=CARTESIAN_POINT ( 'NONE',  ( 24.39999999999999858, -5.520864266206504263E-14, -33.92499999999998295 ) ) ;
#40436=ORIENTED_EDGE ( 'NONE', *, *, #81815, .T. ) ;
#40439=AXIS2_PLACEMENT_3D ( 'NONE', #2879, #102927, #36937 ) ;
#40465=CARTESIAN_POINT ( 'NONE',  ( 3.298144211979590068, -48.98056306480232536, 39.49745726092411502 ) ) ;
#40470=CARTESIAN_POINT ( 'NONE',  ( 3.041236474768552966, 0.000000000000000000, 7.934999999999990727 ) ) ;
#40479=CARTESIAN_POINT ( 'NONE',  ( 55.18164086290596515, -52.14999999999999147, -41.64500000000001023 ) ) ;
#40496=EDGE_CURVE ( 'NONE', #113523, #48370, #67973, .T. ) ;
#40508=CARTESIAN_POINT ( 'NONE',  ( 3.645833333333333037, -1.633150327867689988, 6.094999999999989981 ) ) ;
#40509=CARTESIAN_POINT ( 'NONE',  ( 12.08290314143522082, 3.967499999999992699, -6.871911579029513994 ) ) ;
#40521=CARTESIAN_POINT ( 'NONE',  ( 28.00000000000002487, -52.14999999999999147, 62.92500000000006111 ) ) ;
#40536=CARTESIAN_POINT ( 'NONE',  ( 60.59549430336050335, -44.02090675802819675, 34.92500000000511307 ) ) ;
#40543=CARTESIAN_POINT ( 'NONE',  ( 127.6984665281585762, -50.67230138428261910, 37.61253110040533443 ) ) ;
#40563=CARTESIAN_POINT ( 'NONE',  ( 6.921236474768553748, -9.717572351234235426E-16, -7.934999999999990727 ) ) ;
#40564=CARTESIAN_POINT ( 'NONE',  ( 22.31250000000000000, -4.461849672132299993, -4.461849672132299105 ) ) ;
#40579=EDGE_CURVE ( 'NONE', #20435, #19025, #47237, .T. ) ;
#40582=CARTESIAN_POINT ( 'NONE',  ( 5.687500000000000000, 4.461849672132297329, -4.461849672132302658 ) ) ;
#40622=DIRECTION ( 'NONE',  ( 1.000000000000000000, 0.000000000000000000, 0.000000000000000000 ) ) ;
#40634=CARTESIAN_POINT ( 'NONE',  ( 8.233736474768550195, 5.808823158059036373, 5.808823158059032821 ) ) ;
#40669=CARTESIAN_POINT ( 'NONE',  ( 0.1600000000000005584, -7.937054096915820089, 0.2840606438466312111 ) ) ;
#40703=FILL_AREA_STYLE_COLOUR ( '', #33846 ) ;
#40750=ORIENTED_EDGE ( 'NONE', *, *, #2153, .F. ) ;
#40799=CARTESIAN_POINT ( 'NONE',  ( 17.12956980810188767, -3.967499999999998028, -6.871911579029511330 ) ) ;
#40817=ORIENTED_EDGE ( 'NONE', *, *, #107580, .F. ) ;
#40827=CARTESIAN_POINT ( 'NONE',  ( 10.18706980810188689, -2.126176841940956130, 7.934999999999991616 ) ) ;
#40841=FACE_OUTER_BOUND ( 'NONE', #49764, .T. ) ;
#40843=COLOUR_RGB ( '', 0.66274510, 0.83137255, 0.94901961) ;
#40853=CARTESIAN_POINT ( 'NONE',  ( 128.9683591370937847, -52.14999999999999147, 41.64499999999998181 ) ) ;
#40862=CIRCLE ( 'NONE', #15364, 3.000000000000002220 ) ;
#40888=CARTESIAN_POINT ( 'NONE',  ( 25.39999999999999858, -30.18000000000009564, 15.92499999999935945 ) ) ;
#40890=( NAMED_UNIT ( * ) PLANE_ANGLE_UNIT ( ) SI_UNIT ( $, .RADIAN. ) );
#40912=PRESENTATION_STYLE_ASSIGNMENT (( #51802 ) ) ;
#40922=EDGE_CURVE ( 'NONE', #96698, #98296, #75793, .T. ) ;
#40939=ADVANCED_FACE ( 'NONE', ( #54067 ), #89508, .F. ) ;
#40948=SURFACE_STYLE_FILL_AREA ( #32217 ) ;
#40963=STYLED_ITEM ( 'NONE', ( #99134 ), #109467 ) ;
#40964=CARTESIAN_POINT ( 'NONE',  ( 23.81663961620377279, -1.633150327867691987, -6.094999999999989093 ) ) ;
#40995=CARTESIAN_POINT ( 'NONE',  ( 29.14540314143522437, -2.126176841940958351, -7.934999999999989839 ) ) ;
#41005=( NAMED_UNIT ( * ) PLANE_ANGLE_UNIT ( ) SI_UNIT ( $, .RADIAN. ) );
#41010=LINE ( 'NONE', #30121, #4971 ) ;
#41038=ADVANCED_FACE ( 'NONE', ( #47487 ), #15477, .T. ) ;
#41087=FILL_AREA_STYLE ('',( #129507 ) ) ;
#41094=( GEOMETRIC_REPRESENTATION_CONTEXT ( 3 ) GLOBAL_UNCERTAINTY_ASSIGNED_CONTEXT ( ( #47827 ) ) GLOBAL_UNIT_ASSIGNED_CONTEXT ( ( #12277, #113011, #132682 ) ) REPRESENTATION_CONTEXT ( 'NONE', 'WORKASPACE' ) );
#41100=CARTESIAN_POINT ( 'NONE',  ( 181.0498351327038620, -48.63026969829178370, 38.45492102172562454 ) ) ;
#41102=DIRECTION ( 'NONE',  ( -1.000000000000000000, 0.000000000000000000, 0.000000000000000000 ) ) ;
#41150=CARTESIAN_POINT ( 'NONE',  ( 0.000000000000000000, -47.62213595499959951, 36.92500000000000426 ) ) ;
#41152=CARTESIAN_POINT ( 'NONE',  ( 4.791236474768552966, -9.717572351234235426E-16, -7.934999999999990727 ) ) ;
#41175=CARTESIAN_POINT ( 'NONE',  ( 53.94409967708044462, -48.16486758952232350, -37.61253110040615866 ) ) ;
#41190=EDGE_CURVE ( 'NONE', #62041, #62992, #17632, .T. ) ;
#41192=CARTESIAN_POINT ( 'NONE',  ( 0.2916666666666667407, -3.047499999999994547, 5.278424836066145431 ) ) ;
#41193=CARTESIAN_POINT ( 'NONE',  ( 18.35373647476854941, -5.808823158059035485, -5.808823158059033709 ) ) ;
#41202=ADVANCED_FACE ( 'NONE', ( #40841 ), #107514, .T. ) ;
#41214=CARTESIAN_POINT ( 'NONE',  ( 0.8183591370940056509, -52.14999999999999147, 41.64499999999997470 ) ) ;
#41229=CARTESIAN_POINT ( 'NONE',  ( 125.9828883629226510, -46.44928942427174690, 35.85226645762418229 ) ) ;
#41247=CARTESIAN_POINT ( 'NONE',  ( 6.192069808101886785, -7.934999999999990727, -2.126176841940955242 ) ) ;
#41258=CARTESIAN_POINT ( 'NONE',  ( 18.66666666666666785, -5.278424836066145431, -3.047499999999993658 ) ) ;
#41274=CARTESIAN_POINT ( 'NONE',  ( 25.40000000000000568, 0.1175040200531159013, -7.944505609933036006 ) ) ;
#41314=CARTESIAN_POINT ( 'NONE',  ( 13.19206980810188412, -7.934999999999991616, -2.126176841940955242 ) ) ;
#41336=CIRCLE ( 'NONE', #41441, 3.999999999999989786 ) ;
#41355=CARTESIAN_POINT ( 'NONE',  ( 0.1600000000000024458, -7.674647425206645224, -2.043597544210264072 ) ) ;
#41363=COLOUR_RGB ( '', 0.72549020, 0.75294118, 0.79215686) ;
#41391=FILL_AREA_STYLE ('',( #42140 ) ) ;
#41410=CARTESIAN_POINT ( 'NONE',  ( 26.40000000000000568, -18.48000000000005372, -33.92499999999998295 ) ) ;
#41429=EDGE_CURVE ( 'NONE', #45858, #69422, #127602, .T. ) ;
#41441=AXIS2_PLACEMENT_3D ( 'NONE', #121562, #31019, #486 ) ;
#41443=CARTESIAN_POINT ( 'NONE',  ( 174.7500000000000000, 7.919999999999947526, 19.12499999999998224 ) ) ;
#41491=CARTESIAN_POINT ( 'NONE',  ( 21.94206980810188057, 7.934999999999993392, 2.126176841940951689 ) ) ;
#41519=CARTESIAN_POINT ( 'NONE',  ( 12.52040314143522082, 7.934999999999989839, -2.126176841940961904 ) ) ;
#41551=LINE ( 'NONE', #142329, #111318 ) ;
#41669=CARTESIAN_POINT ( 'NONE',  ( 28.77497294953710849, 4.461849672132300881, 4.461849672132299105 ) ) ;
#41693=ADVANCED_FACE ( 'NONE', ( #43959 ), #57707, .F. ) ;
#41707=CARTESIAN_POINT ( 'NONE',  ( 28.12456980810188867, -6.871911579029512218, 3.967499999999996252 ) ) ;
#41715=CARTESIAN_POINT ( 'NONE',  ( 55.18164086290604331, -49.14999999999998437, 41.64499999999997470 ) ) ;
#41720=CARTESIAN_POINT ( 'NONE',  ( 0.3619179557531525537, -48.99280962439294740, -39.49606053969947084 ) ) ;
#41746=UNCERTAINTY_MEASURE_WITH_UNIT (LENGTH_MEASURE( 1.000000000000000082E-05 ), #93581, 'distance_accuracy_value', 'NONE');
#41756=CARTESIAN_POINT ( 'NONE',  ( 30.47916666666666430, 6.094999999999988205, -1.633150327867694651 ) ) ;
#41770=COLOUR_RGB ( '', 0.31764706, 0.68627451, 0.89019608) ;
#41779=CARTESIAN_POINT ( 'NONE',  ( 131.7497271887055490, -49.14999999999999147, -40.57187971031610374 ) ) ;
#41803=CIRCLE ( 'NONE', #125095, 4.999999999999997335 ) ;
#41807=STYLED_ITEM ( 'NONE', ( #104080 ), #81930 ) ;
#41819=CARTESIAN_POINT ( 'NONE',  ( 183.8160784826765735, -51.89584459748879652, 39.24672819827913628 ) ) ;
#41826=ADVANCED_FACE ( 'NONE', ( #38787 ), #64905, .T. ) ;
#41827=DIRECTION ( 'NONE',  ( -1.000000000000000000, 0.000000000000000000, 0.000000000000000000 ) ) ;
#41849=SURFACE_STYLE_USAGE ( .BOTH. , #141140 ) ;
#41865=( NAMED_UNIT ( * ) PLANE_ANGLE_UNIT ( ) SI_UNIT ( $, .RADIAN. ) );
#41873=AXIS2_PLACEMENT_3D ( 'NONE', #86665, #17790, #97502 ) ;
#41879=SURFACE_STYLE_USAGE ( .BOTH. , #17935 ) ;
#41883=CARTESIAN_POINT ( 'NONE',  ( 2.895403141435219485, 2.126176841940962348, 7.934999999999989839 ) ) ;
#41885=AXIS2_PLACEMENT_3D ( 'NONE', #15377, #26303, #106678 ) ;
#41932=CARTESIAN_POINT ( 'NONE',  ( 4.083333333333333925, -5.278424836066144543, 3.047499999999995879 ) ) ;
#41934=CARTESIAN_POINT ( 'NONE',  ( 20.68706980810188867, -2.126176841940956130, 7.934999999999990727 ) ) ;
#41945=MECHANICAL_DESIGN_GEOMETRIC_PRESENTATION_REPRESENTATION('',(#14075),#127512);
#41946=CARTESIAN_POINT ( 'NONE',  ( 127.6984665281606368, -50.67230138428462993, -37.61253110040882319 ) ) ;
#41954=CARTESIAN_POINT ( 'NONE',  ( 25.39999999999999858, 0.000000000000000000, 0.000000000000000000 ) ) ;
#41958=CARTESIAN_POINT ( 'NONE',  ( 60.42123663339494044, -43.84677628532234195, 34.92499999999998295 ) ) ;
#41964=CARTESIAN_POINT ( 'NONE',  ( 127.7579555295392026, -48.22435659090666604, 37.54366622512468865 ) ) ;
#41976=ORIENTED_EDGE ( 'NONE', *, *, #106226, .F. ) ;
#41980=VECTOR ( 'NONE', #38016, 1000.000000000000000 ) ;
#41982=TOROIDAL_SURFACE ( 'NONE', #136966, 31.92999999999999972, 3.000000000000000000 ) ;
#41988=EDGE_LOOP ( 'NONE', ( #3324, #84082, #43484 ) ) ;
#41992=CARTESIAN_POINT ( 'NONE',  ( 16.54623647476855552, -7.934999999999990727, 4.858786175617117713E-16 ) ) ;
#41997=ORIENTED_EDGE ( 'NONE', *, *, #86910, .F. ) ;
#42007=FACE_OUTER_BOUND ( 'NONE', #37903, .T. ) ;
#42015=EDGE_LOOP ( 'NONE', ( #141381, #60730, #21280, #106094 ) ) ;
#42017=CARTESIAN_POINT ( 'NONE',  ( 25.40000000000000924, -4.504858206827953460, -6.583681173200965908 ) ) ;
#42032=CARTESIAN_POINT ( 'NONE',  ( 151.4000000000000057, -17.48000000000005016, 12.69999999999954454 ) ) ;
#42034=FILL_AREA_STYLE_COLOUR ( '', #92439 ) ;
#42066=CARTESIAN_POINT ( 'NONE',  ( 13.92123647476855197, -9.717572351234235426E-16, -7.934999999999990727 ) ) ;
#42070=CARTESIAN_POINT ( 'NONE',  ( 55.18164086290597226, -49.14999999999998437, -41.64499999999999602 ) ) ;
#42081=CARTESIAN_POINT ( 'NONE',  ( 184.1383206845090967, -50.55966373067075637, -35.89041033429538885 ) ) ;
#42092=COLOUR_RGB ( '', 0.66274510, 0.83137255, 0.94901961) ;
#42095=MECHANICAL_DESIGN_GEOMETRIC_PRESENTATION_REPRESENTATION('',(#55969),#81430);
#42097=CARTESIAN_POINT ( 'NONE',  ( 0.07085943933670184325, -51.15040958483974975, -36.98623100868706359 ) ) ;
#42102=DIRECTION ( 'NONE',  ( 0.000000000000000000, 0.000000000000000000, -1.000000000000000000 ) ) ;
#42118=ORIENTED_EDGE ( 'NONE', *, *, #8812, .F. ) ;
#42140=FILL_AREA_STYLE_COLOUR ( '', #75213 ) ;
#42143=CARTESIAN_POINT ( 'NONE',  ( 23.62500000000000355, 6.094999999999989981, -1.119633336120465690E-15 ) ) ;
#42241=CARTESIAN_POINT ( 'NONE',  ( 15.08790314143521982, 6.871911579029515771, 3.967499999999989146 ) ) ;
#42265=CARTESIAN_POINT ( 'NONE',  ( 4.666666666666666963, -5.278424836066145431, -3.047499999999993658 ) ) ;
#42273=CARTESIAN_POINT ( 'NONE',  ( 10.47873647476855119, -5.808823158059033709, 5.808823158059035485 ) ) ;
#42278=( NAMED_UNIT ( * ) PLANE_ANGLE_UNIT ( ) SI_UNIT ( $, .RADIAN. ) );
#42311=( NAMED_UNIT ( * ) PLANE_ANGLE_UNIT ( ) SI_UNIT ( $, .RADIAN. ) );
#42314=AXIS2_PLACEMENT_3D ( 'NONE', #124272, #23526, #79395 ) ;
#42345=FILL_AREA_STYLE ('',( #8911 ) ) ;
#42374=DIRECTION ( 'NONE',  ( 1.000000000000000000, 0.000000000000000000, -0.000000000000000000 ) ) ;
#42376=DIRECTION ( 'NONE',  ( -1.000000000000000000, 0.000000000000000000, 0.000000000000000000 ) ) ;
#42385=EDGE_CURVE ( 'NONE', #3140, #97576, #51818, .T. ) ;
#42417=CARTESIAN_POINT ( 'NONE',  ( 26.29580628287044064, -5.278424836066144543, 3.047499999999995879 ) ) ;
#42462=CARTESIAN_POINT ( 'NONE',  ( 55.47138350052870948, -49.14501756083438266, 40.36361034346624876 ) ) ;
#42475=ORIENTED_EDGE ( 'NONE', *, *, #44883, .T. ) ;
#42499=CARTESIAN_POINT ( 'NONE',  ( 29.89583333333333925, 1.633150327867687324, -6.094999999999991758 ) ) ;
#42506=SURFACE_STYLE_FILL_AREA ( #141809 ) ;
#42521=SURFACE_STYLE_FILL_AREA ( #141824 ) ;
#42548=CARTESIAN_POINT ( 'NONE',  ( 180.9243601523649261, -48.88932940808383165, 39.16623080367948972 ) ) ;
#42563=CARTESIAN_POINT ( 'NONE',  ( 183.9019840361164029, -51.74944211519454740, 38.65549799471349957 ) ) ;
#42569=CARTESIAN_POINT ( 'NONE',  ( 3.730677800976855973, -49.14999999999999147, -40.92499999999998295 ) ) ;
#42602=VERTEX_POINT ( 'NONE', #7748 ) ;
#42603=PRESENTATION_STYLE_ASSIGNMENT (( #33168 ) ) ;
#42619=CARTESIAN_POINT ( 'NONE',  ( 17.47873647476855652, -5.808823158059033709, 5.808823158059035485 ) ) ;
#42622=CARTESIAN_POINT ( 'NONE',  ( 156.1500000000000057, -57.14999999999999147, -49.92499999999968452 ) ) ;
#42627=FACE_OUTER_BOUND ( 'NONE', #9209, .T. ) ;
#42657=CARTESIAN_POINT ( 'NONE',  ( 181.1500000000000057, -3.180000000000061444, -31.92499999999998295 ) ) ;
#42662=CARTESIAN_POINT ( 'NONE',  ( 9.333333333333333925, 5.278424836066143655, -3.047499999999997655 ) ) ;
#42663=CARTESIAN_POINT ( 'NONE',  ( 18.79123647476855652, -9.717572351234235426E-16, -7.934999999999990727 ) ) ;
#42674=CARTESIAN_POINT ( 'NONE',  ( 127.7579555295392595, -48.22435659090664473, -37.54366622512464602 ) ) ;
#42685=DIRECTION ( 'NONE',  ( 0.1737853339090545957, -0.1737853339090541793, -0.9693282805305111216 ) ) ;
#42697=CARTESIAN_POINT ( 'NONE',  ( 130.7303687233793710, -48.51451318982915950, 38.21513923099971777 ) ) ;
#42700=CARTESIAN_POINT ( 'NONE',  ( 183.8964364361580408, -51.76057561339556656, 38.69631370864702546 ) ) ;
#42708=B_SPLINE_CURVE_WITH_KNOTS ( 'NONE', 3,
 ( #41214, #86166, #19470, #65146, #52098, #130391, #62282, #85419, #20158, #107873, #8542, #109336 ),
 .UNSPECIFIED., .F., .F.,
 ( 4, 2, 2, 2, 2, 4 ),
 ( 0.000000000000000000, 0.001816333612422246432, 0.002724500418633369649, 0.003632667224844492865, 0.005449000837266739297, 0.007265334449688985730 ),
 .UNSPECIFIED. ) ;
#42714=CARTESIAN_POINT ( 'NONE',  ( 16.83790314143521982, -6.871911579029513106, -3.967499999999993587 ) ) ;
#42718=CARTESIAN_POINT ( 'NONE',  ( 165.9183975471111410, 26.96999999999993847, 33.53367344373089054 ) ) ;
#42724=CARTESIAN_POINT ( 'NONE',  ( 27.99999999999996803, -57.14999999999999147, 53.92499999999996874 ) ) ;
#42754=COLOUR_RGB ( '', 0.66274510, 0.83137255, 0.94901961) ;
#42762=CARTESIAN_POINT ( 'NONE',  ( 128.9683591370937563, -52.14999999999999147, 41.64499999999997470 ) ) ;
#42783=CARTESIAN_POINT ( 'NONE',  ( 10.85873647476855197, 5.808823158059031044, -5.808823158059038150 ) ) ;
#42788=DIRECTION ( 'NONE',  ( 0.000000000000000000, 0.000000000000000000, 1.000000000000000000 ) ) ;
#42821=CARTESIAN_POINT ( 'NONE',  ( 0.1600000000000038058, -0.6768933422324286964, -7.934999999999988951 ) ) ;
#42891=( NAMED_UNIT ( * ) PLANE_ANGLE_UNIT ( ) SI_UNIT ( $, .RADIAN. ) );
#42914=VERTEX_POINT ( 'NONE', #104027 ) ;
#42947=ORIENTED_EDGE ( 'NONE', *, *, #118953, .T. ) ;
#42951=CARTESIAN_POINT ( 'NONE',  ( 18.73373647476854842, 5.808823158059036373, 5.808823158059032821 ) ) ;
#42959=DIRECTION ( 'NONE',  ( -1.000000000000000000, -0.000000000000000000, -0.000000000000000000 ) ) ;
#43010=( NAMED_UNIT ( * ) SI_UNIT ( $, .STERADIAN. ) SOLID_ANGLE_UNIT ( ) );
#43043=( LENGTH_UNIT ( ) NAMED_UNIT ( * ) SI_UNIT ( .MILLI., .METRE. ) );
#43054=FILL_AREA_STYLE_COLOUR ( '', #143381 ) ;
#43094=COLOUR_RGB ( '', 0.08235294, 0.09019608, 0.10196078) ;
#43114=DIRECTION ( 'NONE',  ( 0.000000000000000000, 0.000000000000000000, 1.000000000000000000 ) ) ;
#43117=CARTESIAN_POINT ( 'NONE',  ( 24.83747294953710849, 6.094999999999989981, -1.119633336120465690E-15 ) ) ;
#43120=VECTOR ( 'NONE', #85456, 1000.000000000000000 ) ;
#43128=CARTESIAN_POINT ( 'NONE',  ( 25.39999999999999858, -43.14999999999999147, -34.92499999999998295 ) ) ;
#43162=DIRECTION ( 'NONE',  ( 0.000000000000000000, 0.000000000000000000, -1.000000000000000000 ) ) ;
#43179=FILL_AREA_STYLE ('',( #21417 ) ) ;
#43286=CARTESIAN_POINT ( 'NONE',  ( -0.6833603837962275440, -1.633150327867691987, -6.094999999999989093 ) ) ;
#43291=DIRECTION ( 'NONE',  ( 0.000000000000000000, 1.000000000000000000, 5.782411586589357244E-15 ) ) ;
#43311=CARTESIAN_POINT ( 'NONE',  ( 14.27040314143522082, -7.934999999999989839, 2.126176841940957907 ) ) ;
#43320=CARTESIAN_POINT ( 'NONE',  ( 20.12500000000000000, 6.094999999999989981, -1.119633336120465690E-15 ) ) ;
#43331=ORIENTED_EDGE ( 'NONE', *, *, #111888, .F. ) ;
#43347=AXIS2_PLACEMENT_3D ( 'NONE', #122531, #23198, #100796 ) ;
#43355=CARTESIAN_POINT ( 'NONE',  ( 7.291666666666667851, -3.047499999999994547, 5.278424836066145431 ) ) ;
#43356=CARTESIAN_POINT ( 'NONE',  ( 20.97873647476855652, -5.808823158059033709, 5.808823158059035485 ) ) ;
#43367=CARTESIAN_POINT ( 'NONE',  ( 128.1966263608623251, -51.41954113333838450, -38.53170190052303212 ) ) ;
#43368=VERTEX_POINT ( 'NONE', #61160 ) ;
#43390=CARTESIAN_POINT ( 'NONE',  ( 128.8595569075059188, -47.26730531257519630, 36.54674188582486494 ) ) ;
#43400=( GEOMETRIC_REPRESENTATION_CONTEXT ( 3 ) GLOBAL_UNCERTAINTY_ASSIGNED_CONTEXT ( ( #87009 ) ) GLOBAL_UNIT_ASSIGNED_CONTEXT ( ( #60137, #49970, #126777 ) ) REPRESENTATION_CONTEXT ( 'NONE', 'WORKASPACE' ) );
#43407=CARTESIAN_POINT ( 'NONE',  ( 19.02540314143521982, 2.126176841940962348, 7.934999999999988951 ) ) ;
#43436=ORIENTED_EDGE ( 'NONE', *, *, #119112, .T. ) ;
#43473=EDGE_CURVE ( 'NONE', #65849, #8597, #128120, .T. ) ;
#43475=COLOUR_RGB ( '', 0.66274510, 0.83137255, 0.94901961) ;
#43476=CARTESIAN_POINT ( 'NONE',  ( 23.25456980810188767, -6.871911579029512218, 3.967499999999996252 ) ) ;
#43484=ORIENTED_EDGE ( 'NONE', *, *, #83419, .T. ) ;
#43503=CARTESIAN_POINT ( 'NONE',  ( 61.46640106136302961, -1.600000000000086020, -34.92499999999998295 ) ) ;
#43507=UNCERTAINTY_MEASURE_WITH_UNIT (LENGTH_MEASURE( 1.000000000000000082E-05 ), #29495, 'distance_accuracy_value', 'NONE');
#43511=CARTESIAN_POINT ( 'NONE',  ( 0.1599999999999984490, -7.872400080523645371, -1.050197800354446098 ) ) ;
#43558=DIRECTION ( 'NONE',  ( 0.000000000000000000, 0.000000000000000000, -1.000000000000000000 ) ) ;
#43582=ORIENTED_EDGE ( 'NONE', *, *, #91700, .T. ) ;
#43586=DIRECTION ( 'NONE',  ( 0.000000000000000000, -1.000000000000000000, 0.000000000000000000 ) ) ;
#43587=EDGE_LOOP ( 'NONE', ( #51171, #43582, #131710, #90492, #30493, #56979 ) ) ;
#43590=( LENGTH_UNIT ( ) NAMED_UNIT ( * ) SI_UNIT ( .MILLI., .METRE. ) );
#43599=CARTESIAN_POINT ( 'NONE',  ( 25.26393171409163330, 4.523673662833495257, 4.354767379111166292 ) ) ;
#43639=EDGE_CURVE ( 'NONE', #71793, #5240, #54314, .T. ) ;
#43641=CARTESIAN_POINT ( 'NONE',  ( 14.21290314143522160, 3.967499999999992699, -6.871911579029513994 ) ) ;
#43643=ADVANCED_FACE ( 'NONE', ( #15944 ), #126873, .F. ) ;
#43646=EDGE_CURVE ( 'NONE', #66484, #132969, #132757, .T. ) ;
#43708=SURFACE_SIDE_STYLE ('',( #35001 ) ) ;
#43745=CARTESIAN_POINT ( 'NONE',  ( 15.75000000000000000, -7.464222240803106570E-16, -6.094999999999989981 ) ) ;
#43818=CARTESIAN_POINT ( 'NONE',  ( 21.77497294953710494, 4.461849672132300881, 4.461849672132299105 ) ) ;
#43850=DIRECTION ( 'NONE',  ( 0.000000000000000000, 0.000000000000000000, 1.000000000000000000 ) ) ;
#43867=CARTESIAN_POINT ( 'NONE',  ( 55.45435323442900710, -52.10358567239564564, 40.45860062937861557 ) ) ;
#43917=ORIENTED_EDGE ( 'NONE', *, *, #123118, .F. ) ;
#43922=EDGE_CURVE ( 'NONE', #89491, #26834, #97843, .T. ) ;
#43926=SURFACE_STYLE_FILL_AREA ( #109165 ) ;
#43928=DIRECTION ( 'NONE',  ( 0.000000000000000000, 0.000000000000000000, 1.000000000000000000 ) ) ;
#43959=FACE_OUTER_BOUND ( 'NONE', #70755, .T. ) ;
#43970=CARTESIAN_POINT ( 'NONE',  ( 128.5894344200537773, -52.00875322212549179, -39.86617647058817226 ) ) ;
#43975=CARTESIAN_POINT ( 'NONE',  ( 61.46640106136302961, -43.14999999999999147, -34.92499999999998295 ) ) ;
#43979=CARTESIAN_POINT ( 'NONE',  ( 2.524972949537106270, -4.461849672132299993, -4.461849672132299105 ) ) ;
#44005=( LENGTH_UNIT ( ) NAMED_UNIT ( * ) SI_UNIT ( .MILLI., .METRE. ) );
#44025=CARTESIAN_POINT ( 'NONE',  ( 10.91623647476855297, -7.934999999999990727, 4.858786175617117713E-16 ) ) ;
#44057=PLANE ( 'NONE',  #99392 ) ;
#44070=CARTESIAN_POINT ( 'NONE',  ( 14.58333333333333570, -5.278424836066144543, 3.047499999999995879 ) ) ;
#44071=CARTESIAN_POINT ( 'NONE',  ( 18.20790314143522082, -6.871911579029513106, -3.967499999999993587 ) ) ;
#44078=STYLED_ITEM ( 'NONE', ( #143048 ), #97639 ) ;
#44080=EDGE_LOOP ( 'NONE', ( #31334, #90458, #21997, #24663, #94576 ) ) ;
#44093=SURFACE_STYLE_USAGE ( .BOTH. , #133255 ) ;
#44099=( NAMED_UNIT ( * ) PLANE_ANGLE_UNIT ( ) SI_UNIT ( $, .RADIAN. ) );
#44128=CARTESIAN_POINT ( 'NONE',  ( 153.4000000000000057, -1.600000000000094458, 34.92499999999998295 ) ) ;
#44129=CARTESIAN_POINT ( 'NONE',  ( 14.65040314143522160, 7.934999999999988951, -2.126176841940961904 ) ) ;
#44132=CARTESIAN_POINT ( 'NONE',  ( 3.191216777807910354, -48.83231052142030393, -38.98973348322098076 ) ) ;
#44136=EDGE_CURVE ( 'NONE', #11916, #23830, #47094, .T. ) ;
#44147=CARTESIAN_POINT ( 'NONE',  ( 25.39999999999999858, 0.000000000000000000, 0.000000000000000000 ) ) ;
#44155=ORIENTED_EDGE ( 'NONE', *, *, #26901, .F. ) ;
#44166=B_SPLINE_CURVE_WITH_KNOTS ( 'NONE', 3,
 ( #142826, #109482, #140667, #30507, #118183, #40669, #65295, #43511, #118921, #41355, #87732, #29759, #64549, #85569, #129799, #76148, #19611, #63858, #108018, #108729, #9410, #53695, #42821, #87018 ),
 .UNSPECIFIED., .F., .F.,
 ( 4, 2, 2, 1, 2, 2, 2, 2, 2, 1, 2, 2, 4 ),
 ( 1.221256415468642823E-17, 0.002003734080813304470, 0.003005601121219949549, 0.004007468161626595061, 0.005009335202033241008, 0.006011202242439885220, 0.008014936323253174510, 0.01001867040406646293, 0.01102053744447310628, 0.01202240448487974789, 0.01302427152528639297, 0.01402613856569303458, 0.01602987264650632127 ),
 .UNSPECIFIED. ) ;
#44199=( GEOMETRIC_REPRESENTATION_CONTEXT ( 3 ) GLOBAL_UNCERTAINTY_ASSIGNED_CONTEXT ( ( #90978 ) ) GLOBAL_UNIT_ASSIGNED_CONTEXT ( ( #122113, #108349, #120676 ) ) REPRESENTATION_CONTEXT ( 'NONE', 'WORKASPACE' ) );
#44209=CARTESIAN_POINT ( 'NONE',  ( 21.35873647476855552, 5.808823158059031044, -5.808823158059038150 ) ) ;
#44252=CARTESIAN_POINT ( 'NONE',  ( 17.91623647476855652, -7.934999999999990727, 4.858786175617117713E-16 ) ) ;
#44255=( GEOMETRIC_REPRESENTATION_CONTEXT ( 3 ) GLOBAL_UNCERTAINTY_ASSIGNED_CONTEXT ( ( #41746 ) ) GLOBAL_UNIT_ASSIGNED_CONTEXT ( ( #93581, #105160, #39202 ) ) REPRESENTATION_CONTEXT ( 'NONE', 'WORKASPACE' ) );
#44315=DIRECTION ( 'NONE',  ( 0.000000000000000000, 0.000000000000000000, 1.000000000000000000 ) ) ;
#44317=( LENGTH_UNIT ( ) NAMED_UNIT ( * ) SI_UNIT ( .MILLI., .METRE. ) );
#44327=EDGE_LOOP ( 'NONE', ( #131246, #101543, #95465, #47274 ) ) ;
#44335=VECTOR ( 'NONE', #32636, 1000.000000000000000 ) ;
#44336=SURFACE_STYLE_USAGE ( .BOTH. , #45768 ) ;
#44344=ORIENTED_EDGE ( 'NONE', *, *, #40207, .F. ) ;
#44362=ADVANCED_FACE ( 'NONE', ( #23493 ), #134419, .T. ) ;
#44368=FACE_BOUND ( 'NONE', #69242, .T. ) ;
#44383=CARTESIAN_POINT ( 'NONE',  ( 162.5099761671747274, 26.96999999999994557, -34.76218228780558661 ) ) ;
#44388=( GEOMETRIC_REPRESENTATION_CONTEXT ( 3 ) GLOBAL_UNCERTAINTY_ASSIGNED_CONTEXT ( ( #44788 ) ) GLOBAL_UNIT_ASSIGNED_CONTEXT ( ( #88140, #122157, #113428 ) ) REPRESENTATION_CONTEXT ( 'NONE', 'WORKASPACE' ) );
#44391=CARTESIAN_POINT ( 'NONE',  ( 24.71290314143521982, 3.967499999999992699, -6.871911579029513994 ) ) ;
#44444=VECTOR ( 'NONE', #68798, 1000.000000000000000 ) ;
#44446=CIRCLE ( 'NONE', #408, 3.000000000000000000 ) ;
#44454=ORIENTED_EDGE ( 'NONE', *, *, #15465, .T. ) ;
#44455=DIRECTION ( 'NONE',  ( 0.000000000000000000, -1.000000000000000000, 0.000000000000000000 ) ) ;
#44572=CARTESIAN_POINT ( 'NONE',  ( 4.004569808101885897, 6.871911579029510442, -3.967499999999998916 ) ) ;
#44621=SURFACE_STYLE_USAGE ( .BOTH. , #11183 ) ;
#44632=CARTESIAN_POINT ( 'NONE',  ( 0.000000000000000000, 9.913515839097813477E-16, -8.094999999999991758 ) ) ;
#44639=DIRECTION ( 'NONE',  ( -1.000000000000000000, 0.000000000000000000, 0.000000000000000000 ) ) ;
#44647=UNCERTAINTY_MEASURE_WITH_UNIT (LENGTH_MEASURE( 1.000000000000000082E-05 ), #58733, 'distance_accuracy_value', 'NONE');
#44670=PRESENTATION_STYLE_ASSIGNMENT (( #377 ) ) ;
#44676=PRESENTATION_STYLE_ASSIGNMENT (( #19999 ) ) ;
#44750=CARTESIAN_POINT ( 'NONE',  ( -1.995860383796227877, -3.047499999999994547, 5.278424836066145431 ) ) ;
#44770=AXIS2_PLACEMENT_3D ( 'NONE', #92479, #46923, #68637 ) ;
#44778=CARTESIAN_POINT ( 'NONE',  ( 13.24956980810188689, 3.967499999999998916, 6.871911579029510442 ) ) ;
#44783=ORIENTED_EDGE ( 'NONE', *, *, #118575, .F. ) ;
#44788=UNCERTAINTY_MEASURE_WITH_UNIT (LENGTH_MEASURE( 1.000000000000000082E-05 ), #88140, 'distance_accuracy_value', 'NONE');
#44807=MECHANICAL_DESIGN_GEOMETRIC_PRESENTATION_REPRESENTATION('',(#14645),#33207);
#44809=DIRECTION ( 'NONE',  ( -1.000000000000000000, -0.000000000000000000, -0.000000000000000000 ) ) ;
#44818=UNCERTAINTY_MEASURE_WITH_UNIT (LENGTH_MEASURE( 1.000000000000000082E-05 ), #99293, 'distance_accuracy_value', 'NONE');
#44827=CARTESIAN_POINT ( 'NONE',  ( 18.37500000000000355, -6.094999999999989981, 3.732111120401553285E-16 ) ) ;
#44828=CARTESIAN_POINT ( 'NONE',  ( 22.14540314143522082, -2.126176841940958351, -7.934999999999988951 ) ) ;
#44833=ORIENTED_EDGE ( 'NONE', *, *, #123583, .F. ) ;
#44841=CARTESIAN_POINT ( 'NONE',  ( 125.9798776214792468, -48.09441802426616164, -35.89947574910151928 ) ) ;
#44864=ADVANCED_FACE ( 'NONE', ( #36357, #27595 ), #116026, .F. ) ;
#44883=EDGE_CURVE ( 'NONE', #53957, #61426, #4357, .T. ) ;
#44888=CARTESIAN_POINT ( 'NONE',  ( 23.98373647476855197, -5.808823158059035485, -5.808823158059033709 ) ) ;
#44891=CARTESIAN_POINT ( 'NONE',  ( 166.6278473451638149, 26.96999999999994557, 32.76352092273798178 ) ) ;
#44909=CARTESIAN_POINT ( 'NONE',  ( 25.39999999999999858, -14.29000000000013593, 12.69999999999954632 ) ) ;
#44929=CARTESIAN_POINT ( 'NONE',  ( 0.000000000000000000, -4.600000000000012079, -20.40202195861968093 ) ) ;
#44930=VECTOR ( 'NONE', #42959, 1000.000000000000000 ) ;
#44931=LINE ( 'NONE', #142761, #67902 ) ;
#44946=CARTESIAN_POINT ( 'NONE',  ( 14.92080628287044064, 3.047499999999997655, 5.278424836066143655 ) ) ;
#44957=CARTESIAN_POINT ( 'NONE',  ( 22.81706980810188767, -2.126176841940956130, 7.934999999999991616 ) ) ;
#44965=CARTESIAN_POINT ( 'NONE',  ( 28.00000000000002487, -49.14999999999999147, -59.92499999999979821 ) ) ;
#44971=FILL_AREA_STYLE_COLOUR ( '', #142922 ) ;
#44989=UNCERTAINTY_MEASURE_WITH_UNIT (LENGTH_MEASURE( 1.000000000000000082E-05 ), #81499, 'distance_accuracy_value', 'NONE');
#44998=CARTESIAN_POINT ( 'NONE',  ( 23.74956980810188867, 3.967499999999998916, 6.871911579029510442 ) ) ;
#45022=CARTESIAN_POINT ( 'NONE',  ( 24.06249999999999645, 4.461849672132300881, 4.461849672132299105 ) ) ;
#45028=VERTEX_POINT ( 'NONE', #57176 ) ;
#45111=CARTESIAN_POINT ( 'NONE',  ( 27.99999999999999645, -49.14999999999999147, -45.92499999999969873 ) ) ;
#45114=CARTESIAN_POINT ( 'NONE',  ( 31.71290314143522693, 3.967499999999992699, -6.871911579029513994 ) ) ;
#45132=( GEOMETRIC_REPRESENTATION_CONTEXT ( 3 ) GLOBAL_UNCERTAINTY_ASSIGNED_CONTEXT ( ( #37291 ) ) GLOBAL_UNIT_ASSIGNED_CONTEXT ( ( #132329, #58898, #20661 ) ) REPRESENTATION_CONTEXT ( 'NONE', 'WORKASPACE' ) );
#45146=ORIENTED_EDGE ( 'NONE', *, *, #119112, .F. ) ;
#45166=CARTESIAN_POINT ( 'NONE',  ( 1.392138667788030526, -2.420047799299299474, -6.258046653434560014 ) ) ;
#45200=PRESENTATION_STYLE_ASSIGNMENT (( #100261 ) ) ;
#45218=CARTESIAN_POINT ( 'NONE',  ( 24.39999999999999858, -1.600000000000055600, -28.92500000000001492 ) ) ;
#45224=MECHANICAL_DESIGN_GEOMETRIC_PRESENTATION_REPRESENTATION('',(#96072),#135442);
#45239=LINE ( 'NONE', #88728, #34120 ) ;
#45272=( NAMED_UNIT ( * ) SI_UNIT ( $, .STERADIAN. ) SOLID_ANGLE_UNIT ( ) );
#45280=CARTESIAN_POINT ( 'NONE',  ( 31.39997294953710849, 4.461849672132297329, -4.461849672132302658 ) ) ;
#45306=LINE ( 'NONE', #11905, #115457 ) ;
#45311=( NAMED_UNIT ( * ) PLANE_ANGLE_UNIT ( ) SI_UNIT ( $, .RADIAN. ) );
#45323=PRESENTATION_STYLE_ASSIGNMENT (( #89497 ) ) ;
#45332=SURFACE_STYLE_FILL_AREA ( #111240 ) ;
#45335=DIRECTION ( 'NONE',  ( -0.7071067811865487940, 8.659560562354918067E-17, -0.7071067811865463515 ) ) ;
#45388=DIRECTION ( 'NONE',  ( 0.000000000000000000, 0.000000000000000000, -1.000000000000000000 ) ) ;
#45419=ORIENTED_EDGE ( 'NONE', *, *, #116709, .F. ) ;
#45422=CARTESIAN_POINT ( 'NONE',  ( 3.545806282870439308, 5.278424836066143655, -3.047499999999997655 ) ) ;
#45430=CYLINDRICAL_SURFACE ( 'NONE', #124542, 5.999999999999998224 ) ;
#45445=CARTESIAN_POINT ( 'NONE',  ( 3.691639616203772789, 6.094999999999988205, -1.633150327867694651 ) ) ;
#45455=( NAMED_UNIT ( * ) SI_UNIT ( $, .STERADIAN. ) SOLID_ANGLE_UNIT ( ) );
#45473=EDGE_CURVE ( 'NONE', #17685, #37393, #29026, .T. ) ;
#45475=CARTESIAN_POINT ( 'NONE',  ( 9.457903141435219041, 6.871911579029515771, 3.967499999999989146 ) ) ;
#45484=CARTESIAN_POINT ( 'NONE',  ( 20.41666666666667140, 5.278424836066147208, 3.047499999999990550 ) ) ;
#45501=EDGE_LOOP ( 'NONE', ( #140326, #31748, #109171, #36768 ) ) ;
#45503=CARTESIAN_POINT ( 'NONE',  ( 17.25413961620377279, 3.047499999999993214, -5.278424836066146320 ) ) ;
#45517=CARTESIAN_POINT ( 'NONE',  ( 25.39999999999999858, -16.48000000000005016, 12.69999999999954454 ) ) ;
#45523=CARTESIAN_POINT ( 'NONE',  ( 17.20833333333333570, 3.047499999999997655, 5.278424836066143655 ) ) ;
#45524=CARTESIAN_POINT ( 'NONE',  ( 22.29123647476855652, -9.717572351234235426E-16, -7.934999999999990727 ) ) ;
#45540=( NAMED_UNIT ( * ) SI_UNIT ( $, .STERADIAN. ) SOLID_ANGLE_UNIT ( ) );
#45581=CARTESIAN_POINT ( 'NONE',  ( 21.21290314143522338, 3.967499999999992699, -6.871911579029513994 ) ) ;
#45583=CARTESIAN_POINT ( 'NONE',  ( 162.5049720716601200, 26.96999999999993847, 34.75200654934010913 ) ) ;
#45605=ORIENTED_EDGE ( 'NONE', *, *, #78762, .F. ) ;
#45646=CARTESIAN_POINT ( 'NONE',  ( 15.52540314143522160, 2.126176841940962348, 7.934999999999989839 ) ) ;
#45679=LINE ( 'NONE', #43503, #80826 ) ;
#45692=CARTESIAN_POINT ( 'NONE',  ( 24.91623647476855652, -7.934999999999990727, 4.858786175617117713E-16 ) ) ;
#45693=CARTESIAN_POINT ( 'NONE',  ( 2.749569808101886004, 3.967499999999998916, 6.871911579029510442 ) ) ;
#45728=CIRCLE ( 'NONE', #73435, 1.000000000000000888 ) ;
#45745=EDGE_CURVE ( 'NONE', #11327, #94854, #101584, .T. ) ;
#45750=CARTESIAN_POINT ( 'NONE',  ( 3.712903141435219379, 3.967499999999992699, -6.871911579029513994 ) ) ;
#45758=ORIENTED_EDGE ( 'NONE', *, *, #32380, .F. ) ;
#45761=CYLINDRICAL_SURFACE ( 'NONE', #61410, 1.000000000000000888 ) ;
#45768=SURFACE_SIDE_STYLE ('',( #132048 ) ) ;
#45807=CARTESIAN_POINT ( 'NONE',  ( 26.60873647476855552, -5.808823158059033709, 5.808823158059035485 ) ) ;
#45809=FILL_AREA_STYLE ('',( #12428 ) ) ;
#45835=CIRCLE ( 'NONE', #101370, 6.094999999999989093 ) ;
#45845=ORIENTED_EDGE ( 'NONE', *, *, #16833, .F. ) ;
#45858=VERTEX_POINT ( 'NONE', #136360 ) ;
#45880=CARTESIAN_POINT ( 'NONE',  ( 1.274578247585341995, 1.447108250109749417, 6.668332787597689659 ) ) ;
#45949=ORIENTED_EDGE ( 'NONE', *, *, #54951, .F. ) ;
#45968=EDGE_CURVE ( 'NONE', #100698, #107938, #29038, .T. ) ;
#45981=CARTESIAN_POINT ( 'NONE',  ( 0.5045698081018860082, 6.871911579029510442, -3.967499999999998916 ) ) ;
#46009=DIRECTION ( 'NONE',  ( -0.000000000000000000, -1.000000000000000000, -0.000000000000000000 ) ) ;
#46051=UNCERTAINTY_MEASURE_WITH_UNIT (LENGTH_MEASURE( 1.000000000000000082E-05 ), #123452, 'distance_accuracy_value', 'NONE');
#46052=COLOUR_RGB ( '', 0.08235294, 0.09019608, 0.10196078) ;
#46056=EDGE_CURVE ( 'NONE', #73841, #99786, #81260, .T. ) ;
#46059=EDGE_CURVE ( 'NONE', #89491, #50573, #74710, .T. ) ;
#46065=CARTESIAN_POINT ( 'NONE',  ( 152.4000000000000057, 7.919999999999947526, 19.12499999999998224 ) ) ;
#46071=CARTESIAN_POINT ( 'NONE',  ( 25.39999999999999858, 1.126161369193133366, -16.41140641659140798 ) ) ;
#46105=DIRECTION ( 'NONE',  ( -0.000000000000000000, 1.000000000000000000, -0.000000000000000000 ) ) ;
#46157=CARTESIAN_POINT ( 'NONE',  ( 5.004139616203772789, -3.047499999999994547, 5.278424836066145431 ) ) ;
#46170=( NAMED_UNIT ( * ) PLANE_ANGLE_UNIT ( ) SI_UNIT ( $, .RADIAN. ) );
#46184=CARTESIAN_POINT ( 'NONE',  ( 28.00000000000002487, -52.14999999999999147, -59.92499999999979821 ) ) ;
#46193=CARTESIAN_POINT ( 'NONE',  ( 23.89540314143522437, 2.126176841940962348, 7.934999999999989839 ) ) ;
#46198=ORIENTED_EDGE ( 'NONE', *, *, #17130, .T. ) ;
#46203=UNCERTAINTY_MEASURE_WITH_UNIT (LENGTH_MEASURE( 1.000000000000000082E-05 ), #135310, 'distance_accuracy_value', 'NONE');
#46207=SURFACE_STYLE_USAGE ( .BOTH. , #1893 ) ;
#46216=CARTESIAN_POINT ( 'NONE',  ( 17.98330628287043709, 6.094999999999991758, 1.633150327867686880 ) ) ;
#46221=DIRECTION ( 'NONE',  ( 0.000000000000000000, -1.000000000000000000, 0.000000000000000000 ) ) ;
#46235=CARTESIAN_POINT ( 'NONE',  ( 10.64583333333333215, -1.633150327867689988, 6.094999999999989981 ) ) ;
#46245=FILL_AREA_STYLE_COLOUR ( '', #41363 ) ;
#46248=CARTESIAN_POINT ( 'NONE',  ( 123.5545056966553688, -44.02090675800832287, -34.92500000000512728 ) ) ;
#46258=ORIENTED_EDGE ( 'NONE', *, *, #57731, .T. ) ;
#46299=CARTESIAN_POINT ( 'NONE',  ( 25.39999999999999147, -6.329169252561944070, -1.258656420499090878 ) ) ;
#46326=DIRECTION ( 'NONE',  ( 0.000000000000000000, 0.000000000000000000, 1.000000000000000000 ) ) ;
#46334=ORIENTED_EDGE ( 'NONE', *, *, #142492, .T. ) ;
#46347=EDGE_CURVE ( 'NONE', #43368, #112625, #77222, .T. ) ;
#46350=FILL_AREA_STYLE_COLOUR ( '', #29536 ) ;
#46374=CARTESIAN_POINT ( 'NONE',  ( 19.31706980810189123, -2.126176841940956130, 7.934999999999991616 ) ) ;
#46382=EDGE_LOOP ( 'NONE', ( #59414, #107361, #93535, #108544 ) ) ;
#46393=MECHANICAL_DESIGN_GEOMETRIC_PRESENTATION_REPRESENTATION('',(#53263),#65213);
#46404=LINE ( 'NONE', #134093, #66945 ) ;
#46406=PRESENTATION_STYLE_ASSIGNMENT (( #57268 ) ) ;
#46407=UNCERTAINTY_MEASURE_WITH_UNIT (LENGTH_MEASURE( 1.000000000000000082E-05 ), #4278, 'distance_accuracy_value', 'NONE');
#46409=CARTESIAN_POINT ( 'NONE',  ( 156.1499999999997783, -49.14999999999999147, -62.92499999999978400 ) ) ;
#46417=DIRECTION ( 'NONE',  ( 0.000000000000000000, -1.000000000000000000, -5.559056632600920815E-15 ) ) ;
#46418=CARTESIAN_POINT ( 'NONE',  ( 20.83290314143522082, -3.967499999999994476, 6.871911579029513106 ) ) ;
#46479=CIRCLE ( 'NONE', #90405, 1.000000000000000888 ) ;
#46497=DIRECTION ( 'NONE',  ( 0.000000000000000000, 0.000000000000000000, -1.000000000000000000 ) ) ;
#46517=VERTEX_POINT ( 'NONE', #133029 ) ;
#46533=VERTEX_POINT ( 'NONE', #24933 ) ;
#46550=CARTESIAN_POINT ( 'NONE',  ( 25.44206980810188412, 7.934999999999993392, 2.126176841940951689 ) ) ;
#46577=AXIS2_PLACEMENT_3D ( 'NONE', #21024, #143529, #74000 ) ;
#46592=ORIENTED_EDGE ( 'NONE', *, *, #1009, .T. ) ;
#46602=CIRCLE ( 'NONE', #92899, 3.000000000000002665 ) ;
#46612=CARTESIAN_POINT ( 'NONE',  ( 0.9370758337544541350, -5.958929145428653484, -3.977263664294321099 ) ) ;
#46627=CARTESIAN_POINT ( 'NONE',  ( 0.3243279295976794208, 5.567135860803324121, -5.437310639911629551 ) ) ;
#46681=EDGE_LOOP ( 'NONE', ( #111670, #4990, #121154, #105504 ) ) ;
#46689=ADVANCED_FACE ( 'NONE', ( #93777 ), #4257, .F. ) ;
#46731=CARTESIAN_POINT ( 'NONE',  ( 2.108736474768552860, -5.808823158059033709, 5.808823158059035485 ) ) ;
#46739=ORIENTED_EDGE ( 'NONE', *, *, #111556, .F. ) ;
#46755=CARTESIAN_POINT ( 'NONE',  ( 21.62913961620377279, 5.278424836066147208, 3.047499999999990550 ) ) ;
#46762=( LENGTH_UNIT ( ) NAMED_UNIT ( * ) SI_UNIT ( .MILLI., .METRE. ) );
#46764=SURFACE_STYLE_USAGE ( .BOTH. , #1722 ) ;
#46770=DIRECTION ( 'NONE',  ( -1.000000000000000000, -0.000000000000000000, 0.000000000000000000 ) ) ;
#46771=DIRECTION ( 'NONE',  ( 0.9843059135695010342, 0.000000000000000000, -0.1764705882352923805 ) ) ;
#46776=COLOUR_RGB ( '', 0.09019608, 0.27058824, 0.51372549) ;
#46797=CARTESIAN_POINT ( 'NONE',  ( 28.00000000000002487, -57.14999999999999147, -62.92499999999978400 ) ) ;
#46809=VERTEX_POINT ( 'NONE', #51716 ) ;
#46821=CARTESIAN_POINT ( 'NONE',  ( 2.999999999999999112, 1.399999999999986366, 20.40202195861970580 ) ) ;
#46879=CIRCLE ( 'NONE', #132547, 3.000000000000002665 ) ;
#46904=CARTESIAN_POINT ( 'NONE',  ( 4.129139616203772789, 5.278424836066147208, 3.047499999999990550 ) ) ;
#46923=DIRECTION ( 'NONE',  ( 0.000000000000000000, -1.000000000000000000, 0.000000000000000000 ) ) ;
#46928=CARTESIAN_POINT ( 'NONE',  ( 25.35373647476855297, -5.808823158059035485, -5.808823158059033709 ) ) ;
#46934=EDGE_CURVE ( 'NONE', #62052, #137014, #69018, .T. ) ;
#46938=AXIS2_PLACEMENT_3D ( 'NONE', #22976, #78848, #12832 ) ;
#46945=CARTESIAN_POINT ( 'NONE',  ( 128.6958184333952602, -52.10373894832327579, 40.45955814675564000 ) ) ;
#46955=( LENGTH_UNIT ( ) NAMED_UNIT ( * ) SI_UNIT ( .MILLI., .METRE. ) );
#46974=CARTESIAN_POINT ( 'NONE',  ( 16.33333333333333570, 5.278424836066143655, -3.047499999999997655 ) ) ;
#46975=CARTESIAN_POINT ( 'NONE',  ( 24.47873647476855652, -5.808823158059033709, 5.808823158059035485 ) ) ;
#46978=CARTESIAN_POINT ( 'NONE',  ( 25.39999999999999858, -1.599999999999997202, -17.44999999999996732 ) ) ;
#46992=CARTESIAN_POINT ( 'NONE',  ( 122.6835989386368055, -43.15000000000001990, -34.92499999999998295 ) ) ;
#47039=CARTESIAN_POINT ( 'NONE',  ( 25.29623647476855908, 7.934999999999990727, -1.457635852685135314E-15 ) ) ;
#47049=CARTESIAN_POINT ( 'NONE',  ( 9.041666666666666075, 3.047499999999993214, -5.278424836066146320 ) ) ;
#47064=DIRECTION ( 'NONE',  ( -1.000000000000000000, -0.000000000000000000, 0.000000000000000000 ) ) ;
#47066=CARTESIAN_POINT ( 'NONE',  ( 166.8575281714868481, 26.96999999999994202, -34.92499999999998295 ) ) ;
#47094=LINE ( 'NONE', #81839, #74948 ) ;
#47105=CARTESIAN_POINT ( 'NONE',  ( 26.75456980810189123, -6.871911579029512218, 3.967499999999996252 ) ) ;
#47107=DIRECTION ( 'NONE',  ( 0.000000000000000000, 0.000000000000000000, -1.000000000000000000 ) ) ;
#47119=PRESENTATION_STYLE_ASSIGNMENT (( #2076 ) ) ;
#47126=( BOUNDED_CURVE ( )  B_SPLINE_CURVE ( 2, ( #15907, #49335, #82651, #40582, #29666, #5764, #94219, #105786, #28980, #60194, #71786, #126839, #73908 ),
 .UNSPECIFIED., .F., .T. ) 
 B_SPLINE_CURVE_WITH_KNOTS ( ( 3, 2, 2, 2, 2, 2, 3 ),
 ( 0.1500000000000000222, 0.1583333333333333537, 0.1666666666666666852, 0.1750000000000000444, 0.1833333333333333759, 0.1916666666666667351, 0.2000000000000000666 ),
 .UNSPECIFIED. ) 
 CURVE ( )  GEOMETRIC_REPRESENTATION_ITEM ( )  RATIONAL_B_SPLINE_CURVE ( ( 0.9999999999999998890, 0.9659258262890684232, 1.000000000000000000, 0.9659258262890683122, 1.000000000000000000, 0.9659258262890683122, 1.000000000000000000, 0.9659258262890683122, 1.000000000000000000, 0.9659258262890683122, 1.000000000000000000, 0.9659258262890680902, 1.000000000000000222 ) ) 
 REPRESENTATION_ITEM ( '' )  );
#47129=CARTESIAN_POINT ( 'NONE',  ( 60.42123663339243933, -43.84677628530859295, -34.92499999999998295 ) ) ;
#47137=SURFACE_STYLE_USAGE ( .BOTH. , #1392 ) ;
#47140=ADVANCED_FACE ( 'NONE', ( #71158 ), #82737, .T. ) ;
#47152=CARTESIAN_POINT ( 'NONE',  ( 23.60373647476854941, 5.808823158059036373, 5.808823158059032821 ) ) ;
#47154=DIRECTION ( 'NONE',  ( -1.000000000000000000, 0.000000000000000000, 0.000000000000000000 ) ) ;
#47158=ORIENTED_EDGE ( 'NONE', *, *, #122692, .F. ) ;
#47166=CIRCLE ( 'NONE', #130420, 3.999999999999989786 ) ;
#47206=CARTESIAN_POINT ( 'NONE',  ( 0.1867277030207833977, 3.637003262229598022, -7.062723959547544617 ) ) ;
#47237=CIRCLE ( 'NONE', #3181, 3.999999999999989786 ) ;
#47238=VERTEX_POINT ( 'NONE', #63847 ) ;
#47239=CIRCLE ( 'NONE', #56544, 2.552699999999928693 ) ;
#47261=DIRECTION ( 'NONE',  ( -1.000000000000000000, 0.000000000000000000, 0.000000000000000000 ) ) ;
#47271=CARTESIAN_POINT ( 'NONE',  ( 30.54623647476855552, -7.934999999999990727, 4.858786175617117713E-16 ) ) ;
#47273=CARTESIAN_POINT ( 'NONE',  ( 2.837903141435219379, -6.871911579029513106, -3.967499999999993587 ) ) ;
#47274=ORIENTED_EDGE ( 'NONE', *, *, #142492, .F. ) ;
#47278=SURFACE_STYLE_FILL_AREA ( #102337 ) ;
#47309=EDGE_CURVE ( 'NONE', #26834, #20276, #46404, .T. ) ;
#47317=EDGE_CURVE ( 'NONE', #86570, #87517, #45679, .T. ) ;
#47329=CARTESIAN_POINT ( 'NONE',  ( 1.130059519929533574, -4.629186425066019517, -5.239578231266678543 ) ) ;
#47333=CARTESIAN_POINT ( 'NONE',  ( 25.39999999999999858, 7.796566843815467607, 1.475727091950665537 ) ) ;
#47340=EDGE_LOOP ( 'NONE', ( #129436, #117735, #120086, #58943 ) ) ;
#47392=SURFACE_STYLE_USAGE ( .BOTH. , #124184 ) ;
#47400=DIRECTION ( 'NONE',  ( 1.000000000000000000, 0.000000000000000000, 0.000000000000000000 ) ) ;
#47412=CIRCLE ( 'NONE', #82161, 3.000000000000002665 ) ;
#47435=CARTESIAN_POINT ( 'NONE',  ( 149.2199999999997999, -3.180000000000061444, 34.92499999999998295 ) ) ;
#47437=SURFACE_SIDE_STYLE ('',( #122799 ) ) ;
#47439=CARTESIAN_POINT ( 'NONE',  ( 31.83747294953710849, 6.094999999999989981, -1.119633336120465690E-15 ) ) ;
#47462=CARTESIAN_POINT ( 'NONE',  ( 20.46247294953710849, -7.464222240803106570E-16, -6.094999999999989981 ) ) ;
#47469=CARTESIAN_POINT ( 'NONE',  ( 5.228736474768552078, 5.808823158059031044, -5.808823158059038150 ) ) ;
#47480=UNCERTAINTY_MEASURE_WITH_UNIT (LENGTH_MEASURE( 1.000000000000000082E-05 ), #9837, 'distance_accuracy_value', 'NONE');
#47487=FACE_OUTER_BOUND ( 'NONE', #48949, .T. ) ;
#47503=UNCERTAINTY_MEASURE_WITH_UNIT (LENGTH_MEASURE( 1.000000000000000082E-05 ), #116815, 'distance_accuracy_value', 'NONE');
#47540=AXIS2_PLACEMENT_3D ( 'NONE', #46065, #12676, #54790 ) ;
#47544=EDGE_LOOP ( 'NONE', ( #55857, #35764, #128636, #86016 ) ) ;
#47583=CARTESIAN_POINT ( 'NONE',  ( 0.000000000000000000, 0.000000000000000000, 0.000000000000000000 ) ) ;
#47597=CARTESIAN_POINT ( 'NONE',  ( 7.337472949537107603, 6.094999999999989981, -1.119633336120465690E-15 ) ) ;
#47603=DIRECTION ( 'NONE',  ( 0.000000000000000000, -1.000000000000000000, 0.000000000000000000 ) ) ;
#47623=CIRCLE ( 'NONE', #52137, 2.999999999999996003 ) ;
#47624=CARTESIAN_POINT ( 'NONE',  ( 26.81206980810188512, 7.934999999999993392, 2.126176841940951689 ) ) ;
#47637=UNCERTAINTY_MEASURE_WITH_UNIT (LENGTH_MEASURE( 1.000000000000000082E-05 ), #86232, 'distance_accuracy_value', 'NONE');
#47657=ADVANCED_FACE ( 'NONE', ( #9980 ), #44057, .F. ) ;
#47663=( LENGTH_UNIT ( ) NAMED_UNIT ( * ) SI_UNIT ( .MILLI., .METRE. ) );
#47675=CARTESIAN_POINT ( 'NONE',  ( 20.70833333333333570, 3.047499999999997655, 5.278424836066143655 ) ) ;
#47676=CARTESIAN_POINT ( 'NONE',  ( 24.91623647476855652, -7.934999999999990727, 4.858786175617117713E-16 ) ) ;
#47686=EDGE_CURVE ( 'NONE', #21546, #129906, #78116, .T. ) ;
#47688=CARTESIAN_POINT ( 'NONE',  ( 124.7734390271410518, -44.54322672567605679, -35.04755940937983638 ) ) ;
#47743=ORIENTED_EDGE ( 'NONE', *, *, #102451, .F. ) ;
#47793=CARTESIAN_POINT ( 'NONE',  ( 27.04623647476855197, -7.934999999999990727, 4.858786175617117713E-16 ) ) ;
#47794=CARTESIAN_POINT ( 'NONE',  ( 184.1500000000000057, -14.29000000000013593, 12.69999999999954632 ) ) ;
#47817=CARTESIAN_POINT ( 'NONE',  ( 60.07317433568100995, -45.23984008851914496, -35.04755940938199643 ) ) ;
#47827=UNCERTAINTY_MEASURE_WITH_UNIT (LENGTH_MEASURE( 1.000000000000000082E-05 ), #12277, 'distance_accuracy_value', 'NONE');
#47842=CARTESIAN_POINT ( 'NONE',  ( 30.60373647476856007, 5.808823158059036373, 5.808823158059032821 ) ) ;
#47854=SURFACE_SIDE_STYLE ('',( #137695 ) ) ;
#47855=CARTESIAN_POINT ( 'NONE',  ( 22.50413961620377634, -3.047499999999994547, 5.278424836066145431 ) ) ;
#47857=VERTEX_POINT ( 'NONE', #93259 ) ;
#47868=CARTESIAN_POINT ( 'NONE',  ( 55.47138350052870948, -49.14501756083438266, 40.36361034346623455 ) ) ;
#47892=FILL_AREA_STYLE ('',( #69643 ) ) ;
#47895=CYLINDRICAL_SURFACE ( 'NONE', #17727, 2.999999999999999112 ) ;
#47930=CARTESIAN_POINT ( 'NONE',  ( 25.39999999999999858, -16.48000000000005016, -34.92499999999998295 ) ) ;
#47957=CARTESIAN_POINT ( 'NONE',  ( 25.39999999999999858, -30.18000000000009564, -15.92500000000064375 ) ) ;
#47959=CARTESIAN_POINT ( 'NONE',  ( 4.733736474768551972, 5.808823158059036373, 5.808823158059032821 ) ) ;
#47973=FILL_AREA_STYLE_COLOUR ( '', #91172 ) ;
#48008=FACE_OUTER_BOUND ( 'NONE', #50938, .T. ) ;
#48020=CARTESIAN_POINT ( 'NONE',  ( 0.9173080810154149445, 6.103147713859270240, 3.800379278936838912 ) ) ;
#48072=FACE_BOUND ( 'NONE', #61985, .T. ) ;
#48102=VERTEX_POINT ( 'NONE', #100925 ) ;
#48103=CIRCLE ( 'NONE', #52628, 3.999999999999989786 ) ;
#48111=( NAMED_UNIT ( * ) SI_UNIT ( $, .STERADIAN. ) SOLID_ANGLE_UNIT ( ) );
#48112=CARTESIAN_POINT ( 'NONE',  ( 6.921236474768553748, -9.717572351234235426E-16, -7.934999999999990727 ) ) ;
#48143=CARTESIAN_POINT ( 'NONE',  ( 5.812069808101887780, 7.934999999999993392, 2.126176841940951689 ) ) ;
#48150=CARTESIAN_POINT ( 'NONE',  ( 52.60764783923757903, -49.05583548141700589, 39.86617647058822911 ) ) ;
#48181=ORIENTED_EDGE ( 'NONE', *, *, #28993, .T. ) ;
#48227=( NAMED_UNIT ( * ) SI_UNIT ( $, .STERADIAN. ) SOLID_ANGLE_UNIT ( ) );
#48242=DIRECTION ( 'NONE',  ( -0.000000000000000000, 1.000000000000000000, -0.000000000000000000 ) ) ;
#48244=EDGE_CURVE ( 'NONE', #98679, #56501, #104493, .T. ) ;
#48245=CARTESIAN_POINT ( 'NONE',  ( 25.40000000000000568, 7.827890782510358747, -1.361049978288880302 ) ) ;
#48261=CARTESIAN_POINT ( 'NONE',  ( 2.962472949537105826, -7.464222240803106570E-16, -6.094999999999989981 ) ) ;
#48283=TOROIDAL_SURFACE ( 'NONE', #76131, 9.000000000000001776, 3.000000000000000000 ) ;
#48294=CARTESIAN_POINT ( 'NONE',  ( 20.24956980810188867, 3.967499999999998916, 6.871911579029510442 ) ) ;
#48309=( BOUNDED_SURFACE ( )  B_SPLINE_SURFACE ( 3, 2, ( 
 ( #107868, #108567, #131802 ),
 ( #131086, #132554, #10010 ),
 ( #98449, #33244, #8535 ),
 ( #43367, #96977, #120912 ),
 ( #77451, #121614, #141230 ),
 ( #41946, #141984, #31774 ),
 ( #31076, #119461, #64396 ),
 ( #97740, #42674, #75991 ),
 ( #120160, #25891, #57833 ),
 ( #1943, #57127, #112202 ),
 ( #44841, #24455, #68021 ),
 ( #12848, #101306, #78145 ),
 ( #102749, #33927, #59272 ),
 ( #2691, #69413, #47688 ),
 ( #123076, #46248, #124488 ),
 ( #90431, #46992, #123800 ) ),
 .UNSPECIFIED., .F., .F., .F. ) 
 B_SPLINE_SURFACE_WITH_KNOTS ( ( 4, 2, 2, 2, 2, 2, 2, 4 ),
 ( 3, 3 ),
 ( 6.460584911619963400, 6.634759501914277990, 6.808934092208593469, 6.983108682502908060, 7.157283272797222651, 7.331457863091538130, 7.505632453385852720, 7.853981633974482790 ),
 ( 0.000000000000000000, 1.000000000000000000 ),
 .UNSPECIFIED. ) 
 GEOMETRIC_REPRESENTATION_ITEM ( )  RATIONAL_B_SPLINE_SURFACE ( (
 ( 1.000000000000000000, 0.7180326832784531543, 1.000000000000000000),
 ( 1.000000000000000000, 0.7250426641246962012, 1.000000000000000000),
 ( 1.000000000000000000, 0.7353122387370452095, 1.000000000000000000),
 ( 1.000000000000000000, 0.7604116155349263106, 1.000000000000000000),
 ( 1.000000000000000000, 0.7752313834059556541, 1.000000000000000000),
 ( 1.000000000000000000, 0.8070860741948175932, 1.000000000000000000),
 ( 1.000000000000000000, 0.8241077986064178074, 1.000000000000000000),
 ( 1.000000000000000000, 0.8581174656083172536, 1.000000000000000000),
 ( 1.000000000000000000, 0.8751006588765014582, 1.000000000000000000),
 ( 1.000000000000000000, 0.9071649184815153699, 1.000000000000000000),
 ( 1.000000000000000000, 0.9222453908327410410, 1.000000000000000000),
 ( 1.000000000000000000, 0.9490805577171569363, 1.000000000000000000),
 ( 1.000000000000000000, 0.9608359430471251628, 1.000000000000000000),
 ( 1.000000000000000000, 0.9896287210067380435, 1.000000000000000000),
 ( 1.000000000000000000, 1.000097732991007682, 1.000000000000000000),
 ( 1.000000000000000000, 1.000000000000000000, 1.000000000000000000) ) ) 
 REPRESENTATION_ITEM ( '' )  SURFACE ( )  );
#48345=CARTESIAN_POINT ( 'NONE',  ( 19.54166666666666785, 3.047499999999993214, -5.278424836066146320 ) ) ;
#48348=( NAMED_UNIT ( * ) SI_UNIT ( $, .STERADIAN. ) SOLID_ANGLE_UNIT ( ) );
#48355=DIRECTION ( 'NONE',  ( 0.000000000000000000, 6.938893903907227589E-15, -1.000000000000000000 ) ) ;
#48370=VERTEX_POINT ( 'NONE', #131985 ) ;
#48390=ORIENTED_EDGE ( 'NONE', *, *, #95567, .T. ) ;
#48392=CARTESIAN_POINT ( 'NONE',  ( 180.5498074873981693, -49.14999999999999147, 40.57313449935463012 ) ) ;
#48395=FILL_AREA_STYLE ('',( #4111 ) ) ;
#48397=CARTESIAN_POINT ( 'NONE',  ( 3.730677800976857306, -52.14999999999999147, -40.92499999999998295 ) ) ;
#48405=MECHANICAL_DESIGN_GEOMETRIC_PRESENTATION_REPRESENTATION('',(#141012),#69233);
#48406=AXIS2_PLACEMENT_3D ( 'NONE', #18361, #48355, #139509 ) ;
#48420=DIRECTION ( 'NONE',  ( -1.000000000000000000, -0.000000000000000000, -0.000000000000000000 ) ) ;
#48434=( GEOMETRIC_REPRESENTATION_CONTEXT ( 3 ) GLOBAL_UNCERTAINTY_ASSIGNED_CONTEXT ( ( #78119 ) ) GLOBAL_UNIT_ASSIGNED_CONTEXT ( ( #138510, #115272, #82024 ) ) REPRESENTATION_CONTEXT ( 'NONE', 'WORKASPACE' ) );
#48465=CARTESIAN_POINT ( 'NONE',  ( 25.29623647476855908, 7.934999999999990727, -1.457635852685135314E-15 ) ) ;
#48511=CARTESIAN_POINT ( 'NONE',  ( 32.06206980810188867, -7.934999999999991616, -2.126176841940955242 ) ) ;
#48526=CARTESIAN_POINT ( 'NONE',  ( 22.64997294953709783, -4.461849672132299105, 4.461849672132299993 ) ) ;
#48547=CARTESIAN_POINT ( 'NONE',  ( 55.57593013779205648, -49.04047092356913851, 39.41690992498946855 ) ) ;
#48568=ORIENTED_EDGE ( 'NONE', *, *, #137035, .F. ) ;
#48570=DIRECTION ( 'NONE',  ( 0.000000000000000000, 0.000000000000000000, -1.000000000000000000 ) ) ;
#48571=CARTESIAN_POINT ( 'NONE',  ( 3.421236474768552860, -9.717572351234235426E-16, -7.934999999999990727 ) ) ;
#48575=( NAMED_UNIT ( * ) PLANE_ANGLE_UNIT ( ) SI_UNIT ( $, .RADIAN. ) );
#48583=EDGE_CURVE ( 'NONE', #137404, #49688, #124297, .T. ) ;
#48589=DIRECTION ( 'NONE',  ( 0.000000000000000000, 0.000000000000000000, -1.000000000000000000 ) ) ;
#48648=CARTESIAN_POINT ( 'NONE',  ( -0.8079301918981138808, -7.934999999999991616, -2.126176841940955242 ) ) ;
#48660=DIRECTION ( 'NONE',  ( 0.000000000000000000, -1.000000000000000000, 0.000000000000000000 ) ) ;
#48663=CARTESIAN_POINT ( 'NONE',  ( 183.7102003651264681, -49.08473565290606189, -39.91868829876866442 ) ) ;
#48678=MECHANICAL_DESIGN_GEOMETRIC_PRESENTATION_REPRESENTATION('',(#13869),#13976);
#48681=CARTESIAN_POINT ( 'NONE',  ( 2.999999999999999112, -4.600000000000094680, 34.92499999999996874 ) ) ;
#48687=CARTESIAN_POINT ( 'NONE',  ( 2.479166666666666963, 6.094999999999988205, -1.633150327867694651 ) ) ;
#48689=DIRECTION ( 'NONE',  ( -1.000000000000000000, -0.000000000000000000, -0.000000000000000000 ) ) ;
#48720=SURFACE_STYLE_FILL_AREA ( #69055 ) ;
#48761=MECHANICAL_DESIGN_GEOMETRIC_PRESENTATION_REPRESENTATION('',(#34898),#58098);
#48809=ORIENTED_EDGE ( 'NONE', *, *, #57731, .F. ) ;
#48827=CARTESIAN_POINT ( 'NONE',  ( 6.775403141435218934, -2.126176841940958351, -7.934999999999989839 ) ) ;
#48842=ORIENTED_EDGE ( 'NONE', *, *, #131571, .F. ) ;
#48853=CARTESIAN_POINT ( 'NONE',  ( 8.066639616203772789, 1.633150327867685103, 6.094999999999992646 ) ) ;
#48860=CARTESIAN_POINT ( 'NONE',  ( 6.687069808101886892, -2.126176841940956130, 7.934999999999991616 ) ) ;
#48862=VECTOR ( 'NONE', #140164, 1000.000000000000000 ) ;
#48882=CARTESIAN_POINT ( 'NONE',  ( 25.39999999999999858, 7.464222240803104598E-16, -6.094999999999989093 ) ) ;
#48904=EDGE_CURVE ( 'NONE', #90251, #138592, #57966, .T. ) ;
#48949=EDGE_LOOP ( 'NONE', ( #118290, #50161, #100569, #103047, #84961, #126722 ) ) ;
#48971=( GEOMETRIC_REPRESENTATION_CONTEXT ( 3 ) GLOBAL_UNCERTAINTY_ASSIGNED_CONTEXT ( ( #39050 ) ) GLOBAL_UNIT_ASSIGNED_CONTEXT ( ( #19662, #7335, #107382 ) ) REPRESENTATION_CONTEXT ( 'NONE', 'WORKASPACE' ) );
#48984=ORIENTED_EDGE ( 'NONE', *, *, #51783, .T. ) ;
#48994=CARTESIAN_POINT ( 'NONE',  ( 12.14997294953710849, -4.461849672132299105, 4.461849672132299993 ) ) ;
#49021=VECTOR ( 'NONE', #71695, 1000.000000000000000 ) ;
#49031=CARTESIAN_POINT ( 'NONE',  ( 18.49956980810188867, -3.967499999999998028, -6.871911579029511330 ) ) ;
#49040=UNCERTAINTY_MEASURE_WITH_UNIT (LENGTH_MEASURE( 1.000000000000000082E-05 ), #95115, 'distance_accuracy_value', 'NONE');
#49053=EDGE_LOOP ( 'NONE', ( #104049, #45146, #4872, #119186 ) ) ;
#49068=UNCERTAINTY_MEASURE_WITH_UNIT (LENGTH_MEASURE( 1.000000000000000082E-05 ), #46955, 'distance_accuracy_value', 'NONE');
#49082=CARTESIAN_POINT ( 'NONE',  ( 28.00000000000000355, 0.000000000000000000, 6.094999999999989981 ) ) ;
#49084=SURFACE_SIDE_STYLE ('',( #8873 ) ) ;
#49100=CARTESIAN_POINT ( 'NONE',  ( 25.39999999999999858, 0.000000000000000000, 6.094999999999989093 ) ) ;
#49106=( GEOMETRIC_REPRESENTATION_CONTEXT ( 3 ) GLOBAL_UNCERTAINTY_ASSIGNED_CONTEXT ( ( #99673 ) ) GLOBAL_UNIT_ASSIGNED_CONTEXT ( ( #104116, #42311, #60698 ) ) REPRESENTATION_CONTEXT ( 'NONE', 'WORKASPACE' ) );
#49107=( LENGTH_UNIT ( ) NAMED_UNIT ( * ) SI_UNIT ( .MILLI., .METRE. ) );
#49115=( NAMED_UNIT ( * ) SI_UNIT ( $, .STERADIAN. ) SOLID_ANGLE_UNIT ( ) );
#49189=CARTESIAN_POINT ( 'NONE',  ( 131.6379680400227414, -49.11957940092399610, 40.22172306649564177 ) ) ;
#49204=FILL_AREA_STYLE ('',( #4906 ) ) ;
#49208=CARTESIAN_POINT ( 'NONE',  ( 30.25456980810189123, -6.871911579029512218, 3.967499999999996252 ) ) ;
#49220=CIRCLE ( 'NONE', #120995, 2.552699999999928693 ) ;
#49258=CARTESIAN_POINT ( 'NONE',  ( 28.56206980810188512, -7.934999999999991616, -2.126176841940955242 ) ) ;
#49259=CARTESIAN_POINT ( 'NONE',  ( 9.749569808101886892, 3.967499999999998916, 6.871911579029510442 ) ) ;
#49265=STYLED_ITEM ( 'NONE', ( #21339 ), #100016 ) ;
#49270=MECHANICAL_DESIGN_GEOMETRIC_PRESENTATION_REPRESENTATION('',(#33030),#23790);
#49272=FACE_BOUND ( 'NONE', #133948, .T. ) ;
#49273=CARTESIAN_POINT ( 'NONE',  ( 23.37913961620377279, -5.278424836066145431, -3.047499999999993658 ) ) ;
#49317=CARTESIAN_POINT ( 'NONE',  ( 9.254569808101885897, -6.871911579029512218, 3.967499999999996252 ) ) ;
#49319=CARTESIAN_POINT ( 'NONE',  ( 21.43750000000000000, -4.461849672132299105, 4.461849672132299993 ) ) ;
#49335=CARTESIAN_POINT ( 'NONE',  ( 5.395833333333335702, 1.633150327867692431, -6.094999999999989093 ) ) ;
#49387=( BOUNDED_CURVE ( )  B_SPLINE_CURVE ( 2, ( #27307, #106275, #40376, #96132, #93298, #62837, #5551, #137530, #128776, #29452, #17845, #82432, #61433 ),
 .UNSPECIFIED., .F., .T. ) 
 B_SPLINE_CURVE_WITH_KNOTS ( ( 3, 2, 2, 2, 2, 2, 3 ),
 ( 0.3500000000000000333, 0.3583333333333333925, 0.3666666666666666963, 0.3750000000000001110, 0.3833333333333334703, 0.3916666666666667740, 0.4000000000000001332 ),
 .UNSPECIFIED. ) 
 CURVE ( )  GEOMETRIC_REPRESENTATION_ITEM ( )  RATIONAL_B_SPLINE_CURVE ( ( 0.9999999999999997780, 0.9659258262890685343, 1.000000000000000000, 0.9659258262890683122, 1.000000000000000000, 0.9659258262890683122, 1.000000000000000000, 0.9659258262890683122, 1.000000000000000000, 0.9659258262890683122, 1.000000000000000000, 0.9659258262890678681, 1.000000000000000444 ) ) 
 REPRESENTATION_ITEM ( '' )  );
#49392=CARTESIAN_POINT ( 'NONE',  ( 3.858736474768553304, 5.808823158059031044, -5.808823158059038150 ) ) ;
#49401=FILL_AREA_STYLE ('',( #116754 ) ) ;
#49406=FILL_AREA_STYLE ('',( #47973 ) ) ;
#49412=VERTEX_POINT ( 'NONE', #18510 ) ;
#49466=PRESENTATION_STYLE_ASSIGNMENT (( #117508 ) ) ;
#49488=ORIENTED_EDGE ( 'NONE', *, *, #67762, .T. ) ;
#49524=SURFACE_SIDE_STYLE ('',( #3788 ) ) ;
#49536=EDGE_CURVE ( 'NONE', #96891, #47238, #58371, .T. ) ;
#49542=CARTESIAN_POINT ( 'NONE',  ( 15.75000000000000000, -7.464222240803106570E-16, -6.094999999999989981 ) ) ;
#49548=ORIENTED_EDGE ( 'NONE', *, *, #60269, .T. ) ;
#49561=CARTESIAN_POINT ( 'NONE',  ( 11.00456980810188590, 6.871911579029510442, -3.967499999999998916 ) ) ;
#49570=CARTESIAN_POINT ( 'NONE',  ( 11.56663961620377279, 1.633150327867675555, 6.094999999999998863 ) ) ;
#49588=SURFACE_STYLE_FILL_AREA ( #14778 ) ;
#49595=CARTESIAN_POINT ( 'NONE',  ( 4.062069808101886004, -7.934999999999991616, -2.126176841940955242 ) ) ;
#49597=AXIS2_PLACEMENT_3D ( 'NONE', #88779, #102511, #35118 ) ;
#49605=AXIS2_PLACEMENT_3D ( 'NONE', #7662, #29419, #85956 ) ;
#49608=( BOUNDED_CURVE ( )  B_SPLINE_CURVE ( 2, ( #33477, #67528, #56675, #87111, #21129, #121847, #111723, #12389, #100837, #43599, #109569 ),
 .UNSPECIFIED., .F., .F. ) 
 B_SPLINE_CURVE_WITH_KNOTS ( ( 3, 2, 2, 2, 2, 3 ),
 ( 0.7500000000000001110, 0.7583333333333334147, 0.7666666666666668295, 0.7750000000000000222, 0.7833333333333333259, 0.7910556609953053320 ),
 .UNSPECIFIED. ) 
 CURVE ( )  GEOMETRIC_REPRESENTATION_ITEM ( )  RATIONAL_B_SPLINE_CURVE ( ( 0.9999999999999995559, 0.9659258262890687563, 1.000000000000000000, 0.9659258262890683122, 1.000000000000000000, 0.9659258262890683122, 1.000000000000000000, 0.9659258262890683122, 1.000000000000000000, 0.9684241678951878152, 0.9953696770014417439 ) ) 
 REPRESENTATION_ITEM ( '' )  );
#49610=EDGE_CURVE ( 'NONE', #51562, #19565, #35162, .T. ) ;
#49625=PRESENTATION_STYLE_ASSIGNMENT (( #16203 ) ) ;
#49666=( GEOMETRIC_REPRESENTATION_CONTEXT ( 3 ) GLOBAL_UNCERTAINTY_ASSIGNED_CONTEXT ( ( #77950 ) ) GLOBAL_UNIT_ASSIGNED_CONTEXT ( ( #117504, #110905, #100779 ) ) REPRESENTATION_CONTEXT ( 'NONE', 'WORKASPACE' ) );
#49688=VERTEX_POINT ( 'NONE', #135874 ) ;
#49725=CARTESIAN_POINT ( 'NONE',  ( 12.00413961620377279, -3.047499999999994547, 5.278424836066145431 ) ) ;
#49740=ORIENTED_EDGE ( 'NONE', *, *, #50219, .F. ) ;
#49764=EDGE_LOOP ( 'NONE', ( #72230, #76710, #23013, #109519 ) ) ;
#49771=CARTESIAN_POINT ( 'NONE',  ( 0.2480159638836071934, -51.74944211519454029, -38.65549799471448011 ) ) ;
#49799=CIRCLE ( 'NONE', #135576, 28.00000000000003197 ) ;
#49800=SURFACE_STYLE_FILL_AREA ( #93267 ) ;
#49806=CARTESIAN_POINT ( 'NONE',  ( 24.06249999999999645, 4.461849672132300881, 4.461849672132299105 ) ) ;
#49835=SURFACE_STYLE_FILL_AREA ( #59980 ) ;
#49850=ADVANCED_FACE ( 'NONE', ( #108021 ), #64552, .T. ) ;
#49864=( NAMED_UNIT ( * ) PLANE_ANGLE_UNIT ( ) SI_UNIT ( $, .RADIAN. ) );
#49912=CARTESIAN_POINT ( 'NONE',  ( 128.8219055147128529, -52.14999999999999147, -41.05261164187028555 ) ) ;
#49914=DIRECTION ( 'NONE',  ( 0.000000000000000000, -1.000000000000000000, 0.000000000000000000 ) ) ;
#49917=CARTESIAN_POINT ( 'NONE',  ( 4.645403141435220817, -2.126176841940958351, -7.934999999999989839 ) ) ;
#49958=CARTESIAN_POINT ( 'NONE',  ( 28.27040314143521726, -7.934999999999989839, 2.126176841940957907 ) ) ;
#49959=CARTESIAN_POINT ( 'NONE',  ( 11.35373647476855297, -5.808823158059035485, -5.808823158059033709 ) ) ;
#49960=DIRECTION ( 'NONE',  ( -1.000000000000000000, 0.000000000000000000, 0.000000000000000000 ) ) ;
#49970=( NAMED_UNIT ( * ) PLANE_ANGLE_UNIT ( ) SI_UNIT ( $, .RADIAN. ) );
#49981=DIRECTION ( 'NONE',  ( 0.000000000000000000, 0.000000000000000000, -1.000000000000000000 ) ) ;
#49993=CARTESIAN_POINT ( 'NONE',  ( 122.6835989386367345, -43.14999999999999147, 34.92499999999998295 ) ) ;
#49995=CARTESIAN_POINT ( 'NONE',  ( 8.020833333333332149, -6.094999999999989981, -1.633150327867689322 ) ) ;
#50016=CARTESIAN_POINT ( 'NONE',  ( 10.71290314143521982, 3.967499999999992699, -6.871911579029513994 ) ) ;
#50062=AXIS2_PLACEMENT_3D ( 'NONE', #96783, #31585, #12659 ) ;
#50087=( LENGTH_UNIT ( ) NAMED_UNIT ( * ) SI_UNIT ( .MILLI., .METRE. ) );
#50110=( NAMED_UNIT ( * ) PLANE_ANGLE_UNIT ( ) SI_UNIT ( $, .RADIAN. ) );
#50116=ORIENTED_EDGE ( 'NONE', *, *, #101650, .T. ) ;
#50161=ORIENTED_EDGE ( 'NONE', *, *, #24011, .T. ) ;
#50168=SURFACE_SIDE_STYLE ('',( #128444 ) ) ;
#50182=AXIS2_PLACEMENT_3D ( 'NONE', #7536, #95982, #76402 ) ;
#50219=EDGE_CURVE ( 'NONE', #61426, #112167, #55663, .T. ) ;
#50253=CARTESIAN_POINT ( 'NONE',  ( 8.525403141435219823, 2.126176841940962348, 7.934999999999989839 ) ) ;
#50287=CARTESIAN_POINT ( 'NONE',  ( 0.4162364747685528554, -7.934999999999990727, 4.858786175617117713E-16 ) ) ;
#50304=ORIENTED_EDGE ( 'NONE', *, *, #39957, .T. ) ;
#50364=CARTESIAN_POINT ( 'NONE',  ( 0.000000000000000000, -57.15000000000003411, 15.92499999999935589 ) ) ;
#50419=CARTESIAN_POINT ( 'NONE',  ( 19.44163961620376924, -6.094999999999989093, 1.633150327867691765 ) ) ;
#50451=CARTESIAN_POINT ( 'NONE',  ( 31.47873647476854941, -5.808823158059033709, 5.808823158059035485 ) ) ;
#50464=( NAMED_UNIT ( * ) SI_UNIT ( $, .STERADIAN. ) SOLID_ANGLE_UNIT ( ) );
#50483=CYLINDRICAL_SURFACE ( 'NONE', #108814, 28.00000000000001776 ) ;
#50494=CARTESIAN_POINT ( 'NONE',  ( 19.39583333333332860, 1.633150327867687324, -6.094999999999991758 ) ) ;
#50495=FILL_AREA_STYLE ('',( #130747 ) ) ;
#50500=ORIENTED_EDGE ( 'NONE', *, *, #111916, .T. ) ;
#50545=ORIENTED_EDGE ( 'NONE', *, *, #118760, .F. ) ;
#50550=( NAMED_UNIT ( * ) PLANE_ANGLE_UNIT ( ) SI_UNIT ( $, .RADIAN. ) );
#50572=CARTESIAN_POINT ( 'NONE',  ( 11.71247294953710671, 0.000000000000000000, 6.094999999999989981 ) ) ;
#50573=VERTEX_POINT ( 'NONE', #88119 ) ;
#50594=( NAMED_UNIT ( * ) PLANE_ANGLE_UNIT ( ) SI_UNIT ( $, .RADIAN. ) );
#50607=CARTESIAN_POINT ( 'NONE',  ( 0.6130698085689265664, -49.19053253528954173, 40.77637019027827137 ) ) ;
#50610=EDGE_CURVE ( 'NONE', #52815, #21857, #9058, .T. ) ;
#50611=CARTESIAN_POINT ( 'NONE',  ( 6.687069808101886004, -2.126176841940956130, 7.934999999999991616 ) ) ;
#50640=UNCERTAINTY_MEASURE_WITH_UNIT (LENGTH_MEASURE( 1.000000000000000082E-05 ), #38963, 'distance_accuracy_value', 'NONE');
#50650=CARTESIAN_POINT ( 'NONE',  ( 32.35373647476855297, -5.808823158059035485, -5.808823158059033709 ) ) ;
#50651=CARTESIAN_POINT ( 'NONE',  ( 4.062069808101884227, -7.934999999999990727, -2.126176841940955242 ) ) ;
#50659=PRESENTATION_STYLE_ASSIGNMENT (( #36924 ) ) ;
#50663=VECTOR ( 'NONE', #77171, 1000.000000000000000 ) ;
#50676=( NAMED_UNIT ( * ) PLANE_ANGLE_UNIT ( ) SI_UNIT ( $, .RADIAN. ) );
#50683=CARTESIAN_POINT ( 'NONE',  ( 56.39204447045845825, -48.22435659090886162, 37.54366622512055329 ) ) ;
#50691=PRESENTATION_STYLE_ASSIGNMENT (( #128264 ) ) ;
#50717=CARTESIAN_POINT ( 'NONE',  ( 13.04623647476855375, -7.934999999999990727, 4.858786175617117713E-16 ) ) ;
#50726=COLOUR_RGB ( '', 0.66274510, 0.83137255, 0.94901961) ;
#50783=CARTESIAN_POINT ( 'NONE',  ( 32.87956980810189123, 3.967499999999998916, 6.871911579029510442 ) ) ;
#50784=CARTESIAN_POINT ( 'NONE',  ( 5.754569808101886785, -6.871911579029512218, 3.967499999999996252 ) ) ;
#50799=CARTESIAN_POINT ( 'NONE',  ( 183.4813685602576925, -52.14999999947626463, -41.03936837847464858 ) ) ;
#50814=CARTESIAN_POINT ( 'NONE',  ( 0.6713702758573106832, -52.14999999999999147, -41.05044666116291552 ) ) ;
#50821=SURFACE_STYLE_USAGE ( .BOTH. , #93609 ) ;
#50836=ORIENTED_EDGE ( 'NONE', *, *, #99334, .F. ) ;
#50839=ORIENTED_EDGE ( 'NONE', *, *, #52176, .F. ) ;
#50842=FILL_AREA_STYLE_COLOUR ( '', #29411 ) ;
#50857=DIRECTION ( 'NONE',  ( 0.000000000000000000, 0.000000000000000000, 1.000000000000000000 ) ) ;
#50862=DIRECTION ( 'NONE',  ( 0.000000000000000000, -1.000000000000000000, 0.000000000000000000 ) ) ;
#50873=( LENGTH_UNIT ( ) NAMED_UNIT ( * ) SI_UNIT ( .MILLI., .METRE. ) );
#50877=ORIENTED_EDGE ( 'NONE', *, *, #36349, .T. ) ;
#50896=CARTESIAN_POINT ( 'NONE',  ( 28.00000000000002487, -52.14999999999999147, 34.92500000000003268 ) ) ;
#50925=SURFACE_STYLE_USAGE ( .BOTH. , #19700 ) ;
#50938=EDGE_LOOP ( 'NONE', ( #98999, #76328, #23114, #35587, #9693 ) ) ;
#50948=VECTOR ( 'NONE', #63974, 1000.000000000000000 ) ;
#50961=CARTESIAN_POINT ( 'NONE',  ( 13.19206980810188412, -7.934999999999991616, -2.126176841940955242 ) ) ;
#50997=CARTESIAN_POINT ( 'NONE',  ( 10.91623647476855297, -7.934999999999990727, 4.858786175617117713E-16 ) ) ;
#51012=EDGE_LOOP ( 'NONE', ( #119660, #100823, #14705, #78898 ) ) ;
#51024=CARTESIAN_POINT ( 'NONE',  ( 1.942999468602176316, 2.238834683357417088, -5.749481961982899847 ) ) ;
#51052=CARTESIAN_POINT ( 'NONE',  ( 181.1500000000000057, -43.14999999999999147, 31.92499999999998295 ) ) ;
#51123=EDGE_LOOP ( 'NONE', ( #62159, #67963, #11137, #27951 ) ) ;
#51134=CARTESIAN_POINT ( 'NONE',  ( 18.27497294953710494, 4.461849672132300881, 4.461849672132299105 ) ) ;
#51153=CARTESIAN_POINT ( 'NONE',  ( 24.39999999999999858, -2.600000000000055600, -28.92500000000001492 ) ) ;
#51171=ORIENTED_EDGE ( 'NONE', *, *, #65291, .F. ) ;
#51177=CARTESIAN_POINT ( 'NONE',  ( 2.999999998680793478, -47.86718710719738112, -37.19897551713944495 ) ) ;
#51179=EDGE_CURVE ( 'NONE', #90251, #9331, #113405, .T. ) ;
#51214=CARTESIAN_POINT ( 'NONE',  ( 31.06250000000000000, 4.461849672132300881, 4.461849672132299105 ) ) ;
#51233=EDGE_CURVE ( 'NONE', #115565, #52479, #85561, .T. ) ;
#51234=DIRECTION ( 'NONE',  ( -1.000000000000000000, -0.000000000000000000, -0.000000000000000000 ) ) ;
#51272=DIRECTION ( 'NONE',  ( 1.000000000000000000, 0.000000000000000000, 0.000000000000000000 ) ) ;
#51300=CARTESIAN_POINT ( 'NONE',  ( 13.46247294953710494, -7.464222240803106570E-16, -6.094999999999989981 ) ) ;
#51313=PRESENTATION_STYLE_ASSIGNMENT (( #114411 ) ) ;
#51332=FACE_OUTER_BOUND ( 'NONE', #138677, .T. ) ;
#51335=CARTESIAN_POINT ( 'NONE',  ( 7.416236474768552078, -7.934999999999990727, 4.858786175617117713E-16 ) ) ;
#51342=STYLED_ITEM ( 'NONE', ( #52988 ), #23446 ) ;
#51378=CARTESIAN_POINT ( 'NONE',  ( 8.166666666666667851, -5.278424836066145431, -3.047499999999993658 ) ) ;
#51379=CARTESIAN_POINT ( 'NONE',  ( 10.47873647476855119, -5.808823158059033709, 5.808823158059035485 ) ) ;
#51401=DIRECTION ( 'NONE',  ( 0.000000000000000000, -1.000000000000000000, 0.000000000000000000 ) ) ;
#51412=CARTESIAN_POINT ( 'NONE',  ( 53.94409967708047304, -48.16486758952285641, 37.61253110040706815 ) ) ;
#51418=SURFACE_STYLE_FILL_AREA ( #126122 ) ;
#51440=CARTESIAN_POINT ( 'NONE',  ( 5.462903141435219823, -3.967499999999994476, 6.871911579029513106 ) ) ;
#51459=PRESENTATION_STYLE_ASSIGNMENT (( #63068 ) ) ;
#51500=SURFACE_STYLE_FILL_AREA ( #31874 ) ;
#51512=CARTESIAN_POINT ( 'NONE',  ( 13.48373647476855375, -5.808823158059035485, -5.808823158059033709 ) ) ;
#51517=DIRECTION ( 'NONE',  ( 0.000000000000000000, -1.000000000000000000, 0.000000000000000000 ) ) ;
#51522=DIRECTION ( 'NONE',  ( 1.000000000000000000, 0.000000000000000000, 0.000000000000000000 ) ) ;
#51535=AXIS2_PLACEMENT_3D ( 'NONE', #51052, #138780, #117003 ) ;
#51551=CARTESIAN_POINT ( 'NONE',  ( 2.916666666666666963, 5.278424836066147208, 3.047499999999990550 ) ) ;
#51562=VERTEX_POINT ( 'NONE', #18941 ) ;
#51596=MECHANICAL_DESIGN_GEOMETRIC_PRESENTATION_REPRESENTATION('',(#77059),#39082);
#51602=AXIS2_PLACEMENT_3D ( 'NONE', #6834, #95314, #68781 ) ;
#51617=DIRECTION ( 'NONE',  ( 0.000000000000000000, -0.000000000000000000, -1.000000000000000000 ) ) ;
#51634=( LENGTH_UNIT ( ) NAMED_UNIT ( * ) SI_UNIT ( .MILLI., .METRE. ) );
#51665=CARTESIAN_POINT ( 'NONE',  ( 19.73330628287043709, -6.094999999999989981, -1.633150327867689322 ) ) ;
#51677=PRESENTATION_STYLE_ASSIGNMENT (( #116913 ) ) ;
#51680=CARTESIAN_POINT ( 'NONE',  ( 16.54623647476855552, -7.934999999999990727, 4.858786175617117713E-16 ) ) ;
#51691=CARTESIAN_POINT ( 'NONE',  ( 10.83747294953710671, 6.094999999999989981, -1.119633336120465690E-15 ) ) ;
#51708=AXIS2_PLACEMENT_3D ( 'NONE', #113880, #58119, #5080 ) ;
#51716=CARTESIAN_POINT ( 'NONE',  ( 3.730677800976790248, -49.14999999999999147, 40.92499999999998295 ) ) ;
#51718=CARTESIAN_POINT ( 'NONE',  ( 13.97873647476855119, -5.808823158059033709, 5.808823158059035485 ) ) ;
#51757=CARTESIAN_POINT ( 'NONE',  ( 0.000000000000000000, -5.520864266206504263E-14, 0.000000000000000000 ) ) ;
#51764=( NAMED_UNIT ( * ) PLANE_ANGLE_UNIT ( ) SI_UNIT ( $, .RADIAN. ) );
#51776=CARTESIAN_POINT ( 'NONE',  ( 2.999999999999999112, -1.600000000000013634, 20.40202195861969159 ) ) ;
#51783=EDGE_CURVE ( 'NONE', #105463, #112966, #49387, .T. ) ;
#51786=DIRECTION ( 'NONE',  ( 0.9707728879609256456, 0.000000000000000000, -0.2400000000000085398 ) ) ;
#51787=MECHANICAL_DESIGN_GEOMETRIC_PRESENTATION_REPRESENTATION('',(#142027),#125873);
#51802=SURFACE_STYLE_USAGE ( .BOTH. , #19853 ) ;
#51818=CIRCLE ( 'NONE', #37951, 2.999999999999999112 ) ;
#51836=CARTESIAN_POINT ( 'NONE',  ( 180.8471172286433273, -48.98543874033772738, -39.51758185027073011 ) ) ;
#51852=CARTESIAN_POINT ( 'NONE',  ( 19.29580628287044064, -5.278424836066144543, 3.047499999999995879 ) ) ;
#51888=CARTESIAN_POINT ( 'NONE',  ( 32.06206980810188867, -7.934999999999991616, -2.126176841940955242 ) ) ;
#51900=CARTESIAN_POINT ( 'NONE',  ( 3.010427959778297691, -48.08977582060965261, -37.49964900842701354 ) ) ;
#51933=CARTESIAN_POINT ( 'NONE',  ( 33.39583333333333570, 1.633150327867687324, -6.094999999999991758 ) ) ;
#51942=CARTESIAN_POINT ( 'NONE',  ( 52.60764783923754351, -49.05583548141699168, -39.86617647058817937 ) ) ;
#51953=CARTESIAN_POINT ( 'NONE',  ( 1.649863965247968967, -3.804504390074225917, 5.216255841094045387 ) ) ;
#51969=ADVANCED_FACE ( 'NONE', ( #107726 ), #84515, .T. ) ;
#51980=CARTESIAN_POINT ( 'NONE',  ( 25.40000000000000568, -5.414183704902473693, -5.631019616293379215 ) ) ;
#52032=DIRECTION ( 'NONE',  ( 0.000000000000000000, 0.000000000000000000, -1.000000000000000000 ) ) ;
#52038=CARTESIAN_POINT ( 'NONE',  ( 0.3619179557511837397, -48.99280962439293319, 39.49606053969938557 ) ) ;
#52043=CARTESIAN_POINT ( 'NONE',  ( 0.9995698081018860037, -3.967499999999998028, -6.871911579029511330 ) ) ;
#52083=CARTESIAN_POINT ( 'NONE',  ( 7.437500000000000000, -4.461849672132299105, 4.461849672132299993 ) ) ;
#52084=CARTESIAN_POINT ( 'NONE',  ( 12.95790314143521904, 6.871911579029515771, 3.967499999999989146 ) ) ;
#52098=CARTESIAN_POINT ( 'NONE',  ( 0.3394530118782065897, -51.90335959434332835, 39.28179725402794276 ) ) ;
#52102=FILL_AREA_STYLE ('',( #10707 ) ) ;
#52106=CARTESIAN_POINT ( 'NONE',  ( 58.54058136200207230, -46.07581969935849742, 35.63601533998080839 ) ) ;
#52114=CARTESIAN_POINT ( 'NONE',  ( 124.7734390271609328, -44.54322672567447228, 35.04755940937926084 ) ) ;
#52119=( BOUNDED_CURVE ( )  B_SPLINE_CURVE ( 2, ( #60181, #104356, #5021, #49319, #93506, #18778, #73898, #117366, #52136, #40564, #118066, #128979, #129684 ),
 .UNSPECIFIED., .F., .F. ) 
 B_SPLINE_CURVE_WITH_KNOTS ( ( 3, 2, 2, 2, 2, 2, 3 ),
 ( 0.6000000000000000888, 0.6083333333333333925, 0.6166666666666668073, 0.6250000000000001110, 0.6333333333333334147, 0.6416666666666668295, 0.6500000000000001332 ),
 .UNSPECIFIED. ) 
 CURVE ( )  GEOMETRIC_REPRESENTATION_ITEM ( )  RATIONAL_B_SPLINE_CURVE ( ( 0.9999999999999995559, 0.9659258262890687563, 1.000000000000000000, 0.9659258262890683122, 1.000000000000000000, 0.9659258262890683122, 1.000000000000000000, 0.9659258262890683122, 1.000000000000000000, 0.9659258262890683122, 1.000000000000000000, 0.9659258262890678681, 1.000000000000000444 ) ) 
 REPRESENTATION_ITEM ( '' )  );
#52135=CARTESIAN_POINT ( 'NONE',  ( 9.692069808101887674, -7.934999999999990727, -2.126176841940955242 ) ) ;
#52136=CARTESIAN_POINT ( 'NONE',  ( 22.16666666666666785, -5.278424836066145431, -3.047499999999993658 ) ) ;
#52137=AXIS2_PLACEMENT_3D ( 'NONE', #65150, #42685, #10021 ) ;
#52176=EDGE_CURVE ( 'NONE', #58880, #96438, #103972, .T. ) ;
#52201=CARTESIAN_POINT ( 'NONE',  ( 9.400403141435219823, -7.934999999999989839, 2.126176841940957907 ) ) ;
#52202=ORIENTED_EDGE ( 'NONE', *, *, #94553, .F. ) ;
#52213=CARTESIAN_POINT ( 'NONE',  ( 0.000000000000000000, -49.85820393249939286, 34.92500000000001847 ) ) ;
#52234=DIRECTION ( 'NONE',  ( 0.000000000000000000, -1.000000000000000000, 0.000000000000000000 ) ) ;
#52258=ORIENTED_EDGE ( 'NONE', *, *, #20545, .F. ) ;
#52259=CARTESIAN_POINT ( 'NONE',  ( 25.39999999999999858, -2.600000000000013856, 20.40202195861968448 ) ) ;
#52292=DIRECTION ( 'NONE',  ( 0.000000000000000000, 0.000000000000000000, 1.000000000000000000 ) ) ;
#52345=FACE_OUTER_BOUND ( 'NONE', #142253, .T. ) ;
#52368=CARTESIAN_POINT ( 'NONE',  ( 22.67123647476855552, 0.000000000000000000, 7.934999999999990727 ) ) ;
#52372=EDGE_CURVE ( 'NONE', #112966, #108472, #69706, .T. ) ;
#52377=AXIS2_PLACEMENT_3D ( 'NONE', #372, #3746, #11233 ) ;
#52379=ORIENTED_EDGE ( 'NONE', *, *, #120168, .F. ) ;
#52398=CARTESIAN_POINT ( 'NONE',  ( 14.27040314143522082, -7.934999999999989839, 2.126176841940957907 ) ) ;
#52406=( LENGTH_UNIT ( ) NAMED_UNIT ( * ) SI_UNIT ( .MILLI., .METRE. ) );
#52415=TOROIDAL_SURFACE ( 'NONE', #138115, 2.000000000000000000, 1.000000000000000000 ) ;
#52442=CARTESIAN_POINT ( 'NONE',  ( 181.1500000000000057, -43.14999999999999147, 40.92499999999998295 ) ) ;
#52479=VERTEX_POINT ( 'NONE', #78522 ) ;
#52528=FACE_OUTER_BOUND ( 'NONE', #118872, .T. ) ;
#52540=CARTESIAN_POINT ( 'NONE',  ( 22.21247294953710494, 0.000000000000000000, 6.094999999999989981 ) ) ;
#52572=CARTESIAN_POINT ( 'NONE',  ( 33.22873647476855297, 5.808823158059031044, -5.808823158059038150 ) ) ;
#52618=CARTESIAN_POINT ( 'NONE',  ( 31.79166666666666785, -3.047499999999994547, 5.278424836066145431 ) ) ;
#52628=AXIS2_PLACEMENT_3D ( 'NONE', #128119, #29484, #117894 ) ;
#52634=CARTESIAN_POINT ( 'NONE',  ( 128.8216926156730722, -52.14999999996970814, -41.05175048930497184 ) ) ;
#52641=ORIENTED_EDGE ( 'NONE', *, *, #37132, .T. ) ;
#52678=( BOUNDED_CURVE ( )  B_SPLINE_CURVE ( 2, ( #80886, #1824, #133138, #33816, #45422, #22879, #35258, #67148, #111340, #100496, #1141, #89598, #133828 ),
 .UNSPECIFIED., .F., .T. ) 
 B_SPLINE_CURVE_WITH_KNOTS ( ( 3, 2, 2, 2, 2, 2, 3 ),
 ( 0.1500000000000000222, 0.1583333333333333537, 0.1666666666666666852, 0.1750000000000000444, 0.1833333333333333759, 0.1916666666666667351, 0.2000000000000000666 ),
 .UNSPECIFIED. ) 
 CURVE ( )  GEOMETRIC_REPRESENTATION_ITEM ( )  RATIONAL_B_SPLINE_CURVE ( ( 0.9999999999999998890, 0.9659258262890684232, 1.000000000000000000, 0.9659258262890683122, 1.000000000000000000, 0.9659258262890683122, 1.000000000000000000, 0.9659258262890683122, 1.000000000000000000, 0.9659258262890683122, 1.000000000000000000, 0.9659258262890680902, 1.000000000000000222 ) ) 
 REPRESENTATION_ITEM ( '' )  );
#52681=CARTESIAN_POINT ( 'NONE',  ( 183.9257687383401105, -48.73293412427400284, 38.67339632249573356 ) ) ;
#52687=EDGE_CURVE ( 'NONE', #33206, #97401, #64614, .T. ) ;
#52724=STYLED_ITEM ( 'NONE', ( #107755 ), #111895 ) ;
#52728=CARTESIAN_POINT ( 'NONE',  ( 3.340980275923999709, -49.02095135882318999, 39.67421197283140089 ) ) ;
#52732=CARTESIAN_POINT ( 'NONE',  ( 3.916236474768552522, -7.934999999999990727, 4.858786175617117713E-16 ) ) ;
#52764=PRESENTATION_STYLE_ASSIGNMENT (( #63689 ) ) ;
#52771=CARTESIAN_POINT ( 'NONE',  ( 0.5833333333333334814, -5.278424836066144543, 3.047499999999995879 ) ) ;
#52772=CARTESIAN_POINT ( 'NONE',  ( 19.08290314143522437, 3.967499999999992699, -6.871911579029513994 ) ) ;
#52787=FILL_AREA_STYLE_COLOUR ( '', #5449 ) ;
#52794=CARTESIAN_POINT ( 'NONE',  ( 57.48282408945818389, -47.13357697190487983, 36.34567044386079715 ) ) ;
#52800=ORIENTED_EDGE ( 'NONE', *, *, #13040, .F. ) ;
#52802=CARTESIAN_POINT ( 'NONE',  ( 126.6671759105294939, -47.13357697190737383, 36.34567044387055290 ) ) ;
#52815=VERTEX_POINT ( 'NONE', #120374 ) ;
#52823=CARTESIAN_POINT ( 'NONE',  ( 20.48373647476854842, -5.808823158059035485, -5.808823158059033709 ) ) ;
#52828=DIRECTION ( 'NONE',  ( 0.000000000000000000, 0.000000000000000000, 1.000000000000000000 ) ) ;
#52836=CARTESIAN_POINT ( 'NONE',  ( 17.79166666666666785, -3.047499999999994547, 5.278424836066145431 ) ) ;
#52840=SURFACE_SIDE_STYLE ('',( #118830 ) ) ;
#52845=VECTOR ( 'NONE', #97305, 1000.000000000000000 ) ;
#52846=PRESENTATION_STYLE_ASSIGNMENT (( #76060 ) ) ;
#52849=CARTESIAN_POINT ( 'NONE',  ( 25.39999999999999503, 5.312365556086702689, -5.908453331706006395 ) ) ;
#52881=EDGE_CURVE ( 'NONE', #45028, #94854, #13820, .T. ) ;
#52887=CARTESIAN_POINT ( 'NONE',  ( 6.775403141435218934, -2.126176841940958351, -7.934999999999989839 ) ) ;
#52917=CARTESIAN_POINT ( 'NONE',  ( 0.5457257104438988371, -52.10338527932239572, -40.45859298138255866 ) ) ;
#52929=EDGE_CURVE ( 'NONE', #105140, #6561, #4503, .T. ) ;
#52976=ORIENTED_EDGE ( 'NONE', *, *, #66984, .T. ) ;
#52988=PRESENTATION_STYLE_ASSIGNMENT (( #72677 ) ) ;
#53071=CARTESIAN_POINT ( 'NONE',  ( 15.67123647476855552, 0.000000000000000000, 7.934999999999990727 ) ) ;
#53080=DIRECTION ( 'NONE',  ( -1.000000000000000000, -0.000000000000000000, -0.000000000000000000 ) ) ;
#53083=LINE ( 'NONE', #130692, #123424 ) ;
#53093=CARTESIAN_POINT ( 'NONE',  ( 3.791666666666666963, -3.047499999999994547, 5.278424836066145431 ) ) ;
#53097=APPLICATION_CONTEXT ( 'automotive_design' ) ;
#53103=CARTESIAN_POINT ( 'NONE',  ( 15.58290314143522082, 3.967499999999992699, -6.871911579029513994 ) ) ;
#53109=FILL_AREA_STYLE ('',( #85746 ) ) ;
#53111=CARTESIAN_POINT ( 'NONE',  ( 6.316639616203773677, -1.633150327867691765, -6.094999999999989093 ) ) ;
#53141=( BOUNDED_SURFACE ( )  B_SPLINE_SURFACE ( 1, 2, ( 
 ( #126203, #124769, #60254, #103698, #91444, #116013, #4344, #48648, #26880, #58134, #127636, #27582, #36346, #68984, #58863, #92845, #137808, #2979, #94274, #3662, #137081, #39197, #104430, #38483, #14581, #26183, #60996, #37783, #113163, #113893, #13837, #80574, #47273, #25440, #82706, #37044, #5091, #81292, #15962, #49392, #93575, #126885, #69710, #102331, #103023, #47959, #92123, #125496, #7237, #107977, #28329, #85522, #50784, #117431, #62390, #64510, #97858, #73965, #61683, #52887, #18106, #86974, #108685, #17426, #84159, #142097, #30461, #75398, #7962, #40634, #118142, #116745, #39940, #107291, #119573, #9372, #130504, #52201, #118883, #20269, #18849, #73267, #53647, #96390, #141350, #139956, #31183, #42783, #63116, #6503, #105844, #72590, #19571, #94972, #84837, #129044, #86280, #139245, #8650, #63815, #140628, #128358, #29030, #41314, #106553, #51512, #97090, #95704, #42066, #29716, #129760, #74702, #33357, #122442, #11519, #67392, #134062, #99246, #98558, #45646, #78259, #32616, #65976, #666, #131922, #2063, #66665, #121725, #110133, #77555, #112312, #22401, #110829, #54383, #10813, #20991, #55076, #31884, #55800, #57238, #76848, #23107, #68134, #34044, #111581, #46374, #78988, #12260, #121023, #100002, #21722, #143488, #123196, #133352, #56547, #131197, #12961, #76105, #23869, #44209, #101412, #120274, #100718, #142785, #1363, #10122, #88425, #65254, #132665, #44957, #89820, #109437, #43476, #34751, #87688, #89134, #14413, #4174, #27403, #82529, #126046, #16528, #69535, #26712, #93399, #115109, #48465, #3501, #58695, #135496, #124600, #70954, #103535, #81118, #115824, #79727, #47105, #102864, #47793, #37605, #114432, #136904, #125321, #92665, #15780, #57958, #91966, #25275, #60817, #136186, #123910, #36864, #102153, #15100, #91291, #60076, #104245, #81852, #4910, #126717, #49208, #137636, #113724, #2808, #134797, #36180, #71658, #35494, #38314, #80410, #104979, #26010, #5645, #70276, #90560, #24568, #59378, #68824, #112997, #13664, #75242 ),
 ( #119401, #95523, #83241, #74525, #39759, #108513, #86097, #39018, #105671, #20097, #52043, #96925, #29550, #62216, #139790, #138337, #61523, #128871, #141168, #130327, #8480, #73790, #140461, #41883, #40470, #94794, #31017, #117960, #19401, #17940, #52732, #64344, #84668, #28148, #127447, #49917, #41152, #72408, #106371, #7054, #107816, #94095, #129578, #85359, #18663, #116577, #6333, #62939, #17260, #50611, #30278, #139055, #83987, #118708, #51335, #128189, #28864, #73102, #117258, #107114, #7790, #63653, #96219, #88242, #99077, #88969, #54217, #22934, #45475, #34575, #76672, #10642, #22231, #65077, #484, #54907, #31711, #12083, #44025, #143320, #66496, #141928, #67958, #111395, #75933, #9190, #142620, #132494, #78084, #86816, #89653, #87522, #33181, #133882, #44778, #122263, #98403, #109973, #56367, #77393, #123010, #43311, #100546, #120107, #131032, #20817, #67199, #120845, #133190, #21552, #11342, #121559, #110660, #55617, #109266, #78796, #131749, #99819, #23686, #33867, #1194, #9945, #32435, #42619, #65814, #53465, #97674, #38152, #13495, #4014, #49031, #14937, #92493, #27239, #59903, #136720, #112830, #136013, #2630, #36018, #104072, #114263, #48294, #112143, #93226, #12791, #4727, #124425, #137459, #82371, #59214, #35313, #37433, #134616, #101963, #101242, #57778, #113534, #103362, #126550, #57065, #125876, #26548, #68645, #80239, #25825, #1881, #46193, #81672, #90367, #91114, #70789, #114935, #15613, #70100, #25097, #69356, #46928, #135332, #79553, #125136, #102692, #123742, #24398, #14235, #58520, #3338, #47624, #36695, #91789, #80941, #73625, #140305, #38852, #39585, #105510, #41707, #117104, #60649, #83820, #83075, #95361, #27975, #40995, #96066, #18488, #85194, #63494, #129415, #7623, #6174, #127273, #115653, #17101, #107664, #16346, #30103, #61367, #141002, #50451, #19239, #138896, #85920, #51888, #74352, #8322, #118540, #72245, #17779, #62763, #139629, #52572, #96753, #128027, #116413, #130160, #106950, #94637, #28707, #84517, #72952 ) ),
 .UNSPECIFIED., .F., .F., .F. ) 
 B_SPLINE_SURFACE_WITH_KNOTS ( ( 2, 2 ),
 ( 3, 2, 2, 2, 2, 2, 2, 2, 2, 2, 2, 2, 2, 2, 2, 2, 2, 2, 2, 2, 2, 2, 2, 2, 2, 2, 2, 2, 2, 2, 2, 2, 2, 2, 2, 2, 2, 2, 2, 2, 2, 2, 2, 2, 2, 2, 2, 2, 2, 2, 2, 2, 2, 2, 2, 2, 2, 2, 2, 2, 2, 2, 2, 2, 2, 2, 2, 2, 2, 2, 2, 2, 2, 2, 2, 2, 2, 2, 2, 2, 2, 2, 2, 2, 2, 2, 2, 2, 2, 2, 2, 2, 2, 2, 2, 2, 2, 2, 2, 2, 2, 2, 2, 2, 2, 2, 2, 2, 2, 2, 2, 2, 2, 2, 2, 2, 2, 2, 2, 2, 3 ),
 ( 0.000000000000000000, 1.000000000000000000 ),
 ( 0.000000000000000000, 0.008333333333333333218, 0.01666666666666666644, 0.02500000000000000139, 0.03333333333333333287, 0.04166666666666666435, 0.05000000000000000278, 0.05833333333333333426, 0.06666666666666666574, 0.07499999999999999722, 0.08333333333333332871, 0.09166666666666666019, 0.1000000000000000056, 0.1083333333333333370, 0.1166666666666666685, 0.1250000000000000000, 0.1333333333333333315, 0.1416666666666666630, 0.1499999999999999944, 0.1583333333333333259, 0.1666666666666666574, 0.1749999999999999889, 0.1833333333333333204, 0.1916666666666666796, 0.2000000000000000111, 0.2083333333333333426, 0.2166666666666666741, 0.2250000000000000056, 0.2333333333333333370, 0.2416666666666666685, 0.2500000000000000000, 0.2583333333333333592, 0.2666666666666666630, 0.2750000000000000222, 0.2833333333333333259, 0.2916666666666666852, 0.2999999999999999889, 0.3083333333333333481, 0.3166666666666666519, 0.3250000000000000111, 0.3333333333333333148, 0.3416666666666666741, 0.3499999999999999778, 0.3583333333333333370, 0.3666666666666666408, 0.3750000000000000000, 0.3833333333333333592, 0.3916666666666666630, 0.4000000000000000222, 0.4083333333333333259, 0.4166666666666666852, 0.4249999999999999889, 0.4333333333333333481, 0.4416666666666666519, 0.4500000000000000111, 0.4583333333333333148, 0.4666666666666666741, 0.4749999999999999778, 0.4833333333333333370, 0.4916666666666666408, 0.5000000000000000000, 0.5083333333333333037, 0.5166666666666667185, 0.5250000000000000222, 0.5333333333333333259, 0.5416666666666666297, 0.5500000000000000444, 0.5583333333333333481, 0.5666666666666666519, 0.5749999999999999556, 0.5833333333333333703, 0.5916666666666666741, 0.5999999999999999778, 0.6083333333333332815, 0.6166666666666666963, 0.6250000000000000000, 0.6333333333333333037, 0.6416666666666667185, 0.6500000000000000222, 0.6583333333333333259, 0.6666666666666666297, 0.6750000000000000444, 0.6833333333333333481, 0.6916666666666666519, 0.6999999999999999556, 0.7083333333333333703, 0.7166666666666666741, 0.7249999999999999778, 0.7333333333333332815, 0.7416666666666666963, 0.7500000000000000000, 0.7583333333333333037, 0.7666666666666667185, 0.7750000000000000222, 0.7833333333333333259, 0.7916666666666666297, 0.8000000000000000444, 0.8083333333333333481, 0.8166666666666666519, 0.8249999999999999556, 0.8333333333333333703, 0.8416666666666666741, 0.8499999999999999778, 0.8583333333333332815, 0.8666666666666666963, 0.8750000000000000000, 0.8833333333333333037, 0.8916666666666667185, 0.9000000000000000222, 0.9083333333333333259, 0.9166666666666666297, 0.9250000000000000444, 0.9333333333333333481, 0.9416666666666666519, 0.9499999999999999556, 0.9583333333333333703, 0.9666666666666666741, 0.9749999999999999778, 0.9833333333333332815, 0.9916666666666666963, 1.000000000000000000 ),
 .UNSPECIFIED. ) 
 GEOMETRIC_REPRESENTATION_ITEM ( )  RATIONAL_B_SPLINE_SURFACE ( (
 ( 1.000000000000000000, 0.9659258262890683122, 1.000000000000000000, 0.9659258262890683122, 1.000000000000000000, 0.9659258262890683122, 1.000000000000000000, 0.9659258262890683122, 1.000000000000000000, 0.9659258262890683122, 1.000000000000000000, 0.9659258262890683122, 1.000000000000000000, 0.9659258262890683122, 1.000000000000000000, 0.9659258262890683122, 1.000000000000000000, 0.9659258262890683122, 1.000000000000000000, 0.9659258262890683122, 1.000000000000000000, 0.9659258262890683122, 1.000000000000000000, 0.9659258262890683122, 1.000000000000000000, 0.9659258262890683122, 1.000000000000000000, 0.9659258262890683122, 1.000000000000000000, 0.9659258262890683122, 1.000000000000000000, 0.9659258262890683122, 1.000000000000000000, 0.9659258262890683122, 1.000000000000000000, 0.9659258262890683122, 1.000000000000000000, 0.9659258262890683122, 1.000000000000000000, 0.9659258262890683122, 1.000000000000000000, 0.9659258262890683122, 1.000000000000000000, 0.9659258262890683122, 1.000000000000000000, 0.9659258262890683122, 1.000000000000000000, 0.9659258262890683122, 1.000000000000000000, 0.9659258262890683122, 1.000000000000000000, 0.9659258262890683122, 1.000000000000000000, 0.9659258262890683122, 1.000000000000000000, 0.9659258262890683122, 1.000000000000000000, 0.9659258262890683122, 1.000000000000000000, 0.9659258262890683122, 1.000000000000000000, 0.9659258262890683122, 1.000000000000000000, 0.9659258262890683122, 1.000000000000000000, 0.9659258262890683122, 1.000000000000000000, 0.9659258262890683122, 1.000000000000000000, 0.9659258262890683122, 1.000000000000000000, 0.9659258262890683122, 1.000000000000000000, 0.9659258262890683122, 1.000000000000000000, 0.9659258262890683122, 1.000000000000000000, 0.9659258262890683122, 1.000000000000000000, 0.9659258262890683122, 1.000000000000000000, 0.9659258262890683122, 1.000000000000000000, 0.9659258262890683122, 1.000000000000000000, 0.9659258262890683122, 1.000000000000000000, 0.9659258262890683122, 1.000000000000000000, 0.9659258262890683122, 1.000000000000000000, 0.9659258262890683122, 1.000000000000000000, 0.9659258262890683122, 1.000000000000000000, 0.9659258262890683122, 1.000000000000000000, 0.9659258262890683122, 1.000000000000000000, 0.9659258262890683122, 1.000000000000000000, 0.9659258262890683122, 1.000000000000000000, 0.9659258262890683122, 1.000000000000000000, 0.9659258262890683122, 1.000000000000000000, 0.9659258262890683122, 1.000000000000000000, 0.9659258262890683122, 1.000000000000000000, 0.9659258262890683122, 1.000000000000000000, 0.9659258262890683122, 1.000000000000000000, 0.9659258262890683122, 1.000000000000000000, 0.9659258262890683122, 1.000000000000000000, 0.9659258262890683122, 1.000000000000000000, 0.9659258262890683122, 1.000000000000000000, 0.9659258262890683122, 1.000000000000000000, 0.9659258262890683122, 1.000000000000000000, 0.9659258262890683122, 1.000000000000000000, 0.9659258262890683122, 1.000000000000000000, 0.9659258262890683122, 1.000000000000000000, 0.9659258262890683122, 1.000000000000000000, 0.9659258262890683122, 1.000000000000000000, 0.9659258262890683122, 1.000000000000000000, 0.9659258262890683122, 1.000000000000000000, 0.9659258262890683122, 1.000000000000000000, 0.9659258262890683122, 1.000000000000000000, 0.9659258262890683122, 1.000000000000000000, 0.9659258262890683122, 1.000000000000000000, 0.9659258262890683122, 1.000000000000000000, 0.9659258262890683122, 1.000000000000000000, 0.9659258262890683122, 1.000000000000000000, 0.9659258262890683122, 1.000000000000000000, 0.9659258262890683122, 1.000000000000000000, 0.9659258262890683122, 1.000000000000000000, 0.9659258262890683122, 1.000000000000000000, 0.9659258262890683122, 1.000000000000000000, 0.9659258262890683122, 1.000000000000000000, 0.9659258262890683122, 1.000000000000000000, 0.9659258262890683122, 1.000000000000000000, 0.9659258262890683122, 1.000000000000000000, 0.9659258262890683122, 1.000000000000000000, 0.9659258262890683122, 1.000000000000000000, 0.9659258262890683122, 1.000000000000000000, 0.9659258262890683122, 1.000000000000000000, 0.9659258262890683122, 1.000000000000000000, 0.9659258262890683122, 1.000000000000000000, 0.9659258262890683122, 1.000000000000000000, 0.9659258262890683122, 1.000000000000000000, 0.9659258262890683122, 1.000000000000000000, 0.9659258262890683122, 1.000000000000000000, 0.9659258262890683122, 1.000000000000000000, 0.9659258262890683122, 1.000000000000000000, 0.9659258262890683122, 1.000000000000000000, 0.9659258262890683122, 1.000000000000000000, 0.9659258262890683122, 1.000000000000000000, 0.9659258262890683122, 1.000000000000000000, 0.9659258262890683122, 1.000000000000000000, 0.9659258262890683122, 1.000000000000000000, 0.9659258262890683122, 1.000000000000000000, 0.9659258262890683122, 1.000000000000000000, 0.9659258262890683122, 1.000000000000000000, 0.9659258262890683122, 1.000000000000000000, 0.9659258262890683122, 1.000000000000000000, 0.9659258262890683122, 1.000000000000000000, 0.9659258262890683122, 1.000000000000000000, 0.9659258262890683122, 1.000000000000000000, 0.9659258262890683122, 1.000000000000000000, 0.9659258262890683122, 1.000000000000000000, 0.9659258262890683122, 1.000000000000000000, 0.9659258262890683122, 1.000000000000000000, 0.9659258262890683122, 1.000000000000000000, 0.9659258262890683122, 1.000000000000000000, 0.9659258262890683122, 1.000000000000000000, 0.9659258262890683122, 1.000000000000000000),
 ( 1.000000000000000000, 0.9659258262890683122, 1.000000000000000000, 0.9659258262890683122, 1.000000000000000000, 0.9659258262890683122, 1.000000000000000000, 0.9659258262890683122, 1.000000000000000000, 0.9659258262890683122, 1.000000000000000000, 0.9659258262890683122, 1.000000000000000000, 0.9659258262890683122, 1.000000000000000000, 0.9659258262890683122, 1.000000000000000000, 0.9659258262890683122, 1.000000000000000000, 0.9659258262890683122, 1.000000000000000000, 0.9659258262890683122, 1.000000000000000000, 0.9659258262890683122, 1.000000000000000000, 0.9659258262890683122, 1.000000000000000000, 0.9659258262890683122, 1.000000000000000000, 0.9659258262890683122, 1.000000000000000000, 0.9659258262890683122, 1.000000000000000000, 0.9659258262890683122, 1.000000000000000000, 0.9659258262890683122, 1.000000000000000000, 0.9659258262890683122, 1.000000000000000000, 0.9659258262890683122, 1.000000000000000000, 0.9659258262890683122, 1.000000000000000000, 0.9659258262890683122, 1.000000000000000000, 0.9659258262890683122, 1.000000000000000000, 0.9659258262890683122, 1.000000000000000000, 0.9659258262890683122, 1.000000000000000000, 0.9659258262890683122, 1.000000000000000000, 0.9659258262890683122, 1.000000000000000000, 0.9659258262890683122, 1.000000000000000000, 0.9659258262890683122, 1.000000000000000000, 0.9659258262890683122, 1.000000000000000000, 0.9659258262890683122, 1.000000000000000000, 0.9659258262890683122, 1.000000000000000000, 0.9659258262890683122, 1.000000000000000000, 0.9659258262890683122, 1.000000000000000000, 0.9659258262890683122, 1.000000000000000000, 0.9659258262890683122, 1.000000000000000000, 0.9659258262890683122, 1.000000000000000000, 0.9659258262890683122, 1.000000000000000000, 0.9659258262890683122, 1.000000000000000000, 0.9659258262890683122, 1.000000000000000000, 0.9659258262890683122, 1.000000000000000000, 0.9659258262890683122, 1.000000000000000000, 0.9659258262890683122, 1.000000000000000000, 0.9659258262890683122, 1.000000000000000000, 0.9659258262890683122, 1.000000000000000000, 0.9659258262890683122, 1.000000000000000000, 0.9659258262890683122, 1.000000000000000000, 0.9659258262890683122, 1.000000000000000000, 0.9659258262890683122, 1.000000000000000000, 0.9659258262890683122, 1.000000000000000000, 0.9659258262890683122, 1.000000000000000000, 0.9659258262890683122, 1.000000000000000000, 0.9659258262890683122, 1.000000000000000000, 0.9659258262890683122, 1.000000000000000000, 0.9659258262890683122, 1.000000000000000000, 0.9659258262890683122, 1.000000000000000000, 0.9659258262890683122, 1.000000000000000000, 0.9659258262890683122, 1.000000000000000000, 0.9659258262890683122, 1.000000000000000000, 0.9659258262890683122, 1.000000000000000000, 0.9659258262890683122, 1.000000000000000000, 0.9659258262890683122, 1.000000000000000000, 0.9659258262890683122, 1.000000000000000000, 0.9659258262890683122, 1.000000000000000000, 0.9659258262890683122, 1.000000000000000000, 0.9659258262890683122, 1.000000000000000000, 0.9659258262890683122, 1.000000000000000000, 0.9659258262890683122, 1.000000000000000000, 0.9659258262890683122, 1.000000000000000000, 0.9659258262890683122, 1.000000000000000000, 0.9659258262890683122, 1.000000000000000000, 0.9659258262890683122, 1.000000000000000000, 0.9659258262890683122, 1.000000000000000000, 0.9659258262890683122, 1.000000000000000000, 0.9659258262890683122, 1.000000000000000000, 0.9659258262890683122, 1.000000000000000000, 0.9659258262890683122, 1.000000000000000000, 0.9659258262890683122, 1.000000000000000000, 0.9659258262890683122, 1.000000000000000000, 0.9659258262890683122, 1.000000000000000000, 0.9659258262890683122, 1.000000000000000000, 0.9659258262890683122, 1.000000000000000000, 0.9659258262890683122, 1.000000000000000000, 0.9659258262890683122, 1.000000000000000000, 0.9659258262890683122, 1.000000000000000000, 0.9659258262890683122, 1.000000000000000000, 0.9659258262890683122, 1.000000000000000000, 0.9659258262890683122, 1.000000000000000000, 0.9659258262890683122, 1.000000000000000000, 0.9659258262890683122, 1.000000000000000000, 0.9659258262890683122, 1.000000000000000000, 0.9659258262890683122, 1.000000000000000000, 0.9659258262890683122, 1.000000000000000000, 0.9659258262890683122, 1.000000000000000000, 0.9659258262890683122, 1.000000000000000000, 0.9659258262890683122, 1.000000000000000000, 0.9659258262890683122, 1.000000000000000000, 0.9659258262890683122, 1.000000000000000000, 0.9659258262890683122, 1.000000000000000000, 0.9659258262890683122, 1.000000000000000000, 0.9659258262890683122, 1.000000000000000000, 0.9659258262890683122, 1.000000000000000000, 0.9659258262890683122, 1.000000000000000000, 0.9659258262890683122, 1.000000000000000000, 0.9659258262890683122, 1.000000000000000000, 0.9659258262890683122, 1.000000000000000000, 0.9659258262890683122, 1.000000000000000000, 0.9659258262890683122, 1.000000000000000000, 0.9659258262890683122, 1.000000000000000000, 0.9659258262890683122, 1.000000000000000000, 0.9659258262890683122, 1.000000000000000000, 0.9659258262890683122, 1.000000000000000000, 0.9659258262890683122, 1.000000000000000000, 0.9659258262890683122, 1.000000000000000000, 0.9659258262890683122, 1.000000000000000000, 0.9659258262890683122, 1.000000000000000000, 0.9659258262890683122, 1.000000000000000000, 0.9659258262890683122, 1.000000000000000000, 0.9659258262890683122, 1.000000000000000000, 0.9659258262890683122, 1.000000000000000000) ) ) 
 REPRESENTATION_ITEM ( '' )  SURFACE ( )  );
#53175=CARTESIAN_POINT ( 'NONE',  ( 8.504139616203772789, -3.047499999999994547, 5.278424836066145431 ) ) ;
#53180=CARTESIAN_POINT ( 'NONE',  ( 15.31250000000000000, -4.461849672132299993, -4.461849672132299105 ) ) ;
#53189=DIRECTION ( 'NONE',  ( 0.000000000000000000, -1.000000000000000000, 0.000000000000000000 ) ) ;
#53191=ORIENTED_EDGE ( 'NONE', *, *, #76877, .F. ) ;
#53195=DIRECTION ( 'NONE',  ( 1.000000000000000000, 0.000000000000000000, 0.000000000000000000 ) ) ;
#53209=DIRECTION ( 'NONE',  ( 0.000000000000000000, 0.000000000000000000, 1.000000000000000000 ) ) ;
#53220=LINE ( 'NONE', #88010, #12394 ) ;
#53227=CIRCLE ( 'NONE', #104228, 28.00000000000003197 ) ;
#53243=CARTESIAN_POINT ( 'NONE',  ( 28.92080628287044064, 3.047499999999997655, 5.278424836066143655 ) ) ;
#53263=STYLED_ITEM ( 'NONE', ( #75114 ), #83137 ) ;
#53265=DIRECTION ( 'NONE',  ( 0.000000000000000000, -1.000000000000000000, 0.000000000000000000 ) ) ;
#53329=CARTESIAN_POINT ( 'NONE',  ( 30.91666666666666785, 5.278424836066147208, 3.047499999999990550 ) ) ;
#53355=CARTESIAN_POINT ( 'NONE',  ( 128.8635666761577738, -49.19207878845100623, -41.22112633374977975 ) ) ;
#53360=CYLINDRICAL_SURFACE ( 'NONE', #99369, 6.094999999999989093 ) ;
#53362=VERTEX_POINT ( 'NONE', #107558 ) ;
#53402=AXIS2_PLACEMENT_3D ( 'NONE', #105731, #39084, #39830 ) ;
#53465=CARTESIAN_POINT ( 'NONE',  ( 17.77040314143522082, -7.934999999999989839, 2.126176841940957907 ) ) ;
#53477=SURFACE_STYLE_FILL_AREA ( #9954 ) ;
#53500=ORIENTED_EDGE ( 'NONE', *, *, #2035, .F. ) ;
#53504=UNCERTAINTY_MEASURE_WITH_UNIT (LENGTH_MEASURE( 1.000000000000000082E-05 ), #69572, 'distance_accuracy_value', 'NONE');
#53511=SURFACE_STYLE_FILL_AREA ( #110700 ) ;
#53512=CARTESIAN_POINT ( 'NONE',  ( 0.000000000000000000, -30.18000000000009564, -15.92500000000064375 ) ) ;
#53515=CARTESIAN_POINT ( 'NONE',  ( 3.937500000000000000, -4.461849672132299105, 4.461849672132299993 ) ) ;
#53517=CARTESIAN_POINT ( 'NONE',  ( 18.64540314143522082, -2.126176841940958351, -7.934999999999988951 ) ) ;
#53518=FILL_AREA_STYLE ('',( #75980 ) ) ;
#53537=ORIENTED_EDGE ( 'NONE', *, *, #119154, .T. ) ;
#53552=CARTESIAN_POINT ( 'NONE',  ( 129.9042113015468374, -47.96374157527412763, 37.32649486623389379 ) ) ;
#53556=CARTESIAN_POINT ( 'NONE',  ( 184.1499999999998352, -50.24077216217763464, 35.40405119785170029 ) ) ;
#53558=MECHANICAL_DESIGN_GEOMETRIC_PRESENTATION_REPRESENTATION('',(#116148),#53668);
#53566=COLOUR_RGB ( '', 0.72549020, 0.75294118, 0.79215686) ;
#53575=CARTESIAN_POINT ( 'NONE',  ( 151.4000000000000057, -17.48000000000005016, 12.69999999999954454 ) ) ;
#53576=CARTESIAN_POINT ( 'NONE',  ( 13.62956980810188767, -3.967499999999998028, -6.871911579029511330 ) ) ;
#53579=CARTESIAN_POINT ( 'NONE',  ( 163.5342603869775076, 26.96999999999993847, 34.56026864331079196 ) ) ;
#53591=STYLED_ITEM ( 'NONE', ( #51459 ), #99140 ) ;
#53605=CARTESIAN_POINT ( 'NONE',  ( 25.40000000000004476, 7.048307320969255052, -3.667349112489660001 ) ) ;
#53647=CARTESIAN_POINT ( 'NONE',  ( 10.12956980810188767, -3.967499999999998028, -6.871911579029511330 ) ) ;
#53668=( GEOMETRIC_REPRESENTATION_CONTEXT ( 3 ) GLOBAL_UNCERTAINTY_ASSIGNED_CONTEXT ( ( #25835 ) ) GLOBAL_UNIT_ASSIGNED_CONTEXT ( ( #68450, #23471, #45272 ) ) REPRESENTATION_CONTEXT ( 'NONE', 'WORKASPACE' ) );
#53695=CARTESIAN_POINT ( 'NONE',  ( 0.1600000000000003919, -1.341267888597242441, -7.849467545898021648 ) ) ;
#53729=CARTESIAN_POINT ( 'NONE',  ( 24.20833333333333570, 3.047499999999997655, 5.278424836066143655 ) ) ;
#53741=CARTESIAN_POINT ( 'NONE',  ( 151.4000000000000057, -18.48000000000005372, 33.92499999999998295 ) ) ;
#53745=DIRECTION ( 'NONE',  ( 1.000000000000000000, -0.000000000000000000, -0.000000000000000000 ) ) ;
#53773=AXIS2_PLACEMENT_3D ( 'NONE', #66479, #14208, #56351 ) ;
#53781=MECHANICAL_DESIGN_GEOMETRIC_PRESENTATION_REPRESENTATION('',(#2831),#102429);
#53802=EDGE_LOOP ( 'NONE', ( #124849, #84673, #48390, #89280 ) ) ;
#53817=CARTESIAN_POINT ( 'NONE',  ( 19.87913961620377279, -5.278424836066145431, -3.047499999999993658 ) ) ;
#53828=CARTESIAN_POINT ( 'NONE',  ( 18.29623647476855197, 7.934999999999990727, -1.457635852685135314E-15 ) ) ;
#53840=MECHANICAL_DESIGN_GEOMETRIC_PRESENTATION_REPRESENTATION('',(#2786),#86326);
#53898=CARTESIAN_POINT ( 'NONE',  ( 131.7497271886881549, -49.14999999999999147, 40.57187971032495000 ) ) ;
#53900=EDGE_CURVE ( 'NONE', #119311, #19621, #58296, .T. ) ;
#53926=ORIENTED_EDGE ( 'NONE', *, *, #5682, .T. ) ;
#53957=VERTEX_POINT ( 'NONE', #90472 ) ;
#53963=CARTESIAN_POINT ( 'NONE',  ( 0.000000000000000000, -7.600000000000055600, -31.92499999999998650 ) ) ;
#53969=CIRCLE ( 'NONE', #79453, 25.00000000000002842 ) ;
#53997=SURFACE_STYLE_USAGE ( .BOTH. , #119205 ) ;
#54009=CARTESIAN_POINT ( 'NONE',  ( 29.06663961620377279, 1.633150327867695095, 6.094999999999988205 ) ) ;
#54020=LINE ( 'NONE', #43128, #95447 ) ;
#54021=AXIS2_PLACEMENT_3D ( 'NONE', #142605, #120822, #43291 ) ;
#54067=FACE_OUTER_BOUND ( 'NONE', #55760, .T. ) ;
#54072=( GEOMETRIC_REPRESENTATION_CONTEXT ( 3 ) GLOBAL_UNCERTAINTY_ASSIGNED_CONTEXT ( ( #80812 ) ) GLOBAL_UNIT_ASSIGNED_CONTEXT ( ( #12780, #57057, #103356 ) ) REPRESENTATION_CONTEXT ( 'NONE', 'WORKASPACE' ) );
#54075=ORIENTED_EDGE ( 'NONE', *, *, #79207, .T. ) ;
#54083=COLOUR_RGB ( '', 0.09019608, 0.27058824, 0.51372549) ;
#54086=CARTESIAN_POINT ( 'NONE',  ( 24.39999999999999858, -5.520864266206504263E-14, 33.92499999999998295 ) ) ;
#54100=CARTESIAN_POINT ( 'NONE',  ( 32.52083333333333570, -6.094999999999989981, -1.633150327867689100 ) ) ;
#54117=CARTESIAN_POINT ( 'NONE',  ( 128.6786164994711612, -49.14501756083436135, -40.36361034346619903 ) ) ;
#54147=CARTESIAN_POINT ( 'NONE',  ( 180.6620941962883933, -49.11927476322659913, 40.22110306067540364 ) ) ;
#54164=CARTESIAN_POINT ( 'NONE',  ( 184.0821179325846799, -51.13011358081449487, 36.94363806876470591 ) ) ;
#54181=ORIENTED_EDGE ( 'NONE', *, *, #123583, .T. ) ;
#54188=CARTESIAN_POINT ( 'NONE',  ( -0.9750270504628943957, -4.461849672132299993, -4.461849672132299105 ) ) ;
#54217=CARTESIAN_POINT ( 'NONE',  ( 9.166236474768552966, 7.934999999999990727, -1.457635852685135314E-15 ) ) ;
#54225=CARTESIAN_POINT ( 'NONE',  ( 20.56249999999999645, 4.461849672132300881, 4.461849672132299105 ) ) ;
#54241=CARTESIAN_POINT ( 'NONE',  ( 18.56663961620377279, 1.633150327867675555, 6.094999999999998863 ) ) ;
#54260=CARTESIAN_POINT ( 'NONE',  ( 6.416666666666666963, 5.278424836066147208, 3.047499999999990550 ) ) ;
#54261=CARTESIAN_POINT ( 'NONE',  ( 20.83290314143522082, -3.967499999999994476, 6.871911579029513106 ) ) ;
#54281=DIRECTION ( 'NONE',  ( 0.000000000000000000, 1.000000000000000000, -4.625929269271485322E-15 ) ) ;
#54312=CARTESIAN_POINT ( 'NONE',  ( 14.21290314143522160, 3.967499999999992699, -6.871911579029513994 ) ) ;
#54314=CIRCLE ( 'NONE', #135329, 2.999999999999992450 ) ;
#54344=FACE_OUTER_BOUND ( 'NONE', #46382, .T. ) ;
#54357=PRESENTATION_STYLE_ASSIGNMENT (( #131887 ) ) ;
#54376=FILL_AREA_STYLE_COLOUR ( '', #43475 ) ;
#54383=CARTESIAN_POINT ( 'NONE',  ( 17.56706980810188767, 2.126176841940952134, -7.934999999999993392 ) ) ;
#54390=ORIENTED_EDGE ( 'NONE', *, *, #106320, .T. ) ;
#54428=DIRECTION ( 'NONE',  ( 0.000000000000000000, 0.000000000000000000, -1.000000000000000000 ) ) ;
#54473=ORIENTED_EDGE ( 'NONE', *, *, #129278, .F. ) ;
#54479=FACE_OUTER_BOUND ( 'NONE', #51123, .T. ) ;
#54487=ORIENTED_EDGE ( 'NONE', *, *, #41429, .T. ) ;
#54495=FACE_OUTER_BOUND ( 'NONE', #60555, .T. ) ;
#54510=CIRCLE ( 'NONE', #140182, 2.999999999999999112 ) ;
#54515=SURFACE_STYLE_FILL_AREA ( #77687 ) ;
#54518=DIRECTION ( 'NONE',  ( 0.000000000000000000, 0.000000000000000000, -1.000000000000000000 ) ) ;
#54523=FACE_OUTER_BOUND ( 'NONE', #89642, .T. ) ;
#54542=CARTESIAN_POINT ( 'NONE',  ( 14.94206980810188590, 7.934999999999993392, 2.126176841940951689 ) ) ;
#54553=LINE ( 'NONE', #10985, #78612 ) ;
#54559=EDGE_LOOP ( 'NONE', ( #54473, #129776, #15539, #123962, #112203 ) ) ;
#54587=( NAMED_UNIT ( * ) PLANE_ANGLE_UNIT ( ) SI_UNIT ( $, .RADIAN. ) );
#54610=DIRECTION ( 'NONE',  ( -1.000000000000000000, -0.000000000000000000, 0.000000000000000000 ) ) ;
#54635=CARTESIAN_POINT ( 'NONE',  ( 14.14583333333333748, -1.633150327867709528, 6.094999999999979323 ) ) ;
#54637=PRESENTATION_STYLE_ASSIGNMENT (( #74240 ) ) ;
#54638=FACE_OUTER_BOUND ( 'NONE', #103054, .T. ) ;
#54675=EDGE_CURVE ( 'NONE', #98477, #53957, #90759, .T. ) ;
#54705=CARTESIAN_POINT ( 'NONE',  ( 2.000000000000008882, 0.000000000000000000, 0.000000000000000000 ) ) ;
#54708=CYLINDRICAL_SURFACE ( 'NONE', #70160, 1.000000000000000888 ) ;
#54709=CARTESIAN_POINT ( 'NONE',  ( 27.17080628287044064, -3.047499999999997211, -5.278424836066143655 ) ) ;
#54767=DIRECTION ( 'NONE',  ( 0.000000000000000000, 0.000000000000000000, 1.000000000000000000 ) ) ;
#54772=DIRECTION ( 'NONE',  ( 0.000000000000000000, 0.000000000000000000, 1.000000000000000000 ) ) ;
#54790=DIRECTION ( 'NONE',  ( 0.000000000000000000, 0.000000000000000000, 1.000000000000000000 ) ) ;
#54796=CARTESIAN_POINT ( 'NONE',  ( 55.45418156660451103, -52.10373894832327579, -40.45955814675560447 ) ) ;
#54836=EDGE_CURVE ( 'NONE', #119600, #100283, #55769, .T. ) ;
#54839=CARTESIAN_POINT ( 'NONE',  ( 180.8041599634935608, -49.02495722182848681, 39.69341335395905190 ) ) ;
#54882=SURFACE_STYLE_FILL_AREA ( #32408 ) ;
#54893=SURFACE_SIDE_STYLE ('',( #127429 ) ) ;
#54907=CARTESIAN_POINT ( 'NONE',  ( 10.47873647476855119, -5.808823158059033709, 5.808823158059035485 ) ) ;
#54911=DIRECTION ( 'NONE',  ( 0.000000000000000000, 0.000000000000000000, -1.000000000000000000 ) ) ;
#54916=( LENGTH_UNIT ( ) NAMED_UNIT ( * ) SI_UNIT ( .MILLI., .METRE. ) );
#54918=UNCERTAINTY_MEASURE_WITH_UNIT (LENGTH_MEASURE( 1.000000000000000082E-05 ), #50873, 'distance_accuracy_value', 'NONE');
#54951=EDGE_CURVE ( 'NONE', #21857, #105963, #85648, .T. ) ;
#54952=( NAMED_UNIT ( * ) SI_UNIT ( $, .STERADIAN. ) SOLID_ANGLE_UNIT ( ) );
#54954=CARTESIAN_POINT ( 'NONE',  ( 24.39999999999999858, -1.600000000000086020, -34.92499999999998295 ) ) ;
#54955=CARTESIAN_POINT ( 'NONE',  ( 13.27083333333333393, 6.094999999999991758, 1.633150327867687102 ) ) ;
#54956=CARTESIAN_POINT ( 'NONE',  ( 15.14540314143521904, -2.126176841940958351, -7.934999999999988951 ) ) ;
#54958=CARTESIAN_POINT ( 'NONE',  ( 0.000000000000000000, 0.9892420537897055333, 14.41609864557725729 ) ) ;
#54967=SURFACE_SIDE_STYLE ('',( #65870 ) ) ;
#54970=CARTESIAN_POINT ( 'NONE',  ( 174.7500000000000000, 7.919999999999947526, -16.42230000000009227 ) ) ;
#55007=AXIS2_PLACEMENT_3D ( 'NONE', #39706, #73731, #83938 ) ;
#55012=CARTESIAN_POINT ( 'NONE',  ( 19.17123647476855197, 0.000000000000000000, 7.934999999999990727 ) ) ;
#55014=CARTESIAN_POINT ( 'NONE',  ( 3.345840036506314785, -49.02495722182847970, -39.69341335395904480 ) ) ;
#55076=CARTESIAN_POINT ( 'NONE',  ( 18.00456980810188767, 6.871911579029510442, -3.967499999999998916 ) ) ;
#55109=UNCERTAINTY_MEASURE_WITH_UNIT (LENGTH_MEASURE( 1.000000000000000082E-05 ), #82033, 'distance_accuracy_value', 'NONE');
#55161=CARTESIAN_POINT ( 'NONE',  ( 24.39999999999999858, -7.600000000000055600, -28.92499999999998650 ) ) ;
#55179=SURFACE_STYLE_USAGE ( .BOTH. , #87086 ) ;
#55190=( NAMED_UNIT ( * ) SI_UNIT ( $, .STERADIAN. ) SOLID_ANGLE_UNIT ( ) );
#55243=CARTESIAN_POINT ( 'NONE',  ( 30.25456980810189123, -6.871911579029512218, 3.967499999999996252 ) ) ;
#55280=LINE ( 'NONE', #64012, #11131 ) ;
#55334=EDGE_CURVE ( 'NONE', #104144, #49412, #135726, .T. ) ;
#55375=CIRCLE ( 'NONE', #32182, 25.00000000000002487 ) ;
#55416=CARTESIAN_POINT ( 'NONE',  ( 24.69163961620376924, 6.094999999999988205, -1.633150327867694651 ) ) ;
#55431=ORIENTED_EDGE ( 'NONE', *, *, #126109, .T. ) ;
#55455=EDGE_CURVE ( 'NONE', #127303, #9331, #58457, .T. ) ;
#55457=PRESENTATION_STYLE_ASSIGNMENT (( #87369 ) ) ;
#55467=CARTESIAN_POINT ( 'NONE',  ( 184.1500000000000057, -57.15000000000009095, 34.92499999999998295 ) ) ;
#55555=SURFACE_SIDE_STYLE ('',( #110602 ) ) ;
#55567=CIRCLE ( 'NONE', #131943, 2.552699999999928693 ) ;
#55573=CARTESIAN_POINT ( 'NONE',  ( 156.1500000000000057, -57.14999999999999147, -53.92499999999968452 ) ) ;
#55594=CARTESIAN_POINT ( 'NONE',  ( -0.3916937171295608033, 1.633150327867687324, -6.094999999999991758 ) ) ;
#55606=EDGE_LOOP ( 'NONE', ( #90015, #125379, #122100, #83117 ) ) ;
#55617=CARTESIAN_POINT ( 'NONE',  ( 16.02040314143522082, 7.934999999999989839, -2.126176841940961904 ) ) ;
#55625=CARTESIAN_POINT ( 'NONE',  ( 20.85416666666666430, 1.633150327867675555, 6.094999999999998863 ) ) ;
#55663=LINE ( 'NONE', #54954, #69351 ) ;
#55664=CARTESIAN_POINT ( 'NONE',  ( 14.43749999999999822, -4.461849672132299105, 4.461849672132299993 ) ) ;
#55665=CARTESIAN_POINT ( 'NONE',  ( 23.45790314143522437, 6.871911579029515771, 3.967499999999989146 ) ) ;
#55682=FILL_AREA_STYLE_COLOUR ( '', #64149 ) ;
#55688=STYLED_ITEM ( 'NONE', ( #22942 ), #81831 ) ;
#55722=LINE ( 'NONE', #53575, #43120 ) ;
#55723=CARTESIAN_POINT ( 'NONE',  ( 15.08790314143521982, 6.871911579029515771, 3.967499999999989146 ) ) ;
#55727=CARTESIAN_POINT ( 'NONE',  ( 165.1810627992761340, 26.96999999999993847, 33.99267764067941755 ) ) ;
#55736=COLOUR_RGB ( '', 0.66274510, 0.83137255, 0.94901961) ;
#55751=SURFACE_STYLE_USAGE ( .BOTH. , #22352 ) ;
#55760=EDGE_LOOP ( 'NONE', ( #2660, #11777, #100213, #108739 ) ) ;
#55766=CARTESIAN_POINT ( 'NONE',  ( 156.1499999999997783, -49.14999999999999147, 34.92500000000004690 ) ) ;
#55769=CIRCLE ( 'NONE', #41885, 28.00000000000003197 ) ;
#55784=CARTESIAN_POINT ( 'NONE',  ( 174.7500000000000000, 7.919999999999947526, 16.57230000000005532 ) ) ;
#55800=CARTESIAN_POINT ( 'NONE',  ( 18.29623647476855197, 7.934999999999990727, -1.457635852685135314E-15 ) ) ;
#55808=MECHANICAL_DESIGN_GEOMETRIC_PRESENTATION_REPRESENTATION('',(#25663),#102160);
#55822=CARTESIAN_POINT ( 'NONE',  ( 25.39999999999999858, -14.29000000000013593, 12.69999999999954632 ) ) ;
#55824=CARTESIAN_POINT ( 'NONE',  ( 25.39999999999999858, -2.600000000000056044, -28.92500000000001492 ) ) ;
#55826=EDGE_LOOP ( 'NONE', ( #45605, #12712, #141358, #54487 ) ) ;
#55844=CARTESIAN_POINT ( 'NONE',  ( 20.97873647476855652, -5.808823158059033709, 5.808823158059035485 ) ) ;
#55846=DIRECTION ( 'NONE',  ( 0.000000000000000000, 0.000000000000000000, -1.000000000000000000 ) ) ;
#55857=ORIENTED_EDGE ( 'NONE', *, *, #96098, .T. ) ;
#55905=FACE_OUTER_BOUND ( 'NONE', #134167, .T. ) ;
#55908=ORIENTED_EDGE ( 'NONE', *, *, #1009, .F. ) ;
#55921=( NAMED_UNIT ( * ) PLANE_ANGLE_UNIT ( ) SI_UNIT ( $, .RADIAN. ) );
#55949=COLOUR_RGB ( '', 0.66274510, 0.83137255, 0.94901961) ;
#55969=STYLED_ITEM ( 'NONE', ( #5814 ), #116311 ) ;
#55979=CARTESIAN_POINT ( 'NONE',  ( 27.62956980810189123, -3.967499999999998028, -6.871911579029511330 ) ) ;
#55981=VERTEX_POINT ( 'NONE', #82856 ) ;
#56049=( NAMED_UNIT ( * ) PLANE_ANGLE_UNIT ( ) SI_UNIT ( $, .RADIAN. ) );
#56052=CARTESIAN_POINT ( 'NONE',  ( 0.9950436184061330902, 5.292275011207155266, 4.751003958219890855 ) ) ;
#56070=STYLED_ITEM ( 'NONE', ( #57754 ), #118359 ) ;
#56074=ORIENTED_EDGE ( 'NONE', *, *, #81751, .F. ) ;
#56075=CARTESIAN_POINT ( 'NONE',  ( 0.1600000000000006695, 2.227659143332861191, -7.636621307949803317 ) ) ;
#56119=DIRECTION ( 'NONE',  ( 0.000000000000000000, 0.000000000000000000, -1.000000000000000000 ) ) ;
#56163=CARTESIAN_POINT ( 'NONE',  ( 30.23330628287044419, -6.094999999999989981, -1.633150327867689100 ) ) ;
#56173=AXIS2_PLACEMENT_3D ( 'NONE', #71770, #115934, #48570 ) ;
#56187=COLOUR_RGB ( '', 0.31764706, 0.68627451, 0.89019608) ;
#56221=DIRECTION ( 'NONE',  ( -0.000000000000000000, 0.000000000000000000, 1.000000000000000000 ) ) ;
#56239=CARTESIAN_POINT ( 'NONE',  ( 16.37913961620377279, -5.278424836066145431, -3.047499999999993658 ) ) ;
#56273=ORIENTED_EDGE ( 'NONE', *, *, #120959, .T. ) ;
#56290=COLOUR_RGB ( '', 0.72549020, 0.75294118, 0.79215686) ;
#56338=CIRCLE ( 'NONE', #58047, 3.000000000000002665 ) ;
#56341=CARTESIAN_POINT ( 'NONE',  ( 4.712472949537106715, 0.000000000000000000, 6.094999999999989981 ) ) ;
#56351=DIRECTION ( 'NONE',  ( 0.000000000000000000, 0.000000000000000000, 1.000000000000000000 ) ) ;
#56367=CARTESIAN_POINT ( 'NONE',  ( 13.83290314143522082, -3.967499999999994476, 6.871911579029513106 ) ) ;
#56368=CARTESIAN_POINT ( 'NONE',  ( 0.000000000000000000, -43.14999999999999147, -40.92499999999998295 ) ) ;
#56376=UNCERTAINTY_MEASURE_WITH_UNIT (LENGTH_MEASURE( 1.000000000000000082E-05 ), #37717, 'distance_accuracy_value', 'NONE');
#56414=CARTESIAN_POINT ( 'NONE',  ( 18.81250000000000355, -4.461849672132299993, -4.461849672132299105 ) ) ;
#56457=AXIS2_PLACEMENT_3D ( 'NONE', #64403, #10017, #54281 ) ;
#56475=CARTESIAN_POINT ( 'NONE',  ( 3.487905803711529806, -49.11927476322659913, -40.22110306067540364 ) ) ;
#56497=( NAMED_UNIT ( * ) PLANE_ANGLE_UNIT ( ) SI_UNIT ( $, .RADIAN. ) );
#56501=VERTEX_POINT ( 'NONE', #82676 ) ;
#56502=FILL_AREA_STYLE ('',( #12214 ) ) ;
#56532=VERTEX_POINT ( 'NONE', #97817 ) ;
#56544=AXIS2_PLACEMENT_3D ( 'NONE', #107943, #8616, #141318 ) ;
#56547=CARTESIAN_POINT ( 'NONE',  ( 20.62956980810188412, -3.967499999999998028, -6.871911579029511330 ) ) ;
#56579=UNCERTAINTY_MEASURE_WITH_UNIT (LENGTH_MEASURE( 1.000000000000000082E-05 ), #38703, 'distance_accuracy_value', 'NONE');
#56590=CARTESIAN_POINT ( 'NONE',  ( 18.64540314143522437, -2.126176841940958351, -7.934999999999989839 ) ) ;
#56645=CARTESIAN_POINT ( 'NONE',  ( 3.567069808101886341, 2.126176841940952134, -7.934999999999992504 ) ) ;
#56647=( GEOMETRIC_REPRESENTATION_CONTEXT ( 3 ) GLOBAL_UNCERTAINTY_ASSIGNED_CONTEXT ( ( #113024 ) ) GLOBAL_UNIT_ASSIGNED_CONTEXT ( ( #133699, #78600, #101045 ) ) REPRESENTATION_CONTEXT ( 'NONE', 'WORKASPACE' ) );
#56675=CARTESIAN_POINT ( 'NONE',  ( 24.25413961620377279, 3.047499999999993214, -5.278424836066146320 ) ) ;
#56676=ORIENTED_EDGE ( 'NONE', *, *, #137035, .T. ) ;
#56682=EDGE_CURVE ( 'NONE', #69422, #46533, #66633, .T. ) ;
#56710=CARTESIAN_POINT ( 'NONE',  ( 23.40040314143521982, -7.934999999999989839, 2.126176841940957907 ) ) ;
#56764=CARTESIAN_POINT ( 'NONE',  ( 0.5388684133533581111, -7.552109465304689628, -0.3911787640923247711 ) ) ;
#56798=( NAMED_UNIT ( * ) PLANE_ANGLE_UNIT ( ) SI_UNIT ( $, .RADIAN. ) );
#56804=CARTESIAN_POINT ( 'NONE',  ( 25.39999999999999858, 0.000000000000000000, 0.000000000000000000 ) ) ;
#56818=COLOUR_RGB ( '', 0.09019608, 0.27058824, 0.51372549) ;
#56855=EDGE_LOOP ( 'NONE', ( #31296, #126900, #25428 ) ) ;
#56877=CARTESIAN_POINT ( 'NONE',  ( 32.27497294953710849, 4.461849672132300881, 4.461849672132299105 ) ) ;
#56901=FILL_AREA_STYLE_COLOUR ( '', #96008 ) ;
#56910=LINE ( 'NONE', #1732, #95569 ) ;
#56928=ORIENTED_EDGE ( 'NONE', *, *, #82275, .F. ) ;
#56979=ORIENTED_EDGE ( 'NONE', *, *, #124972, .T. ) ;
#56996=CARTESIAN_POINT ( 'NONE',  ( 24.39999999999999858, -16.48000000000005016, -34.92499999999998295 ) ) ;
#57018=CARTESIAN_POINT ( 'NONE',  ( 25.39999999999999858, 7.796566843815467607, 1.475727091950665537 ) ) ;
#57026=ORIENTED_EDGE ( 'NONE', *, *, #76877, .T. ) ;
#57036=CARTESIAN_POINT ( 'NONE',  ( 3.983306282870438864, 6.094999999999991758, 1.633150327867687102 ) ) ;
#57057=( NAMED_UNIT ( * ) PLANE_ANGLE_UNIT ( ) SI_UNIT ( $, .RADIAN. ) );
#57065=CARTESIAN_POINT ( 'NONE',  ( 22.87456980810188867, 6.871911579029510442, -3.967499999999998916 ) ) ;
#57094=FILL_AREA_STYLE_COLOUR ( '', #64661 ) ;
#57104=CARTESIAN_POINT ( 'NONE',  ( 2.999999999999999112, -1.600000000000086020, -31.92499999999998295 ) ) ;
#57108=( NAMED_UNIT ( * ) PLANE_ANGLE_UNIT ( ) SI_UNIT ( $, .RADIAN. ) );
#57112=CARTESIAN_POINT ( 'NONE',  ( 10.06250000000000178, 4.461849672132300881, 4.461849672132299105 ) ) ;
#57127=CARTESIAN_POINT ( 'NONE',  ( 126.9785101690948608, -47.44491123045356318, -36.62621018405940276 ) ) ;
#57143=ADVANCED_FACE ( 'NONE', ( #23290 ), #53141, .T. ) ;
#57158=CARTESIAN_POINT ( 'NONE',  ( 152.4000000000000057, -17.48000000000005016, -33.92499999999998295 ) ) ;
#57171=CARTESIAN_POINT ( 'NONE',  ( 23.83790314143521982, -6.871911579029513106, -3.967499999999993587 ) ) ;
#57172=CARTESIAN_POINT ( 'NONE',  ( 25.40000000000000568, -6.088644610809077484, -0.2782657062331916342 ) ) ;
#57176=CARTESIAN_POINT ( 'NONE',  ( 0.000000000000000000, 0.9892420537897061994, -14.41609864557725729 ) ) ;
#57197=DIRECTION ( 'NONE',  ( 0.000000000000000000, 0.000000000000000000, 1.000000000000000000 ) ) ;
#57215=DIRECTION ( 'NONE',  ( -0.000000000000000000, 0.000000000000000000, 1.000000000000000000 ) ) ;
#57238=CARTESIAN_POINT ( 'NONE',  ( 18.44206980810188767, 7.934999999999993392, 2.126176841940951689 ) ) ;
#57246=VERTEX_POINT ( 'NONE', #98923 ) ;
#57261=CARTESIAN_POINT ( 'NONE',  ( 57.90314192168424512, -45.52550609311789032, -35.40428284070723208 ) ) ;
#57268=SURFACE_STYLE_USAGE ( .BOTH. , #2092 ) ;
#57275=CARTESIAN_POINT ( 'NONE',  ( 152.4000000000000057, -17.48000000000005016, 12.69999999999954632 ) ) ;
#57282=CARTESIAN_POINT ( 'NONE',  ( 18.49956980810188867, -3.967499999999998028, -6.871911579029511330 ) ) ;
#57333=ORIENTED_EDGE ( 'NONE', *, *, #55455, .T. ) ;
#57335=CARTESIAN_POINT ( 'NONE',  ( 1.671236474768553082, 0.000000000000000000, 7.934999999999990727 ) ) ;
#57370=EDGE_LOOP ( 'NONE', ( #63568, #79404, #122813 ) ) ;
#57379=PRESENTATION_STYLE_ASSIGNMENT (( #125477 ) ) ;
#57384=EDGE_LOOP ( 'NONE', ( #114896, #33522, #114009, #1484 ) ) ;
#57395=CARTESIAN_POINT ( 'NONE',  ( 29.67123647476855552, 0.000000000000000000, 7.934999999999990727 ) ) ;
#57470=CARTESIAN_POINT ( 'NONE',  ( 1.101062715680663384, 3.976440521211707768, 5.768354895643406977 ) ) ;
#57482=DIRECTION ( 'NONE',  ( 0.000000000000000000, 0.000000000000000000, -1.000000000000000000 ) ) ;
#57527=DIRECTION ( 'NONE',  ( -1.000000000000000000, 0.000000000000000000, 0.000000000000000000 ) ) ;
#57528=AXIS2_PLACEMENT_3D ( 'NONE', #71983, #115410, #27013 ) ;
#57549=CIRCLE ( 'NONE', #97117, 2.999999999999999112 ) ;
#57572=CARTESIAN_POINT ( 'NONE',  ( 31.69163961620377634, 6.094999999999988205, -1.633150327867694651 ) ) ;
#57583=FILL_AREA_STYLE ('',( #33687 ) ) ;
#57592=( NAMED_UNIT ( * ) SI_UNIT ( $, .STERADIAN. ) SOLID_ANGLE_UNIT ( ) );
#57603=EDGE_CURVE ( 'NONE', #98296, #80652, #115483, .T. ) ;
#57606=SURFACE_STYLE_FILL_AREA ( #99637 ) ;
#57632=( GEOMETRIC_REPRESENTATION_CONTEXT ( 3 ) GLOBAL_UNCERTAINTY_ASSIGNED_CONTEXT ( ( #105383 ) ) GLOBAL_UNIT_ASSIGNED_CONTEXT ( ( #89244, #38434, #60949 ) ) REPRESENTATION_CONTEXT ( 'NONE', 'WORKASPACE' ) );
#57633=FACE_OUTER_BOUND ( 'NONE', #53802, .T. ) ;
#57707=CYLINDRICAL_SURFACE ( 'NONE', #13950, 2.552699999999959779 ) ;
#57724=AXIS2_PLACEMENT_3D ( 'NONE', #72070, #70643, #82920 ) ;
#57725=CARTESIAN_POINT ( 'NONE',  ( 26.40000000000000568, -16.48000000000005016, -12.70000000000045404 ) ) ;
#57731=EDGE_CURVE ( 'NONE', #40407, #58595, #55280, .T. ) ;
#57742=CARTESIAN_POINT ( 'NONE',  ( 2.524972949537106270, -4.461849672132299993, -4.461849672132299105 ) ) ;
#57754=PRESENTATION_STYLE_ASSIGNMENT (( #12771 ) ) ;
#57767=PRESENTATION_STYLE_ASSIGNMENT (( #4005 ) ) ;
#57778=CARTESIAN_POINT ( 'NONE',  ( 22.29123647476855652, -9.717572351234235426E-16, -7.934999999999990727 ) ) ;
#57783=ORIENTED_EDGE ( 'NONE', *, *, #121757, .F. ) ;
#57821=CARTESIAN_POINT ( 'NONE',  ( 13.41666666666666785, 5.278424836066147208, 3.047499999999990550 ) ) ;
#57822=CARTESIAN_POINT ( 'NONE',  ( 22.87456980810188867, 6.871911579029510442, -3.967499999999998916 ) ) ;
#57833=CARTESIAN_POINT ( 'NONE',  ( 128.8595569075059473, -47.26730531257628343, -36.54674188582578154 ) ) ;
#57851=STYLED_ITEM ( 'NONE', ( #121597 ), #139780 ) ;
#57873=ORIENTED_EDGE ( 'NONE', *, *, #46059, .F. ) ;
#57884=CARTESIAN_POINT ( 'NONE',  ( 23.69206980810188412, -7.934999999999990727, -2.126176841940955242 ) ) ;
#57909=SURFACE_STYLE_FILL_AREA ( #112957 ) ;
#57949=CARTESIAN_POINT ( 'NONE',  ( 14.48330628287044064, 6.094999999999991758, 1.633150327867686880 ) ) ;
#57958=CARTESIAN_POINT ( 'NONE',  ( 28.06706980810189123, 2.126176841940952134, -7.934999999999993392 ) ) ;
#57966=CIRCLE ( 'NONE', #28, 2.999999999999998224 ) ;
#57990=( LENGTH_UNIT ( ) NAMED_UNIT ( * ) SI_UNIT ( .MILLI., .METRE. ) );
#57998=EDGE_CURVE ( 'NONE', #98679, #31597, #92283, .T. ) ;
#58002=CARTESIAN_POINT ( 'NONE',  ( 19.66623647476855297, 7.934999999999990727, -1.457635852685135314E-15 ) ) ;
#58004=CARTESIAN_POINT ( 'NONE',  ( 1.874569808101886226, 6.871911579029510442, -3.967499999999998916 ) ) ;
#58018=ORIENTED_EDGE ( 'NONE', *, *, #116212, .T. ) ;
#58019=CARTESIAN_POINT ( 'NONE',  ( 25.39999999999999858, -7.600000000000061817, 33.92499999999998295 ) ) ;
#58034=CARTESIAN_POINT ( 'NONE',  ( 56.10188787153392553, -51.19676978474260665, 38.21513923099968935 ) ) ;
#58047=AXIS2_PLACEMENT_3D ( 'NONE', #113445, #135926, #45388 ) ;
#58049=EDGE_CURVE ( 'NONE', #121495, #65849, #131919, .T. ) ;
#58051=ORIENTED_EDGE ( 'NONE', *, *, #2449, .T. ) ;
#58052=CARTESIAN_POINT ( 'NONE',  ( 8.358306282870438864, -1.633150327867700202, 6.094999999999985540 ) ) ;
#58060=ORIENTED_EDGE ( 'NONE', *, *, #119046, .T. ) ;
#58083=FILL_AREA_STYLE_COLOUR ( '', #21187 ) ;
#58088=( GEOMETRIC_REPRESENTATION_CONTEXT ( 3 ) GLOBAL_UNCERTAINTY_ASSIGNED_CONTEXT ( ( #127136 ) ) GLOBAL_UNIT_ASSIGNED_CONTEXT ( ( #59065, #101079, #133732 ) ) REPRESENTATION_CONTEXT ( 'NONE', 'WORKASPACE' ) );
#58098=( GEOMETRIC_REPRESENTATION_CONTEXT ( 3 ) GLOBAL_UNCERTAINTY_ASSIGNED_CONTEXT ( ( #70990 ) ) GLOBAL_UNIT_ASSIGNED_CONTEXT ( ( #98940, #133740, #1043 ) ) REPRESENTATION_CONTEXT ( 'NONE', 'WORKASPACE' ) );
#58119=DIRECTION ( 'NONE',  ( -0.000000000000000000, 1.000000000000000000, 0.000000000000000000 ) ) ;
#58133=CARTESIAN_POINT ( 'NONE',  ( 23.69206980810188057, -7.934999999999991616, -2.126176841940955242 ) ) ;
#58134=CARTESIAN_POINT ( 'NONE',  ( -0.5162635252314473622, -5.808823158059035485, -5.808823158059033709 ) ) ;
#58139=FILL_AREA_STYLE_COLOUR ( '', #7139 ) ;
#58145=CARTESIAN_POINT ( 'NONE',  ( 28.00000000000002487, -49.14999999999999147, -34.92499999999976978 ) ) ;
#58151=CARTESIAN_POINT ( 'NONE',  ( 55.56056557994608625, -52.00875322212550600, 39.86617647058822200 ) ) ;
#58179=( NAMED_UNIT ( * ) SI_UNIT ( $, .STERADIAN. ) SOLID_ANGLE_UNIT ( ) );
#58223=CARTESIAN_POINT ( 'NONE',  ( 152.4000000000000057, 7.919999999999947526, -18.97500000000001918 ) ) ;
#58263=AXIS2_PLACEMENT_3D ( 'NONE', #94567, #93863, #38783 ) ;
#58286=ORIENTED_EDGE ( 'NONE', *, *, #38752, .T. ) ;
#58296=CIRCLE ( 'NONE', #88258, 9.000000000000001776 ) ;
#58318=DIRECTION ( 'NONE',  ( -1.000000000000000000, 0.000000000000000000, 0.000000000000000000 ) ) ;
#58319=CARTESIAN_POINT ( 'NONE',  ( -0.5162635252314473622, -5.808823158059035485, -5.808823158059033709 ) ) ;
#58351=FILL_AREA_STYLE ('',( #134441 ) ) ;
#58354=( LENGTH_UNIT ( ) NAMED_UNIT ( * ) SI_UNIT ( .MILLI., .METRE. ) );
#58371=LINE ( 'NONE', #132340, #7063 ) ;
#58412=ORIENTED_EDGE ( 'NONE', *, *, #130295, .T. ) ;
#58418=CARTESIAN_POINT ( 'NONE',  ( 25.39999999999999858, 0.000000000000000000, 0.000000000000000000 ) ) ;
#58448=CARTESIAN_POINT ( 'NONE',  ( 184.1500000000000057, 26.96999999999993847, 34.92499999999998295 ) ) ;
#58457=LINE ( 'NONE', #136663, #113691 ) ;
#58473=FACE_OUTER_BOUND ( 'NONE', #43587, .T. ) ;
#58490=CARTESIAN_POINT ( 'NONE',  ( 4.566639616203772789, 1.633150327867695095, 6.094999999999988205 ) ) ;
#58520=CARTESIAN_POINT ( 'NONE',  ( 26.52040314143521726, 7.934999999999989839, -2.126176841940961904 ) ) ;
#58567=CARTESIAN_POINT ( 'NONE',  ( 24.93750000000000000, -4.461849672132299105, 4.461849672132299993 ) ) ;
#58570=COLOUR_RGB ( '', 0.66274510, 0.83137255, 0.94901961) ;
#58579=MECHANICAL_DESIGN_GEOMETRIC_PRESENTATION_REPRESENTATION('',(#40037),#23628);
#58595=VERTEX_POINT ( 'NONE', #31578 ) ;
#58611=EDGE_CURVE ( 'NONE', #65308, #73841, #55375, .T. ) ;
#58626=CARTESIAN_POINT ( 'NONE',  ( 22.37956980810188767, 3.967499999999998916, 6.871911579029510442 ) ) ;
#58629=FILL_AREA_STYLE ('',( #123129 ) ) ;
#58648=VECTOR ( 'NONE', #1568, 1000.000000000000000 ) ;
#58650=ORIENTED_EDGE ( 'NONE', *, *, #58611, .T. ) ;
#58673=VECTOR ( 'NONE', #102311, 1000.000000000000000 ) ;
#58674=ORIENTED_EDGE ( 'NONE', *, *, #52687, .T. ) ;
#58695=CARTESIAN_POINT ( 'NONE',  ( 25.58790314143521982, 6.871911579029515771, 3.967499999999989146 ) ) ;
#58706=VERTEX_POINT ( 'NONE', #2473 ) ;
#58707=VECTOR ( 'NONE', #112120, 1000.000000000000000 ) ;
#58709=CARTESIAN_POINT ( 'NONE',  ( 28.00000000000002487, -49.14999999999999147, -62.92499999999978400 ) ) ;
#58725=PLANE ( 'NONE',  #104567 ) ;
#58733=( LENGTH_UNIT ( ) NAMED_UNIT ( * ) SI_UNIT ( .MILLI., .METRE. ) );
#58736=CARTESIAN_POINT ( 'NONE',  ( 24.04123647476855652, 0.000000000000000000, 7.934999999999990727 ) ) ;
#58766=CARTESIAN_POINT ( 'NONE',  ( 55.56056557994607914, -52.00875322212550600, 39.86617647058822200 ) ) ;
#58795=( NAMED_UNIT ( * ) PLANE_ANGLE_UNIT ( ) SI_UNIT ( $, .RADIAN. ) );
#58833=FILL_AREA_STYLE ('',( #14554 ) ) ;
#58835=EDGE_CURVE ( 'NONE', #120201, #24682, #139488, .T. ) ;
#58838=PRESENTATION_STYLE_ASSIGNMENT (( #126180 ) ) ;
#58863=CARTESIAN_POINT ( 'NONE',  ( 0.2129031414352194063, 3.967499999999992699, -6.871911579029513994 ) ) ;
#58867=B_SPLINE_CURVE_WITH_KNOTS ( 'NONE', 3,
 ( #47333, #90045, #134294, #135033, #34994, #79235, #71720, #35726, #79946, #36400, #115883, #77771, #121949, #61573 ),
 .UNSPECIFIED., .F., .F.,
 ( 4, 2, 2, 2, 2, 2, 4 ),
 ( 4.978884922136755915E-17, 0.001506230150421708188, 0.002259345225632537237, 0.003012460300843366502, 0.004518690451265024166, 0.005271805526475853432, 0.006024920601686684432 ),
 .UNSPECIFIED. ) ;
#58869=CYLINDRICAL_SURFACE ( 'NONE', #210, 3.999999999999989786 ) ;
#58878=SURFACE_STYLE_USAGE ( .BOTH. , #4360 ) ;
#58879=( GEOMETRIC_REPRESENTATION_CONTEXT ( 3 ) GLOBAL_UNCERTAINTY_ASSIGNED_CONTEXT ( ( #137671 ) ) GLOBAL_UNIT_ASSIGNED_CONTEXT ( ( #108838, #34177, #133490 ) ) REPRESENTATION_CONTEXT ( 'NONE', 'WORKASPACE' ) );
#58880=VERTEX_POINT ( 'NONE', #64032 ) ;
#58898=( NAMED_UNIT ( * ) PLANE_ANGLE_UNIT ( ) SI_UNIT ( $, .RADIAN. ) );
#58919=CARTESIAN_POINT ( 'NONE',  ( 0.9064515957856063011, -6.147188561885386981, -3.738859411846097824 ) ) ;
#58932=CARTESIAN_POINT ( 'NONE',  ( 0.5411153073439879391, 7.255925504780224244, -2.140831595022724798 ) ) ;
#58943=ORIENTED_EDGE ( 'NONE', *, *, #66058, .F. ) ;
#58997=EDGE_LOOP ( 'NONE', ( #15987, #131625, #128700, #45845 ) ) ;
#59005=ORIENTED_EDGE ( 'NONE', *, *, #3601, .F. ) ;
#59028=CARTESIAN_POINT ( 'NONE',  ( -0.8079301918981138808, -7.934999999999991616, -2.126176841940955242 ) ) ;
#59052=CARTESIAN_POINT ( 'NONE',  ( 7.191639616203771901, 6.094999999999988205, -1.633150327867694651 ) ) ;
#59059=CARTESIAN_POINT ( 'NONE',  ( 2.457903141435219485, 6.871911579029515771, 3.967499999999989146 ) ) ;
#59065=( LENGTH_UNIT ( ) NAMED_UNIT ( * ) SI_UNIT ( .MILLI., .METRE. ) );
#59081=CARTESIAN_POINT ( 'NONE',  ( 11.66666666666666785, -5.278424836066145431, -3.047499999999993658 ) ) ;
#59085=UNCERTAINTY_MEASURE_WITH_UNIT (LENGTH_MEASURE( 1.000000000000000082E-05 ), #8518, 'distance_accuracy_value', 'NONE');
#59109=EDGE_LOOP ( 'NONE', ( #69275, #136183 ) ) ;
#59122=PRESENTATION_STYLE_ASSIGNMENT (( #101861 ) ) ;
#59151=( NAMED_UNIT ( * ) SI_UNIT ( $, .STERADIAN. ) SOLID_ANGLE_UNIT ( ) );
#59167=FILL_AREA_STYLE ('',( #24352 ) ) ;
#59182=CARTESIAN_POINT ( 'NONE',  ( 10.10830628287043709, 1.633150327867687324, -6.094999999999991758 ) ) ;
#59189=FILL_AREA_STYLE_COLOUR ( '', #74270 ) ;
#59204=PRESENTATION_STYLE_ASSIGNMENT (( #14928 ) ) ;
#59214=CARTESIAN_POINT ( 'NONE',  ( 21.41623647476855652, -7.934999999999990727, 4.858786175617117713E-16 ) ) ;
#59226=UNCERTAINTY_MEASURE_WITH_UNIT (LENGTH_MEASURE( 1.000000000000000082E-05 ), #90075, 'distance_accuracy_value', 'NONE');
#59249=SURFACE_SIDE_STYLE ('',( #3369 ) ) ;
#59261=CARTESIAN_POINT ( 'NONE',  ( 22.89583333333333215, 1.633150327867687324, -6.094999999999991758 ) ) ;
#59270=DIRECTION ( 'NONE',  ( -1.000000000000000000, -0.000000000000000000, -0.000000000000000000 ) ) ;
#59272=CARTESIAN_POINT ( 'NONE',  ( 126.2468580783230578, -45.52550609312092433, -35.40428284070834053 ) ) ;
#59274=CARTESIAN_POINT ( 'NONE',  ( 27.99999999999999645, -49.14999999999999147, -49.92499999999968452 ) ) ;
#59295=CARTESIAN_POINT ( 'NONE',  ( 24.39999999999999858, 1.399999999999987699, -20.40202195861970580 ) ) ;
#59312=FILL_AREA_STYLE ('',( #102797 ) ) ;
#59313=CARTESIAN_POINT ( 'NONE',  ( 21.94206980810188057, 7.934999999999992504, 2.126176841940951689 ) ) ;
#59316=CARTESIAN_POINT ( 'NONE',  ( 3.062159117892274018, -48.47815212813052455, -38.14157743968407033 ) ) ;
#59323=EDGE_LOOP ( 'NONE', ( #77161, #132965 ) ) ;
#59325=CARTESIAN_POINT ( 'NONE',  ( 9.333333333333333925, 5.278424836066143655, -3.047499999999997655 ) ) ;
#59338=VERTEX_POINT ( 'NONE', #141420 ) ;
#59378=CARTESIAN_POINT ( 'NONE',  ( 32.58790314143522693, 6.871911579029515771, 3.967499999999989146 ) ) ;
#59389=SURFACE_STYLE_FILL_AREA ( #16540 ) ;
#59403=CARTESIAN_POINT ( 'NONE',  ( 59.70964273381705567, -44.90675832754596541, -35.11767176073973218 ) ) ;
#59413=UNCERTAINTY_MEASURE_WITH_UNIT (LENGTH_MEASURE( 1.000000000000000082E-05 ), #120046, 'distance_accuracy_value', 'NONE');
#59414=ORIENTED_EDGE ( 'NONE', *, *, #116171, .T. ) ;
#59425=CARTESIAN_POINT ( 'NONE',  ( 30.89540314143522437, 2.126176841940962348, 7.934999999999989839 ) ) ;
#59438=CARTESIAN_POINT ( 'NONE',  ( 23.96247294953710849, -7.464222240803106570E-16, -6.094999999999989981 ) ) ;
#59445=CARTESIAN_POINT ( 'NONE',  ( 25.39999999999999858, 0.000000000000000000, 6.094999999999989093 ) ) ;
#59461=CARTESIAN_POINT ( 'NONE',  ( 0.000000000000000000, -30.18000000000009564, 12.69999999999954454 ) ) ;
#59471=FILL_AREA_STYLE_COLOUR ( '', #35335 ) ;
#59478=CARTESIAN_POINT ( 'NONE',  ( 0.7962364747685526378, 7.934999999999990727, -1.457635852685135314E-15 ) ) ;
#59480=FILL_AREA_STYLE ('',( #70378 ) ) ;
#59516=FILL_AREA_STYLE ('',( #80550 ) ) ;
#59527=ORIENTED_EDGE ( 'NONE', *, *, #57998, .F. ) ;
#59558=VERTEX_POINT ( 'NONE', #58019 ) ;
#59586=DIRECTION ( 'NONE',  ( 0.000000000000000000, -1.000000000000000000, 0.000000000000000000 ) ) ;
#59622=DIRECTION ( 'NONE',  ( 0.000000000000000000, -1.000000000000000000, 5.075120898959324592E-15 ) ) ;
#59679=ORIENTED_EDGE ( 'NONE', *, *, #122379, .T. ) ;
#59696=CARTESIAN_POINT ( 'NONE',  ( 156.1500000000000057, -49.14999999999999147, 53.92499999999997584 ) ) ;
#59711=CARTESIAN_POINT ( 'NONE',  ( 4.733736474768551972, 5.808823158059036373, 5.808823158059032821 ) ) ;
#59736=CARTESIAN_POINT ( 'NONE',  ( 7.774972949537104938, 4.461849672132300881, 4.461849672132299105 ) ) ;
#59740=ORIENTED_EDGE ( 'NONE', *, *, #46059, .T. ) ;
#59741=ORIENTED_EDGE ( 'NONE', *, *, #35081, .F. ) ;
#59742=CIRCLE ( 'NONE', #126852, 5.999999999999998224 ) ;
#59746=CARTESIAN_POINT ( 'NONE',  ( 9.312069808101886892, 7.934999999999993392, 2.126176841940951689 ) ) ;
#59749=CARTESIAN_POINT ( 'NONE',  ( 184.1499999999998067, -49.85820393249939286, 34.92500000000001847 ) ) ;
#59794=( LENGTH_UNIT ( ) NAMED_UNIT ( * ) SI_UNIT ( .MILLI., .METRE. ) );
#59802=DIRECTION ( 'NONE',  ( 0.000000000000000000, 0.000000000000000000, 1.000000000000000000 ) ) ;
#59811=CARTESIAN_POINT ( 'NONE',  ( 61.46640106136302961, -49.14999999999999147, -40.92499999999998295 ) ) ;
#59826=DIRECTION ( 'NONE',  ( 0.000000000000000000, -1.000000000000000000, 0.000000000000000000 ) ) ;
#59827=VECTOR ( 'NONE', #49960, 1000.000000000000000 ) ;
#59864=CARTESIAN_POINT ( 'NONE',  ( 13.75413961620377457, 3.047499999999993214, -5.278424836066146320 ) ) ;
#59903=CARTESIAN_POINT ( 'NONE',  ( 19.08290314143522437, 3.967499999999992699, -6.871911579029513994 ) ) ;
#59916=STYLED_ITEM ( 'NONE', ( #6758 ), #36322 ) ;
#59949=FACE_OUTER_BOUND ( 'NONE', #119880, .T. ) ;
#59954=CARTESIAN_POINT ( 'NONE',  ( 23.33333333333333570, 5.278424836066143655, -3.047499999999997655 ) ) ;
#59973=PRESENTATION_STYLE_ASSIGNMENT (( #104885 ) ) ;
#59980=FILL_AREA_STYLE ('',( #105585 ) ) ;
#59994=CARTESIAN_POINT ( 'NONE',  ( 52.51203195997703688, -49.11957940092398900, -40.22172306649560625 ) ) ;
#60012=VERTEX_POINT ( 'NONE', #2466 ) ;
#60071=VERTEX_POINT ( 'NONE', #55467 ) ;
#60076=CARTESIAN_POINT ( 'NONE',  ( 29.52540314143522338, 2.126176841940962348, 7.934999999999989839 ) ) ;
#60106=EDGE_CURVE ( 'NONE', #23830, #59558, #41803, .T. ) ;
#60111=DIRECTION ( 'NONE',  ( 0.000000000000000000, 0.000000000000000000, -1.000000000000000000 ) ) ;
#60124=CARTESIAN_POINT ( 'NONE',  ( 31.33290314143522082, -3.967499999999994476, 6.871911579029513106 ) ) ;
#60125=CARTESIAN_POINT ( 'NONE',  ( 3.332903141435219929, -3.967499999999994476, 6.871911579029513106 ) ) ;
#60127=LINE ( 'NONE', #93451, #59827 ) ;
#60137=( LENGTH_UNIT ( ) NAMED_UNIT ( * ) SI_UNIT ( .MILLI., .METRE. ) );
#60180=CARTESIAN_POINT ( 'NONE',  ( 7.796236474768553748, 7.934999999999990727, -1.457635852685135314E-15 ) ) ;
#60181=CARTESIAN_POINT ( 'NONE',  ( 21.00000000000000000, 0.000000000000000000, 6.094999999999989981 ) ) ;
#60183=EDGE_CURVE ( 'NONE', #134905, #119311, #139862, .T. ) ;
#60194=CARTESIAN_POINT ( 'NONE',  ( 6.562500000000000888, 4.461849672132300881, 4.461849672132299105 ) ) ;
#60207=( LENGTH_UNIT ( ) NAMED_UNIT ( * ) SI_UNIT ( .MILLI., .METRE. ) );
#60223=( NAMED_UNIT ( * ) PLANE_ANGLE_UNIT ( ) SI_UNIT ( $, .RADIAN. ) );
#60236=EDGE_LOOP ( 'NONE', ( #56273, #67738, #79722, #116225 ) ) ;
#60253=CARTESIAN_POINT ( 'NONE',  ( 33.02540314143521272, 2.126176841940962348, 7.934999999999989839 ) ) ;
#60254=CARTESIAN_POINT ( 'NONE',  ( -1.537096858564780844, -3.967499999999994476, 6.871911579029513106 ) ) ;
#60259=LINE ( 'NONE', #39943, #7266 ) ;
#60261=EDGE_LOOP ( 'NONE', ( #59527, #44833, #39328, #93085 ) ) ;
#60269=EDGE_CURVE ( 'NONE', #104004, #71281, #92689, .T. ) ;
#60278=AXIS2_PLACEMENT_3D ( 'NONE', #54705, #126693, #43114 ) ;
#60306=COLOUR_RGB ( '', 0.31764706, 0.68627451, 0.89019608) ;
#60342=( NAMED_UNIT ( * ) PLANE_ANGLE_UNIT ( ) SI_UNIT ( $, .RADIAN. ) );
#60361=MECHANICAL_DESIGN_GEOMETRIC_PRESENTATION_REPRESENTATION('',(#41807),#141342);
#60405=( GEOMETRIC_REPRESENTATION_CONTEXT ( 3 ) GLOBAL_UNCERTAINTY_ASSIGNED_CONTEXT ( ( #47637 ) ) GLOBAL_UNIT_ASSIGNED_CONTEXT ( ( #86232, #108641, #31836 ) ) REPRESENTATION_CONTEXT ( 'NONE', 'WORKASPACE' ) );
#60432=CARTESIAN_POINT ( 'NONE',  ( 9.546236474768553748, -7.934999999999990727, 4.858786175617117713E-16 ) ) ;
#60443=CARTESIAN_POINT ( 'NONE',  ( 10.98330628287044064, 6.094999999999991758, 1.633150327867686880 ) ) ;
#60457=CIRCLE ( 'NONE', #34991, 3.999999999999989786 ) ;
#60467=CARTESIAN_POINT ( 'NONE',  ( 0.5620698081018862258, -7.934999999999991616, -2.126176841940955242 ) ) ;
#60485=CARTESIAN_POINT ( 'NONE',  ( 156.1499999999997783, -49.14999999999999147, 34.92500000000004690 ) ) ;
#60498=UNCERTAINTY_MEASURE_WITH_UNIT (LENGTH_MEASURE( 1.000000000000000082E-05 ), #69301, 'distance_accuracy_value', 'NONE');
#60551=ORIENTED_EDGE ( 'NONE', *, *, #7015, .T. ) ;
#60555=EDGE_LOOP ( 'NONE', ( #135250, #116194, #19154, #40750 ) ) ;
#60563=DIRECTION ( 'NONE',  ( 0.000000000000000000, 0.000000000000000000, 1.000000000000000000 ) ) ;
#60565=EDGE_CURVE ( 'NONE', #46809, #119897, #2547, .T. ) ;
#60580=VERTEX_POINT ( 'NONE', #79934 ) ;
#60610=CARTESIAN_POINT ( 'NONE',  ( 18.71247294953710494, 0.000000000000000000, 6.094999999999989981 ) ) ;
#60649=CARTESIAN_POINT ( 'NONE',  ( 28.41623647476855652, -7.934999999999990727, 4.858786175617117713E-16 ) ) ;
#60662=CARTESIAN_POINT ( 'NONE',  ( 0.4397996348738452688, -49.08473565290605478, -39.91868829876771230 ) ) ;
#60696=CARTESIAN_POINT ( 'NONE',  ( 23.04166666666666785, 3.047499999999993214, -5.278424836066146320 ) ) ;
#60698=( NAMED_UNIT ( * ) SI_UNIT ( $, .STERADIAN. ) SOLID_ANGLE_UNIT ( ) );
#60728=LINE ( 'NONE', #17182, #122075 ) ;
#60730=ORIENTED_EDGE ( 'NONE', *, *, #24011, .F. ) ;
#60754=CARTESIAN_POINT ( 'NONE',  ( 25.39999999999999858, -5.131256043349313067, -6.052638797879072108 ) ) ;
#60781=EDGE_LOOP ( 'NONE', ( #111951, #105874, #17577, #8371, #62748 ) ) ;
#60799=CARTESIAN_POINT ( 'NONE',  ( 131.7507865773015112, -49.14999999999999147, 40.57473644908944976 ) ) ;
#60817=CARTESIAN_POINT ( 'NONE',  ( 28.50456980810189123, 6.871911579029510442, -3.967499999999998916 ) ) ;
#60847=CARTESIAN_POINT ( 'NONE',  ( 55.86145213702158685, -48.75494892434144845, -38.51155878621100470 ) ) ;
#60864=CARTESIAN_POINT ( 'NONE',  ( 25.79123647476855652, -9.717572351234235426E-16, -7.934999999999990727 ) ) ;
#60865=CARTESIAN_POINT ( 'NONE',  ( 6.103736474768552078, 5.808823158059035485, 5.808823158059032821 ) ) ;
#60880=CARTESIAN_POINT ( 'NONE',  ( 23.52497294953710849, -4.461849672132299993, -4.461849672132299105 ) ) ;
#60881=COLOUR_RGB ( '', 0.31764706, 0.68627451, 0.89019608) ;
#60882=COLOUR_RGB ( '', 0.09019608, 0.27058824, 0.51372549) ;
#60890=FILL_AREA_STYLE ('',( #115897 ) ) ;
#60894=( LENGTH_UNIT ( ) NAMED_UNIT ( * ) SI_UNIT ( .MILLI., .METRE. ) );
#60900=EDGE_CURVE ( 'NONE', #137014, #129906, #60457, .T. ) ;
#60925=CARTESIAN_POINT ( 'NONE',  ( 5.608736474768551972, -5.808823158059033709, 5.808823158059035485 ) ) ;
#60949=( NAMED_UNIT ( * ) SI_UNIT ( $, .STERADIAN. ) SOLID_ANGLE_UNIT ( ) );
#60962=ORIENTED_EDGE ( 'NONE', *, *, #53900, .T. ) ;
#60972=CARTESIAN_POINT ( 'NONE',  ( 0.000000000000000000, -57.15000000000009095, 34.92499999999998295 ) ) ;
#60976=AXIS2_PLACEMENT_3D ( 'NONE', #124251, #14044, #91626 ) ;
#60994=CARTESIAN_POINT ( 'NONE',  ( 32.44206980810188412, 7.934999999999993392, 2.126176841940951689 ) ) ;
#60996=CARTESIAN_POINT ( 'NONE',  ( 1.962903141435219601, -3.967499999999994476, 6.871911579029513106 ) ) ;
#61009=SURFACE_STYLE_USAGE ( .BOTH. , #80586 ) ;
#61011=( LENGTH_UNIT ( ) NAMED_UNIT ( * ) SI_UNIT ( .MILLI., .METRE. ) );
#61046=ORIENTED_EDGE ( 'NONE', *, *, #65246, .T. ) ;
#61143=ORIENTED_EDGE ( 'NONE', *, *, #15645, .T. ) ;
#61160=CARTESIAN_POINT ( 'NONE',  ( 9.962472949537104938, -7.464222240803106570E-16, -6.094999999999989981 ) ) ;
#61172=CARTESIAN_POINT ( 'NONE',  ( 12.31706980810188412, -2.126176841940956130, 7.934999999999991616 ) ) ;
#61198=( NAMED_UNIT ( * ) PLANE_ANGLE_UNIT ( ) SI_UNIT ( $, .RADIAN. ) );
#61207=CARTESIAN_POINT ( 'NONE',  ( 6.103736474768552078, 5.808823158059036373, 5.808823158059032821 ) ) ;
#61213=VERTEX_POINT ( 'NONE', #54958 ) ;
#61220=CARTESIAN_POINT ( 'NONE',  ( 184.0791405606630917, -51.15040958483975686, -36.98623100868703517 ) ) ;
#61294=ORIENTED_EDGE ( 'NONE', *, *, #2035, .T. ) ;
#61305=ADVANCED_FACE ( 'NONE', ( #109316 ), #9238, .F. ) ;
#61307=AXIS2_PLACEMENT_3D ( 'NONE', #77226, #3185, #102535 ) ;
#61317=CARTESIAN_POINT ( 'NONE',  ( 181.1500000000000057, -43.14999999999999147, -34.92499999999998295 ) ) ;
#61333=CARTESIAN_POINT ( 'NONE',  ( 13.31663961620377279, -1.633150327867691987, -6.094999999999989093 ) ) ;
#61367=CARTESIAN_POINT ( 'NONE',  ( 31.18706980810189222, -2.126176841940956130, 7.934999999999991616 ) ) ;
#61371=ORIENTED_EDGE ( 'NONE', *, *, #138395, .F. ) ;
#61372=MECHANICAL_DESIGN_GEOMETRIC_PRESENTATION_REPRESENTATION('',(#21987),#3447);
#61381=CARTESIAN_POINT ( 'NONE',  ( 1.301042606982605163E-14, -47.62213595499957819, -36.92499999999998295 ) ) ;
#61410=AXIS2_PLACEMENT_3D ( 'NONE', #101524, #46497, #132776 ) ;
#61413=CARTESIAN_POINT ( 'NONE',  ( 22.60416666666666430, -1.633150327867691987, -6.094999999999989093 ) ) ;
#61426=VERTEX_POINT ( 'NONE', #93981 ) ;
#61433=CARTESIAN_POINT ( 'NONE',  ( 14.00000000000000178, 0.000000000000000000, 6.094999999999989981 ) ) ;
#61435=CARTESIAN_POINT ( 'NONE',  ( 1.547775330865844623, -2.540876819987784252, 6.037041738182785444 ) ) ;
#61446=ORIENTED_EDGE ( 'NONE', *, *, #12704, .T. ) ;
#61461=DIRECTION ( 'NONE',  ( -0.9707728879609257566, 0.000000000000000000, -0.2400000000000086786 ) ) ;
#61475=FILL_AREA_STYLE ('',( #104187 ) ) ;
#61507=PRESENTATION_STYLE_ASSIGNMENT (( #4156 ) ) ;
#61519=CARTESIAN_POINT ( 'NONE',  ( 0.1679803408748695992, -48.55783623716597219, 38.28685941347700350 ) ) ;
#61523=CARTESIAN_POINT ( 'NONE',  ( 1.874569808101886226, 6.871911579029510442, -3.967499999999998916 ) ) ;
#61528=EDGE_LOOP ( 'NONE', ( #95991, #44155, #81219, #142636 ) ) ;
#61547=CARTESIAN_POINT ( 'NONE',  ( 55.49226980200836579, -49.12413125935074731, -39.93743342457434409 ) ) ;
#61565=CARTESIAN_POINT ( 'NONE',  ( 27.97873647476855297, -5.808823158059033709, 5.808823158059035485 ) ) ;
#61566=CARTESIAN_POINT ( 'NONE',  ( 7.999569808101885116, -3.967499999999998028, -6.871911579029511330 ) ) ;
#61573=CARTESIAN_POINT ( 'NONE',  ( 25.39999999999999503, 3.246059068589359775, 5.158694168414005077 ) ) ;
#61588=CARTESIAN_POINT ( 'NONE',  ( 152.4000000000000057, -14.29000000000013593, -12.70000000000045404 ) ) ;
#61591=CARTESIAN_POINT ( 'NONE',  ( 57.90314192168177954, -45.52550609312090302, 35.40428284070832632 ) ) ;
#61621=CARTESIAN_POINT ( 'NONE',  ( 9.837903141435219823, -6.871911579029513106, -3.967499999999993587 ) ) ;
#61648=ORIENTED_EDGE ( 'NONE', *, *, #113154, .F. ) ;
#61670=ORIENTED_EDGE ( 'NONE', *, *, #122692, .T. ) ;
#61683=CARTESIAN_POINT ( 'NONE',  ( 6.629569808101885897, -3.967499999999998028, -6.871911579029511330 ) ) ;
#61730=ORIENTED_EDGE ( 'NONE', *, *, #132268, .F. ) ;
#61767=SURFACE_STYLE_FILL_AREA ( #126288 ) ;
#61825=CARTESIAN_POINT ( 'NONE',  ( 151.4000000000000057, -18.48000000000005372, -34.92499999999998295 ) ) ;
#61851=CARTESIAN_POINT ( 'NONE',  ( 9.254569808101885897, -6.871911579029512218, 3.967499999999996252 ) ) ;
#61887=CARTESIAN_POINT ( 'NONE',  ( 2.166236474768552966, 7.934999999999990727, -1.457635852685135314E-15 ) ) ;
#61907=DIRECTION ( 'NONE',  ( 0.000000000000000000, 0.000000000000000000, -1.000000000000000000 ) ) ;
#61913=CARTESIAN_POINT ( 'NONE',  ( 10.64583333333333393, -1.633150327867700202, 6.094999999999985540 ) ) ;
#61954=DIRECTION ( 'NONE',  ( 0.2400000000000085398, -0.000000000000000000, 0.9707728879609256456 ) ) ;
#61985=EDGE_LOOP ( 'NONE', ( #52258, #52379 ) ) ;
#62021=CARTESIAN_POINT ( 'NONE',  ( 11.42080628287044064, 3.047499999999997655, 5.278424836066143655 ) ) ;
#62041=VERTEX_POINT ( 'NONE', #121797 ) ;
#62052=VERTEX_POINT ( 'NONE', #34116 ) ;
#62068=CARTESIAN_POINT ( 'NONE',  ( 0.1679803408763183847, -48.55783623716211395, -38.28685941347502819 ) ) ;
#62097=CARTESIAN_POINT ( 'NONE',  ( 25.39999999999999858, -16.48000000000005016, 33.92499999999998295 ) ) ;
#62099=CARTESIAN_POINT ( 'NONE',  ( 30.04166666666666785, 3.047499999999993214, -5.278424836066146320 ) ) ;
#62109=DIRECTION ( 'NONE',  ( 0.000000000000000000, 0.000000000000000000, 1.000000000000000000 ) ) ;
#62117=DIRECTION ( 'NONE',  ( -1.000000000000000000, -0.000000000000000000, -0.000000000000000000 ) ) ;
#62123=LINE ( 'NONE', #104148, #68301 ) ;
#62131=STYLED_ITEM ( 'NONE', ( #123598 ), #38134 ) ;
#62145=LINE ( 'NONE', #117892, #86054 ) ;
#62156=VERTEX_POINT ( 'NONE', #115904 ) ;
#62159=ORIENTED_EDGE ( 'NONE', *, *, #90529, .F. ) ;
#62206=ADVANCED_FACE ( 'NONE', ( #15175 ), #127236, .T. ) ;
#62213=CARTESIAN_POINT ( 'NONE',  ( 0.01167931549069121423, -50.55966373066888053, 35.89041033429500516 ) ) ;
#62216=CARTESIAN_POINT ( 'NONE',  ( 1.437069808101885782, 2.126176841940952134, -7.934999999999993392 ) ) ;
#62246=ORIENTED_EDGE ( 'NONE', *, *, #132268, .T. ) ;
#62257=CARTESIAN_POINT ( 'NONE',  ( 4.229166666666666963, -6.094999999999989093, 1.633150327867691765 ) ) ;
#62258=CARTESIAN_POINT ( 'NONE',  ( 5.520403141435219929, 7.934999999999988951, -2.126176841940961904 ) ) ;
#62278=AXIS2_PLACEMENT_3D ( 'NONE', #1480, #66082, #110248 ) ;
#62282=CARTESIAN_POINT ( 'NONE',  ( 0.2153679725188470950, -51.67626207039724306, 38.40320453011149482 ) ) ;
#62321=CARTESIAN_POINT ( 'NONE',  ( 10.27540314143522160, -2.126176841940958351, -7.934999999999988951 ) ) ;
#62327=EDGE_CURVE ( 'NONE', #52815, #78350, #33260, .T. ) ;
#62330=CARTESIAN_POINT ( 'NONE',  ( 0.000000000000000000, -7.600000000000055600, -28.92499999999998650 ) ) ;
#62337=CARTESIAN_POINT ( 'NONE',  ( 17.93750000000000355, -4.461849672132299105, 4.461849672132299993 ) ) ;
#62357=ORIENTED_EDGE ( 'NONE', *, *, #121722, .T. ) ;
#62371=AXIS2_PLACEMENT_3D ( 'NONE', #77655, #76212, #31291 ) ;
#62390=CARTESIAN_POINT ( 'NONE',  ( 6.046236474768552860, -7.934999999999990727, 4.858786175617117713E-16 ) ) ;
#62402=DIRECTION ( 'NONE',  ( -1.000000000000000000, -0.000000000000000000, -0.000000000000000000 ) ) ;
#62406=CARTESIAN_POINT ( 'NONE',  ( 2.999999999999999112, -7.600000000000053824, -34.92499999999998295 ) ) ;
#62421=AXIS2_PLACEMENT_3D ( 'NONE', #58223, #68372, #112551 ) ;
#62458=FACE_OUTER_BOUND ( 'NONE', #875, .T. ) ;
#62510=ORIENTED_EDGE ( 'NONE', *, *, #48583, .T. ) ;
#62521=CARTESIAN_POINT ( 'NONE',  ( 3.102554694470387897, -48.63825160239814949, 38.47250499286694492 ) ) ;
#62528=EDGE_CURVE ( 'NONE', #130484, #18319, #30920, .T. ) ;
#62531=ORIENTED_EDGE ( 'NONE', *, *, #74448, .T. ) ;
#62552=CARTESIAN_POINT ( 'NONE',  ( 159.7320121765528711, 26.96999999999993847, -34.92499999999998295 ) ) ;
#62556=CARTESIAN_POINT ( 'NONE',  ( 14.06706980810188412, 2.126176841940952134, -7.934999999999993392 ) ) ;
#62565=CARTESIAN_POINT ( 'NONE',  ( 11.71247294953710671, 0.000000000000000000, 6.094999999999989981 ) ) ;
#62589=CARTESIAN_POINT ( 'NONE',  ( 14.41623647476855297, -7.934999999999990727, 4.858786175617117713E-16 ) ) ;
#62596=CARTESIAN_POINT ( 'NONE',  ( 5.004139616203772789, -3.047499999999994547, 5.278424836066145431 ) ) ;
#62598=DIRECTION ( 'NONE',  ( 0.000000000000000000, -5.075120898959323014E-15, -1.000000000000000000 ) ) ;
#62614=CARTESIAN_POINT ( 'NONE',  ( 156.1500000000000057, -49.14999999999999147, -53.92499999999968452 ) ) ;
#62619=ORIENTED_EDGE ( 'NONE', *, *, #2753, .T. ) ;
#62638=ADVANCED_FACE ( 'NONE', ( #6955 ), #67813, .T. ) ;
#62641=VERTEX_POINT ( 'NONE', #19310 ) ;
#62658=AXIS2_PLACEMENT_3D ( 'NONE', #110840, #34055, #131937 ) ;
#62731=ORIENTED_EDGE ( 'NONE', *, *, #111556, .T. ) ;
#62735=CARTESIAN_POINT ( 'NONE',  ( 14.04580628287044064, 5.278424836066143655, -3.047499999999997655 ) ) ;
#62748=ORIENTED_EDGE ( 'NONE', *, *, #112443, .F. ) ;
#62763=CARTESIAN_POINT ( 'NONE',  ( 32.93706980810188156, 2.126176841940952134, -7.934999999999993392 ) ) ;
#62770=ADVANCED_FACE ( 'NONE', ( #111296 ), #53360, .F. ) ;
#62778=CARTESIAN_POINT ( 'NONE',  ( 3.298144211979623819, -48.98056306480231825, -39.49745726092410791 ) ) ;
#62805=EDGE_LOOP ( 'NONE', ( #130112, #132313, #98611, #31842, #106181 ) ) ;
#62837=CARTESIAN_POINT ( 'NONE',  ( 12.97916666666666607, 6.094999999999988205, -1.633150327867694651 ) ) ;
#62848=COLOUR_RGB ( '', 0.40784314, 0.44705882, 0.49803922) ;
#62871=SURFACE_SIDE_STYLE ('',( #8412 ) ) ;
#62873=( LENGTH_UNIT ( ) NAMED_UNIT ( * ) SI_UNIT ( .MILLI., .METRE. ) );
#62880=CARTESIAN_POINT ( 'NONE',  ( 184.0378153480267258, -51.37040454773216425, 37.49526731630399468 ) ) ;
#62881=AXIS2_PLACEMENT_3D ( 'NONE', #42622, #107819, #54911 ) ;
#62883=( NAMED_UNIT ( * ) SI_UNIT ( $, .STERADIAN. ) SOLID_ANGLE_UNIT ( ) );
#62884=VECTOR ( 'NONE', #121490, 1000.000000000000000 ) ;
#62896=VECTOR ( 'NONE', #29721, 1000.000000000000000 ) ;
#62935=CARTESIAN_POINT ( 'NONE',  ( 0.5414528859217531132, -52.10163751122425424, 40.43817685073605617 ) ) ;
#62939=CARTESIAN_POINT ( 'NONE',  ( 6.395403141435219929, 2.126176841940962348, 7.934999999999989839 ) ) ;
#62951=VECTOR ( 'NONE', #112846, 1000.000000000000000 ) ;
#62962=CIRCLE ( 'NONE', #88410, 28.00000000000001776 ) ;
#62967=CARTESIAN_POINT ( 'NONE',  ( 54.91896556007530705, -47.51495700085917662, -36.79359617903136126 ) ) ;
#62986=CARTESIAN_POINT ( 'NONE',  ( 1.166666666666666741, -5.278424836066145431, -3.047499999999993658 ) ) ;
#62987=CARTESIAN_POINT ( 'NONE',  ( 6.541236474768552966, 0.000000000000000000, 7.934999999999990727 ) ) ;
#62992=VERTEX_POINT ( 'NONE', #127923 ) ;
#62997=ORIENTED_EDGE ( 'NONE', *, *, #115028, .T. ) ;
#63018=CARTESIAN_POINT ( 'NONE',  ( 56.65265948608892188, -50.37061236291013699, 37.32649486623391510 ) ) ;
#63034=ADVANCED_FACE ( 'NONE', ( #54638 ), #143058, .T. ) ;
#63038=DIRECTION ( 'NONE',  ( 0.000000000000000000, 0.000000000000000000, -1.000000000000000000 ) ) ;
#63048=CARTESIAN_POINT ( 'NONE',  ( 13.48373647476855375, -5.808823158059035485, -5.808823158059033709 ) ) ;
#63068=SURFACE_STYLE_USAGE ( .BOTH. , #7185 ) ;
#63109=( NAMED_UNIT ( * ) PLANE_ANGLE_UNIT ( ) SI_UNIT ( $, .RADIAN. ) );
#63114=DIRECTION ( 'NONE',  ( -1.000000000000000000, -0.000000000000000000, 0.000000000000000000 ) ) ;
#63116=CARTESIAN_POINT ( 'NONE',  ( 11.00456980810188590, 6.871911579029510442, -3.967499999999998916 ) ) ;
#63150=ORIENTED_EDGE ( 'NONE', *, *, #62528, .F. ) ;
#63172=VERTEX_POINT ( 'NONE', #45218 ) ;
#63201=ORIENTED_EDGE ( 'NONE', *, *, #104302, .F. ) ;
#63234=DIRECTION ( 'NONE',  ( 0.000000000000000000, 0.000000000000000000, 1.000000000000000000 ) ) ;
#63258=CARTESIAN_POINT ( 'NONE',  ( 3.487905803711476072, -49.11927476322658492, 40.22110306067541075 ) ) ;
#63297=CARTESIAN_POINT ( 'NONE',  ( 22.52540314143522338, 2.126176841940962348, 7.934999999999989839 ) ) ;
#63320=CARTESIAN_POINT ( 'NONE',  ( 4.520833333333333037, -6.094999999999989981, -1.633150327867689322 ) ) ;
#63327=CARTESIAN_POINT ( 'NONE',  ( 13.10373647476855297, 5.808823158059036373, 5.808823158059032821 ) ) ;
#63361=DIRECTION ( 'NONE',  ( 0.000000000000000000, 1.000000000000000000, -5.782411586589357244E-15 ) ) ;
#63375=( GEOMETRIC_REPRESENTATION_CONTEXT ( 3 ) GLOBAL_UNCERTAINTY_ASSIGNED_CONTEXT ( ( #127485 ) ) GLOBAL_UNIT_ASSIGNED_CONTEXT ( ( #31779, #141991, #140521 ) ) REPRESENTATION_CONTEXT ( 'NONE', 'WORKASPACE' ) );
#63376=SURFACE_STYLE_USAGE ( .BOTH. , #114318 ) ;
#63378=LINE ( 'NONE', #120534, #14438 ) ;
#63387=SURFACE_STYLE_FILL_AREA ( #128607 ) ;
#63389=( NAMED_UNIT ( * ) SI_UNIT ( $, .STERADIAN. ) SOLID_ANGLE_UNIT ( ) );
#63396=CIRCLE ( 'NONE', #17000, 2.999999999999998224 ) ;
#63443=DIRECTION ( 'NONE',  ( 0.9843059135695010342, 0.000000000000000000, 0.1764705882352919641 ) ) ;
#63449=DIRECTION ( 'NONE',  ( -1.000000000000000000, -0.000000000000000000, -0.000000000000000000 ) ) ;
#63464=CARTESIAN_POINT ( 'NONE',  ( 25.27497294953710849, 4.461849672132300881, 4.461849672132299105 ) ) ;
#63475=EDGE_CURVE ( 'NONE', #32751, #105463, #54553, .T. ) ;
#63494=CARTESIAN_POINT ( 'NONE',  ( 29.72873647476855297, 5.808823158059031044, -5.808823158059038150 ) ) ;
#63563=CARTESIAN_POINT ( 'NONE',  ( 128.9683591370938416, -49.14999999999998437, -41.64500000000001023 ) ) ;
#63568=ORIENTED_EDGE ( 'NONE', *, *, #25823, .F. ) ;
#63583=AXIS2_PLACEMENT_3D ( 'NONE', #138118, #38806, #6833 ) ;
#63596=( NAMED_UNIT ( * ) PLANE_ANGLE_UNIT ( ) SI_UNIT ( $, .RADIAN. ) );
#63603=( NAMED_UNIT ( * ) PLANE_ANGLE_UNIT ( ) SI_UNIT ( $, .RADIAN. ) );
#63614=ORIENTED_EDGE ( 'NONE', *, *, #106320, .F. ) ;
#63629=CARTESIAN_POINT ( 'NONE',  ( -0.2458603837962275163, 3.047499999999993214, -5.278424836066146320 ) ) ;
#63650=CARTESIAN_POINT ( 'NONE',  ( 3.221442824812094763, -48.88296141031990061, 39.14553452061911543 ) ) ;
#63653=CARTESIAN_POINT ( 'NONE',  ( 8.437069808101885116, 2.126176841940952134, -7.934999999999993392 ) ) ;
#63679=CARTESIAN_POINT ( 'NONE',  ( 55.29044309249841405, -47.26730531257518919, -36.54674188582485783 ) ) ;
#63689=SURFACE_STYLE_USAGE ( .BOTH. , #106404 ) ;
#63696=CARTESIAN_POINT ( 'NONE',  ( 5.395833333333334814, 1.633150327867687324, -6.094999999999991758 ) ) ;
#63697=CARTESIAN_POINT ( 'NONE',  ( 19.95790314143522437, 6.871911579029515771, 3.967499999999989146 ) ) ;
#63709=ORIENTED_EDGE ( 'NONE', *, *, #128289, .T. ) ;
#63713=DIRECTION ( 'NONE',  ( 0.000000000000000000, 0.000000000000000000, 1.000000000000000000 ) ) ;
#63723=ADVANCED_FACE ( 'NONE', ( #84169 ), #88022, .T. ) ;
#63731=CARTESIAN_POINT ( 'NONE',  ( 124.0768256643112011, -45.23984008851422800, 35.04755940937925374 ) ) ;
#63765=( LENGTH_UNIT ( ) NAMED_UNIT ( * ) SI_UNIT ( .MILLI., .METRE. ) );
#63770=FILL_AREA_STYLE_COLOUR ( '', #55736 ) ;
#63788=( NAMED_UNIT ( * ) SI_UNIT ( $, .STERADIAN. ) SOLID_ANGLE_UNIT ( ) );
#63806=CARTESIAN_POINT ( 'NONE',  ( 26.40000000000000568, -17.48000000000005016, -33.92499999999998295 ) ) ;
#63807=PLANE ( 'NONE',  #17974 ) ;
#63815=CARTESIAN_POINT ( 'NONE',  ( 12.60873647476855197, -5.808823158059033709, 5.808823158059035485 ) ) ;
#63818=( GEOMETRIC_REPRESENTATION_CONTEXT ( 3 ) GLOBAL_UNCERTAINTY_ASSIGNED_CONTEXT ( ( #111257 ) ) GLOBAL_UNIT_ASSIGNED_CONTEXT ( ( #93309, #4814, #49115 ) ) REPRESENTATION_CONTEXT ( 'NONE', 'WORKASPACE' ) );
#63837=VERTEX_POINT ( 'NONE', #52213 ) ;
#63847=CARTESIAN_POINT ( 'NONE',  ( 153.4000000000000057, 26.96999999999993847, 34.92499999999998295 ) ) ;
#63850=UNCERTAINTY_MEASURE_WITH_UNIT (LENGTH_MEASURE( 1.000000000000000082E-05 ), #46762, 'distance_accuracy_value', 'NONE');
#63858=CARTESIAN_POINT ( 'NONE',  ( 0.1600000000000008915, -3.866712830111943333, -6.953158445676763222 ) ) ;
#63929=CIRCLE ( 'NONE', #50062, 5.999999999999998224 ) ;
#63954=SURFACE_STYLE_USAGE ( .BOTH. , #19712 ) ;
#63974=DIRECTION ( 'NONE',  ( -0.000000000000000000, 1.000000000000000000, 1.091707662666338270E-16 ) ) ;
#63977=CARTESIAN_POINT ( 'NONE',  ( 20.48373647476854842, -5.808823158059035485, -5.808823158059033709 ) ) ;
#64002=ORIENTED_EDGE ( 'NONE', *, *, #91353, .T. ) ;
#64004=DIRECTION ( 'NONE',  ( -1.000000000000000000, 0.000000000000000000, 0.000000000000000000 ) ) ;
#64010=CARTESIAN_POINT ( 'NONE',  ( 15.14540314143522082, -2.126176841940958351, -7.934999999999989839 ) ) ;
#64012=CARTESIAN_POINT ( 'NONE',  ( 184.1500000000000057, -43.14999999999999147, 31.92499999999998295 ) ) ;
#64032=CARTESIAN_POINT ( 'NONE',  ( 11.71247294953710671, 0.000000000000000000, 6.094999999999989981 ) ) ;
#64068=FILL_AREA_STYLE_COLOUR ( '', #30083 ) ;
#64075=CARTESIAN_POINT ( 'NONE',  ( 14.58333333333333570, -5.278424836066144543, 3.047499999999995879 ) ) ;
#64089=( NAMED_UNIT ( * ) SI_UNIT ( $, .STERADIAN. ) SOLID_ANGLE_UNIT ( ) );
#64094=CARTESIAN_POINT ( 'NONE',  ( 174.7500000000000000, 7.919999999999947526, -18.97500000000001918 ) ) ;
#64123=DIRECTION ( 'NONE',  ( 1.000000000000000000, 0.000000000000000000, 0.000000000000000000 ) ) ;
#64132=( NAMED_UNIT ( * ) SI_UNIT ( $, .STERADIAN. ) SOLID_ANGLE_UNIT ( ) );
#64149=COLOUR_RGB ( '', 0.09019608, 0.27058824, 0.51372549) ;
#64150=CARTESIAN_POINT ( 'NONE',  ( 21.92080628287044064, 3.047499999999997655, 5.278424836066143655 ) ) ;
#64216=ORIENTED_EDGE ( 'NONE', *, *, #114038, .F. ) ;
#64227=CARTESIAN_POINT ( 'NONE',  ( 29.45833333333333570, -3.047499999999997211, -5.278424836066143655 ) ) ;
#64248=VECTOR ( 'NONE', #57197, 1000.000000000000000 ) ;
#64289=ADVANCED_FACE ( 'NONE', ( #42627 ), #115810, .T. ) ;
#64299=ORIENTED_EDGE ( 'NONE', *, *, #140716, .F. ) ;
#64318=DIRECTION ( 'NONE',  ( 1.000000000000000000, 0.000000000000000000, 0.000000000000000000 ) ) ;
#64344=CARTESIAN_POINT ( 'NONE',  ( 4.062069808101884227, -7.934999999999991616, -2.126176841940955242 ) ) ;
#64352=SURFACE_SIDE_STYLE ('',( #53477 ) ) ;
#64384=CARTESIAN_POINT ( 'NONE',  ( 0.7291666666666667407, -6.094999999999989093, 1.633150327867691765 ) ) ;
#64385=CARTESIAN_POINT ( 'NONE',  ( 13.24956980810188689, 3.967499999999998916, 6.871911579029510442 ) ) ;
#64396=CARTESIAN_POINT ( 'NONE',  ( 129.9042113015468942, -47.96374157527412763, -37.32649486623387958 ) ) ;
#64403=CARTESIAN_POINT ( 'NONE',  ( 3.000000000000000000, -4.600000000000012079, -20.40202195861968093 ) ) ;
#64416=CARTESIAN_POINT ( 'NONE',  ( 126.2468580783130960, -45.52550609312172725, 35.40428284070863896 ) ) ;
#64420=CARTESIAN_POINT ( 'NONE',  ( 183.6042742895559741, -52.10338527932238151, 40.45859298138253735 ) ) ;
#64436=CARTESIAN_POINT ( 'NONE',  ( 15.37956980810188767, 3.967499999999998916, 6.871911579029510442 ) ) ;
#64447=ORIENTED_EDGE ( 'NONE', *, *, #52929, .T. ) ;
#64452=CARTESIAN_POINT ( 'NONE',  ( 18.81250000000000355, -4.461849672132299993, -4.461849672132299105 ) ) ;
#64500=CARTESIAN_POINT ( 'NONE',  ( 184.1500000000000057, 0.000000000000000000, 0.000000000000000000 ) ) ;
#64510=CARTESIAN_POINT ( 'NONE',  ( 6.192069808101887674, -7.934999999999991616, -2.126176841940955242 ) ) ;
#64549=CARTESIAN_POINT ( 'NONE',  ( 0.1600000000000008360, -6.382865826061452807, -4.762547549401616287 ) ) ;
#64552=CYLINDRICAL_SURFACE ( 'NONE', #143229, 1.000000000000000000 ) ;
#64563=CIRCLE ( 'NONE', #6656, 3.000000000000002220 ) ;
#64564=ORIENTED_EDGE ( 'NONE', *, *, #20578, .F. ) ;
#64597=AXIS2_PLACEMENT_3D ( 'NONE', #30095, #66326, #43850 ) ;
#64599=( NAMED_UNIT ( * ) SI_UNIT ( $, .STERADIAN. ) SOLID_ANGLE_UNIT ( ) );
#64612=ORIENTED_EDGE ( 'NONE', *, *, #74448, .F. ) ;
#64614=LINE ( 'NONE', #129874, #13727 ) ;
#64630=COLOUR_RGB ( '', 0.72549020, 0.75294118, 0.79215686) ;
#64635=EDGE_CURVE ( 'NONE', #66768, #137573, #85835, .T. ) ;
#64646=FILL_AREA_STYLE ('',( #128486 ) ) ;
#64657=FACE_OUTER_BOUND ( 'NONE', #22938, .T. ) ;
#64661=COLOUR_RGB ( '', 0.08235294, 0.09019608, 0.10196078) ;
#64664=MECHANICAL_DESIGN_GEOMETRIC_PRESENTATION_REPRESENTATION('',(#131834),#101705);
#64667=PLANE ( 'NONE',  #106111 ) ;
#64692=CARTESIAN_POINT ( 'NONE',  ( 14.65040314143522338, 7.934999999999989839, -2.126176841940961904 ) ) ;
#64698=STYLED_ITEM ( 'NONE', ( #31135 ), #21254 ) ;
#64706=VERTEX_POINT ( 'NONE', #65661 ) ;
#64728=CARTESIAN_POINT ( 'NONE',  ( 3.000000000000000000, -49.85820393249935734, -34.92499999999996874 ) ) ;
#64788=( GEOMETRIC_REPRESENTATION_CONTEXT ( 3 ) GLOBAL_UNCERTAINTY_ASSIGNED_CONTEXT ( ( #59085 ) ) GLOBAL_UNIT_ASSIGNED_CONTEXT ( ( #8518, #36739, #524 ) ) REPRESENTATION_CONTEXT ( 'NONE', 'WORKASPACE' ) );
#64791=CARTESIAN_POINT ( 'NONE',  ( 8.212472949537106715, 0.000000000000000000, 6.094999999999989981 ) ) ;
#64795=CARTESIAN_POINT ( 'NONE',  ( 14.00000000000000178, 0.000000000000000000, 6.094999999999989981 ) ) ;
#64805=DIRECTION ( 'NONE',  ( 0.000000000000000000, 0.000000000000000000, 1.000000000000000000 ) ) ;
#64815=EDGE_CURVE ( 'NONE', #66768, #86570, #26915, .T. ) ;
#64853=CARTESIAN_POINT ( 'NONE',  ( 25.39999999999999858, 0.000000000000000000, 0.000000000000000000 ) ) ;
#64869=CARTESIAN_POINT ( 'NONE',  ( 27.02497294953710494, -4.461849672132299993, -4.461849672132299105 ) ) ;
#64871=ORIENTED_EDGE ( 'NONE', *, *, #78263, .T. ) ;
#64905=TOROIDAL_SURFACE ( 'NONE', #118042, 2.000000000000000000, 1.000000000000000000 ) ;
#64917=CARTESIAN_POINT ( 'NONE',  ( 184.1500000000000057, -17.48000000000005016, -12.70000000000045404 ) ) ;
#64936=DIRECTION ( 'NONE',  ( 0.000000000000000000, -1.000000000000000000, 0.000000000000000000 ) ) ;
#64958=ADVANCED_FACE ( 'NONE', ( #129793 ), #109002, .F. ) ;
#64973=DIRECTION ( 'NONE',  ( 0.000000000000000000, 0.06845965770171358322, -0.9976538855070752332 ) ) ;
#64979=CIRCLE ( 'NONE', #2414, 3.000000000000002220 ) ;
#65004=EDGE_LOOP ( 'NONE', ( #89678, #22338, #70664, #140286, #46198, #4963, #142427, #136057, #38425, #71402 ) ) ;
#65005=ORIENTED_EDGE ( 'NONE', *, *, #56682, .T. ) ;
#65007=( GEOMETRIC_REPRESENTATION_CONTEXT ( 3 ) GLOBAL_UNCERTAINTY_ASSIGNED_CONTEXT ( ( #122867 ) ) GLOBAL_UNIT_ASSIGNED_CONTEXT ( ( #52406, #42278, #20477 ) ) REPRESENTATION_CONTEXT ( 'NONE', 'WORKASPACE' ) );
#65020=AXIS2_PLACEMENT_3D ( 'NONE', #20329, #97922, #65321 ) ;
#65028=CARTESIAN_POINT ( 'NONE',  ( 2.670806282870439308, -3.047499999999997211, -5.278424836066143655 ) ) ;
#65035=EDGE_CURVE ( 'NONE', #117767, #141737, #131229, .T. ) ;
#65044=( LENGTH_UNIT ( ) NAMED_UNIT ( * ) SI_UNIT ( .MILLI., .METRE. ) );
#65077=CARTESIAN_POINT ( 'NONE',  ( 10.18706980810188689, -2.126176841940956130, 7.934999999999991616 ) ) ;
#65085=FILL_AREA_STYLE_COLOUR ( '', #90329 ) ;
#65087=( LENGTH_UNIT ( ) NAMED_UNIT ( * ) SI_UNIT ( .MILLI., .METRE. ) );
#65113=UNCERTAINTY_MEASURE_WITH_UNIT (LENGTH_MEASURE( 1.000000000000000082E-05 ), #87432, 'distance_accuracy_value', 'NONE');
#65125=CARTESIAN_POINT ( 'NONE',  ( 4.520833333333333037, -6.094999999999989981, -1.633150327867689100 ) ) ;
#65127=CARTESIAN_POINT ( 'NONE',  ( 13.68706980810188512, -2.126176841940956130, 7.934999999999990727 ) ) ;
#65144=ADVANCED_FACE ( 'NONE', ( #100041 ), #58725, .F. ) ;
#65146=CARTESIAN_POINT ( 'NONE',  ( 0.3872656504350777129, -51.96230815476842224, 39.57541490114646621 ) ) ;
#65150=CARTESIAN_POINT ( 'NONE',  ( 131.5423521607622774, -52.00875322212549179, -39.33676470588227403 ) ) ;
#65165=CARTESIAN_POINT ( 'NONE',  ( 184.1499999999998067, -49.85820393249939286, 34.92500000000001847 ) ) ;
#65181=CARTESIAN_POINT ( 'NONE',  ( 18.15040314143521982, 7.934999999999988951, -2.126176841940961904 ) ) ;
#65185=ADVANCED_FACE ( 'NONE', ( #112339 ), #41982, .T. ) ;
#65213=( GEOMETRIC_REPRESENTATION_CONTEXT ( 3 ) GLOBAL_UNCERTAINTY_ASSIGNED_CONTEXT ( ( #44647 ) ) GLOBAL_UNIT_ASSIGNED_CONTEXT ( ( #58733, #85227, #107697 ) ) REPRESENTATION_CONTEXT ( 'NONE', 'WORKASPACE' ) );
#65246=EDGE_CURVE ( 'NONE', #8597, #49412, #81884, .T. ) ;
#65254=CARTESIAN_POINT ( 'NONE',  ( 22.52540314143522338, 2.126176841940962348, 7.934999999999989839 ) ) ;
#65291=EDGE_CURVE ( 'NONE', #47857, #71793, #115861, .T. ) ;
#65295=CARTESIAN_POINT ( 'NONE',  ( 0.1600000000000025013, -7.946673527226693956, -0.3850431644948629772 ) ) ;
#65308=VERTEX_POINT ( 'NONE', #37646 ) ;
#65321=DIRECTION ( 'NONE',  ( 0.000000000000000000, 0.000000000000000000, -1.000000000000000000 ) ) ;
#65332=CARTESIAN_POINT ( 'NONE',  ( 22.89583333333333570, 1.633150327867706864, -6.094999999999981100 ) ) ;
#65347=DIRECTION ( 'NONE',  ( 0.000000000000000000, -1.000000000000000000, 0.000000000000000000 ) ) ;
#65381=VECTOR ( 'NONE', #108934, 1000.000000000000000 ) ;
#65389=CARTESIAN_POINT ( 'NONE',  ( 3.062159117892259808, -48.47815212813054586, 38.14157743968410585 ) ) ;
#65415=STYLED_ITEM ( 'NONE', ( #105059 ), #62206 ) ;
#65428=CARTESIAN_POINT ( 'NONE',  ( 20.92123647476855197, -9.717572351234235426E-16, -7.934999999999990727 ) ) ;
#65468=DIRECTION ( 'NONE',  ( -1.000000000000000000, -0.000000000000000000, -0.000000000000000000 ) ) ;
#65483=MECHANICAL_DESIGN_GEOMETRIC_PRESENTATION_REPRESENTATION('',(#130022),#26128);
#65500=CARTESIAN_POINT ( 'NONE',  ( 0.1600000000000011136, 3.289720434613005118, -7.220939306079887210 ) ) ;
#65524=FILL_AREA_STYLE ('',( #76369 ) ) ;
#65554=EDGE_LOOP ( 'NONE', ( #119885, #130054, #56928, #103911 ) ) ;
#65560=VERTEX_POINT ( 'NONE', #89688 ) ;
#65601=FILL_AREA_STYLE ('',( #11130 ) ) ;
#65612=MECHANICAL_DESIGN_GEOMETRIC_PRESENTATION_REPRESENTATION('',(#128099),#118852);
#65613=CARTESIAN_POINT ( 'NONE',  ( 20.46247294953710849, -7.464222240803106570E-16, -6.094999999999989981 ) ) ;
#65617=CARTESIAN_POINT ( 'NONE',  ( 0.1600000000000011136, 3.289720434613005118, -7.220939306079887210 ) ) ;
#65635=CARTESIAN_POINT ( 'NONE',  ( 128.6958184333952886, -52.10373894832327579, -40.45955814675561157 ) ) ;
#65660=CARTESIAN_POINT ( 'NONE',  ( 52.26932219902325727, -49.14999999999999147, 40.92499999999998295 ) ) ;
#65661=CARTESIAN_POINT ( 'NONE',  ( 152.4000000000000057, -16.48000000000005016, -12.70000000000045404 ) ) ;
#65675=AXIS2_PLACEMENT_3D ( 'NONE', #51153, #96055, #17090 ) ;
#65678=ADVANCED_FACE ( 'NONE', ( #137495 ), #39628, .T. ) ;
#65679=CARTESIAN_POINT ( 'NONE',  ( 156.1499999999997783, -49.14999999999999147, -34.92499999999975557 ) ) ;
#65681=SURFACE_STYLE_USAGE ( .BOTH. , #112694 ) ;
#65683=CARTESIAN_POINT ( 'NONE',  ( 156.1499999999997783, -52.14999999999999147, -62.92499999999978400 ) ) ;
#65686=AXIS2_PLACEMENT_3D ( 'NONE', #6073, #103275, #72137 ) ;
#65733=ORIENTED_EDGE ( 'NONE', *, *, #26901, .T. ) ;
#65749=SURFACE_STYLE_FILL_AREA ( #109197 ) ;
#65759=CARTESIAN_POINT ( 'NONE',  ( 184.1499999999998067, -50.22575108203859173, 35.38524182944927077 ) ) ;
#65777=ORIENTED_EDGE ( 'NONE', *, *, #26827, .T. ) ;
#65788=CARTESIAN_POINT ( 'NONE',  ( 0.6291396162037723450, 5.278424836066147208, 3.047499999999990550 ) ) ;
#65814=CARTESIAN_POINT ( 'NONE',  ( 17.62456980810188867, -6.871911579029512218, 3.967499999999996252 ) ) ;
#65816=DIRECTION ( 'NONE',  ( 1.804112415015877406E-15, 0.000000000000000000, -1.000000000000000000 ) ) ;
#65822=FILL_AREA_STYLE ('',( #65085 ) ) ;
#65837=VERTEX_POINT ( 'NONE', #46797 ) ;
#65846=( NAMED_UNIT ( * ) PLANE_ANGLE_UNIT ( ) SI_UNIT ( $, .RADIAN. ) );
#65849=VERTEX_POINT ( 'NONE', #77949 ) ;
#65860=CARTESIAN_POINT ( 'NONE',  ( 14.72916666666666607, -6.094999999999989093, 1.633150327867691765 ) ) ;
#65861=CARTESIAN_POINT ( 'NONE',  ( 12.66623647476855297, 7.934999999999990727, -1.457635852685135314E-15 ) ) ;
#65870=SURFACE_STYLE_FILL_AREA ( #32496 ) ;
#65885=VERTEX_POINT ( 'NONE', #112012 ) ;
#65908=CARTESIAN_POINT ( 'NONE',  ( 3.600192512601737782, -49.14999999999999147, -40.57313449935462302 ) ) ;
#65910=CARTESIAN_POINT ( 'NONE',  ( 24.39999999999999858, -7.600000000000061817, 33.92499999999998295 ) ) ;
#65911=MECHANICAL_DESIGN_GEOMETRIC_PRESENTATION_REPRESENTATION('',(#107567),#49666);
#65920=STYLED_ITEM ( 'NONE', ( #109099 ), #88505 ) ;
#65966=CARTESIAN_POINT ( 'NONE',  ( 13.60830628287043886, 1.633150327867687324, -6.094999999999991758 ) ) ;
#65976=CARTESIAN_POINT ( 'NONE',  ( 15.96290314143521805, -3.967499999999994476, 6.871911579029513106 ) ) ;
#65980=CARTESIAN_POINT ( 'NONE',  ( 52.51281677483321175, -49.11905619111353616, -40.21880474160295904 ) ) ;
#66058=EDGE_CURVE ( 'NONE', #53362, #63172, #85775, .T. ) ;
#66069=DIRECTION ( 'NONE',  ( 0.000000000000000000, -1.000000000000000000, 0.000000000000000000 ) ) ;
#66082=DIRECTION ( 'NONE',  ( -1.000000000000000000, -0.000000000000000000, 0.000000000000000000 ) ) ;
#66132=CARTESIAN_POINT ( 'NONE',  ( 29.81706980810189478, -2.126176841940956130, 7.934999999999991616 ) ) ;
#66141=CARTESIAN_POINT ( 'NONE',  ( 24.39999999999999858, 1.399999999999987699, -20.40202195861970580 ) ) ;
#66177=PRESENTATION_STYLE_ASSIGNMENT (( #23350 ) ) ;
#66179=EDGE_CURVE ( 'NONE', #74851, #2777, #76973, .T. ) ;
#66192=( LENGTH_UNIT ( ) NAMED_UNIT ( * ) SI_UNIT ( .MILLI., .METRE. ) );
#66228=ADVANCED_FACE ( 'NONE', ( #121258 ), #132167, .F. ) ;
#66268=( BOUNDED_CURVE ( )  B_SPLINE_CURVE ( 3, ( #141777, #110526, #143179, #86678 ),
 .UNSPECIFIED., .F., .T. ) 
 B_SPLINE_CURVE_WITH_KNOTS ( ( 4, 4 ),
 ( 0.1773996044403679528, 1.570796326794896558 ),
 .UNSPECIFIED. ) 
 CURVE ( )  GEOMETRIC_REPRESENTATION_ITEM ( )  RATIONAL_B_SPLINE_CURVE ( ( 1.000000000000000000, 0.8446433258982463110, 0.8446433258982463110, 1.000000000000000000 ) ) 
 REPRESENTATION_ITEM ( '' )  );
#66271=ORIENTED_EDGE ( 'NONE', *, *, #2449, .F. ) ;
#66277=DIRECTION ( 'NONE',  ( 1.000000000000000000, 0.000000000000000000, -0.000000000000000000 ) ) ;
#66293=CARTESIAN_POINT ( 'NONE',  ( 131.5423521607622774, -49.05583548141699168, -39.86617647058817226 ) ) ;
#66297=CARTESIAN_POINT ( 'NONE',  ( 28.19163961620376924, 6.094999999999988205, -1.633150327867694651 ) ) ;
#66318=( NAMED_UNIT ( * ) PLANE_ANGLE_UNIT ( ) SI_UNIT ( $, .RADIAN. ) );
#66326=DIRECTION ( 'NONE',  ( -1.000000000000000000, -0.000000000000000000, -0.000000000000000000 ) ) ;
#66336=SURFACE_STYLE_USAGE ( .BOTH. , #13337 ) ;
#66344=SURFACE_STYLE_FILL_AREA ( #22085 ) ;
#66366=UNCERTAINTY_MEASURE_WITH_UNIT (LENGTH_MEASURE( 1.000000000000000082E-05 ), #12189, 'distance_accuracy_value', 'NONE');
#66393=CARTESIAN_POINT ( 'NONE',  ( 3.000000000000000000, 0.9892420537897061994, -14.41609864557725729 ) ) ;
#66433=FILL_AREA_STYLE ('',( #121493 ) ) ;
#66470=CARTESIAN_POINT ( 'NONE',  ( 0.9208062828704389746, 3.047499999999997655, 5.278424836066143655 ) ) ;
#66476=VECTOR ( 'NONE', #101065, 1000.000000000000000 ) ;
#66479=CARTESIAN_POINT ( 'NONE',  ( 25.39999999999999858, 0.000000000000000000, 0.000000000000000000 ) ) ;
#66484=VERTEX_POINT ( 'NONE', #128421 ) ;
#66491=ORIENTED_EDGE ( 'NONE', *, *, #140761, .T. ) ;
#66496=CARTESIAN_POINT ( 'NONE',  ( 11.20790314143521904, -6.871911579029513106, -3.967499999999993587 ) ) ;
#66537=CARTESIAN_POINT ( 'NONE',  ( 9.916666666666667851, 5.278424836066147208, 3.047499999999990550 ) ) ;
#66538=CARTESIAN_POINT ( 'NONE',  ( 14.70790314143522082, -6.871911579029513106, -3.967499999999993587 ) ) ;
#66570=ORIENTED_EDGE ( 'NONE', *, *, #89884, .F. ) ;
#66572=STYLED_ITEM ( 'NONE', ( #47119 ), #34639 ) ;
#66586=CARTESIAN_POINT ( 'NONE',  ( 184.1500000000000057, -43.14999999999999147, -40.92499999999998295 ) ) ;
#66594=DIRECTION ( 'NONE',  ( 0.000000000000000000, -1.000000000000000000, 0.000000000000000000 ) ) ;
#66595=CARTESIAN_POINT ( 'NONE',  ( 17.42123647476855908, -9.717572351234235426E-16, -7.934999999999990727 ) ) ;
#66597=EDGE_CURVE ( 'NONE', #8328, #58706, #91848, .T. ) ;
#66610=ORIENTED_EDGE ( 'NONE', *, *, #116199, .T. ) ;
#66620=TOROIDAL_SURFACE ( 'NONE', #110562, 25.00000000000002487, 3.000000000000000000 ) ;
#66633=LINE ( 'NONE', #91258, #18282 ) ;
#66651=ORIENTED_EDGE ( 'NONE', *, *, #33224, .F. ) ;
#66653=CARTESIAN_POINT ( 'NONE',  ( 14.62913961620377101, 5.278424836066147208, 3.047499999999990550 ) ) ;
#66665=CARTESIAN_POINT ( 'NONE',  ( 16.54623647476855552, -7.934999999999990727, 4.858786175617117713E-16 ) ) ;
#66681=FACE_OUTER_BOUND ( 'NONE', #78792, .T. ) ;
#66688=VERTEX_POINT ( 'NONE', #137517 ) ;
#66704=CARTESIAN_POINT ( 'NONE',  ( 23.45790314143522437, 6.871911579029515771, 3.967499999999989146 ) ) ;
#66768=VERTEX_POINT ( 'NONE', #39652 ) ;
#66774=( GEOMETRIC_REPRESENTATION_CONTEXT ( 3 ) GLOBAL_UNCERTAINTY_ASSIGNED_CONTEXT ( ( #2842 ) ) GLOBAL_UNIT_ASSIGNED_CONTEXT ( ( #105526, #41005, #50464 ) ) REPRESENTATION_CONTEXT ( 'NONE', 'WORKASPACE' ) );
#66832=CARTESIAN_POINT ( 'NONE',  ( 23.83790314143521982, -6.871911579029513106, -3.967499999999993587 ) ) ;
#66916=VERTEX_POINT ( 'NONE', #51942 ) ;
#66945=VECTOR ( 'NONE', #32644, 1000.000000000000000 ) ;
#66977=B_SPLINE_CURVE_WITH_KNOTS ( 'NONE', 3,
 ( #32538, #65908, #56475, #55014, #99179, #23046, #44132, #78917, #59316, #79663, #123844, #125976 ),
 .UNSPECIFIED., .F., .F.,
 ( 4, 2, 2, 2, 2, 4 ),
 ( 4.336808689942017736E-19, 0.001108890051515398897, 0.001663335077273098020, 0.002217780103030797360, 0.003326670154546215123, 0.004435560206061632885 ),
 .UNSPECIFIED. ) ;
#66984=EDGE_CURVE ( 'NONE', #43368, #58880, #125832, .T. ) ;
#67002=CARTESIAN_POINT ( 'NONE',  ( 3.129569808101886341, -3.967499999999998028, -6.871911579029511330 ) ) ;
#67035=CARTESIAN_POINT ( 'NONE',  ( 153.4000000000000057, -1.600000000000086020, -34.92499999999998295 ) ) ;
#67048=( GEOMETRIC_REPRESENTATION_CONTEXT ( 3 ) GLOBAL_UNCERTAINTY_ASSIGNED_CONTEXT ( ( #128902 ) ) GLOBAL_UNIT_ASSIGNED_CONTEXT ( ( #122294, #65846, #78836 ) ) REPRESENTATION_CONTEXT ( 'NONE', 'WORKASPACE' ) );
#67066=CARTESIAN_POINT ( 'NONE',  ( 149.2199999999997999, -3.180000000000061444, -31.92499999999998295 ) ) ;
#67075=CARTESIAN_POINT ( 'NONE',  ( 52.60764783923757193, -49.05583548141699879, 39.86617647058822200 ) ) ;
#67089=EDGE_CURVE ( 'NONE', #71281, #94899, #7686, .T. ) ;
#67143=VERTEX_POINT ( 'NONE', #24842 ) ;
#67148=CARTESIAN_POINT ( 'NONE',  ( 3.983306282870438864, 6.094999999999991758, 1.633150327867686880 ) ) ;
#67156=CARTESIAN_POINT ( 'NONE',  ( 2.816639616203773677, -1.633150327867687102, -6.094999999999992646 ) ) ;
#67171=CARTESIAN_POINT ( 'NONE',  ( 10.54580628287044064, 5.278424836066143655, -3.047499999999997655 ) ) ;
#67199=CARTESIAN_POINT ( 'NONE',  ( 14.99956980810188689, -3.967499999999998028, -6.871911579029511330 ) ) ;
#67200=DIRECTION ( 'NONE',  ( -0.7071067811865487940, 0.000000000000000000, 0.7071067811865463515 ) ) ;
#67205=ORIENTED_EDGE ( 'NONE', *, *, #49610, .T. ) ;
#67207=DIRECTION ( 'NONE',  ( 1.000000000000000000, 0.000000000000000000, 0.000000000000000000 ) ) ;
#67216=DIRECTION ( 'NONE',  ( 0.000000000000000000, -1.000000000000000000, 0.000000000000000000 ) ) ;
#67225=( GEOMETRIC_REPRESENTATION_CONTEXT ( 3 ) GLOBAL_UNCERTAINTY_ASSIGNED_CONTEXT ( ( #117296 ) ) GLOBAL_UNIT_ASSIGNED_CONTEXT ( ( #65087, #28874, #106379 ) ) REPRESENTATION_CONTEXT ( 'NONE', 'WORKASPACE' ) );
#67229=CARTESIAN_POINT ( 'NONE',  ( 17.10830628287044419, 1.633150327867706864, -6.094999999999981100 ) ) ;
#67234=DIRECTION ( 'NONE',  ( 0.000000000000000000, -1.000000000000000000, 0.000000000000000000 ) ) ;
#67247=CARTESIAN_POINT ( 'NONE',  ( 10.50000000000000000, 0.000000000000000000, 6.094999999999989981 ) ) ;
#67269=DIRECTION ( 'NONE',  ( 0.000000000000000000, 0.000000000000000000, 1.000000000000000000 ) ) ;
#67310=CARTESIAN_POINT ( 'NONE',  ( 24.71290314143521982, 3.967499999999992699, -6.871911579029513994 ) ) ;
#67321=ORIENTED_EDGE ( 'NONE', *, *, #80568, .F. ) ;
#67349=ORIENTED_EDGE ( 'NONE', *, *, #14329, .F. ) ;
#67370=ORIENTED_EDGE ( 'NONE', *, *, #58049, .F. ) ;
#67392=CARTESIAN_POINT ( 'NONE',  ( 14.94206980810188590, 7.934999999999993392, 2.126176841940951689 ) ) ;
#67398=ORIENTED_EDGE ( 'NONE', *, *, #83543, .F. ) ;
#67409=DIRECTION ( 'NONE',  ( 0.000000000000000000, 0.000000000000000000, 1.000000000000000000 ) ) ;
#67414=DIRECTION ( 'NONE',  ( 0.000000000000000000, -1.000000000000000000, 0.000000000000000000 ) ) ;
#67426=ORIENTED_EDGE ( 'NONE', *, *, #33006, .F. ) ;
#67437=CARTESIAN_POINT ( 'NONE',  ( 22.72873647476856007, 5.808823158059031044, -5.808823158059038150 ) ) ;
#67528=CARTESIAN_POINT ( 'NONE',  ( 24.10830628287044419, 1.633150327867706864, -6.094999999999981100 ) ) ;
#67535=( BOUNDED_SURFACE ( )  B_SPLINE_SURFACE ( 3, 2, ( 
 ( #119348, #20765, #7736 ),
 ( #29492, #76618, #40411 ),
 ( #129519, #109922, #96170 ),
 ( #9132, #10586, #109206 ),
 ( #41819, #141868, #128818 ),
 ( #42563, #120789, #21500 ),
 ( #118657, #141110, #30219 ),
 ( #62880, #52681, #41100 ),
 ( #54164, #86035, #85295 ),
 ( #95470, #20042, #86764 ),
 ( #65759, #30963, #130987 ),
 ( #75882, #98350, #139736 ) ),
 .UNSPECIFIED., .F., .F., .F. ) 
 B_SPLINE_SURFACE_WITH_KNOTS ( ( 4, 2, 2, 2, 2, 4 ),
 ( 3, 3 ),
 ( 0.000000000000000000, 0.001647923167088021727, 0.002471884750632032807, 0.003295846334176043453, 0.004943769501264065613, 0.006591692668352086906 ),
 ( 0.000000000000000000, 1.000000000000000000 ),
 .UNSPECIFIED. ) 
 GEOMETRIC_REPRESENTATION_ITEM ( )  RATIONAL_B_SPLINE_SURFACE ( (
 ( 1.000000000000000000, 0.7071067811865475727, 1.000000000000000000),
 ( 1.000000000000000000, 0.7122033721490172997, 1.000000000000000000),
 ( 1.000000000000000000, 0.7158366153114614772, 1.000000000000000000),
 ( 1.000000000000000000, 0.7192720032936079644, 1.000000000000000000),
 ( 1.000000000000000000, 0.7200809050419507695, 1.000000000000000000),
 ( 1.000000000000000000, 0.7210491446662772308, 1.000000000000000000),
 ( 1.000000000000000000, 0.7212054070302064135, 1.000000000000000000),
 ( 1.000000000000000000, 0.7207522793910704495, 1.000000000000000000),
 ( 1.000000000000000000, 0.7192424821650112987, 1.000000000000000000),
 ( 1.000000000000000000, 0.7143802006613869660, 1.000000000000000000),
 ( 1.000000000000000000, 0.7109884861397428590, 1.000000000000000000),
 ( 1.000000000000000000, 0.7071067811865475727, 1.000000000000000000) ) ) 
 REPRESENTATION_ITEM ( '' )  SURFACE ( )  );
#67570=CARTESIAN_POINT ( 'NONE',  ( 27.77540314143521982, -2.126176841940958351, -7.934999999999989839 ) ) ;
#67586=STYLED_ITEM ( 'NONE', ( #103648 ), #98966 ) ;
#67623=DIRECTION ( 'NONE',  ( 1.000000000000000000, 0.000000000000000000, 0.000000000000000000 ) ) ;
#67646=DIRECTION ( 'NONE',  ( 1.000000000000000000, 0.000000000000000000, 0.000000000000000000 ) ) ;
#67653=EDGE_CURVE ( 'NONE', #65849, #104144, #71059, .T. ) ;
#67669=ORIENTED_EDGE ( 'NONE', *, *, #83543, .T. ) ;
#67734=TOROIDAL_SURFACE ( 'NONE', #104738, 3.000000000000000000, 3.000000000000000000 ) ;
#67738=ORIENTED_EDGE ( 'NONE', *, *, #46056, .F. ) ;
#67749=CARTESIAN_POINT ( 'NONE',  ( 1.087903141435219379, 6.871911579029515771, 3.967499999999989146 ) ) ;
#67762=EDGE_CURVE ( 'NONE', #21857, #52815, #81610, .T. ) ;
#67763=SURFACE_STYLE_USAGE ( .BOTH. , #12612 ) ;
#67766=DIRECTION ( 'NONE',  ( 0.000000000000000000, 0.000000000000000000, 1.000000000000000000 ) ) ;
#67772=VERTEX_POINT ( 'NONE', #70370 ) ;
#67788=DIRECTION ( 'NONE',  ( 0.000000000000000000, 5.559056632600921604E-15, -1.000000000000000000 ) ) ;
#67800=SURFACE_SIDE_STYLE ('',( #26402 ) ) ;
#67804=SURFACE_SIDE_STYLE ('',( #45332 ) ) ;
#67813=TOROIDAL_SURFACE ( 'NONE', #86304, 5.000000000000000000, 1.000000000000000000 ) ;
#67902=VECTOR ( 'NONE', #133330, 1000.000000000000000 ) ;
#67912=DIRECTION ( 'NONE',  ( 1.000000000000000000, 0.000000000000000000, -0.000000000000000000 ) ) ;
#67927=CARTESIAN_POINT ( 'NONE',  ( 7.045806282870439752, 5.278424836066143655, -3.047499999999997655 ) ) ;
#67955=COLOUR_RGB ( '', 0.08235294, 0.09019608, 0.10196078) ;
#67958=CARTESIAN_POINT ( 'NONE',  ( 11.49956980810188689, -3.967499999999998028, -6.871911579029511330 ) ) ;
#67963=ORIENTED_EDGE ( 'NONE', *, *, #119198, .T. ) ;
#67965=UNCERTAINTY_MEASURE_WITH_UNIT (LENGTH_MEASURE( 1.000000000000000082E-05 ), #30207, 'distance_accuracy_value', 'NONE');
#67973=LINE ( 'NONE', #112159, #13210 ) ;
#67999=SURFACE_SIDE_STYLE ('',( #100589 ) ) ;
#68006=CARTESIAN_POINT ( 'NONE',  ( 11.22916666666666430, -6.094999999999989093, 1.633150327867691765 ) ) ;
#68007=CARTESIAN_POINT ( 'NONE',  ( 24.77040314143521726, -7.934999999999988951, 2.126176841940957907 ) ) ;
#68021=CARTESIAN_POINT ( 'NONE',  ( 127.6280169629029331, -46.44627868284427308, -35.89947574910254957 ) ) ;
#68024=DIRECTION ( 'NONE',  ( 0.000000000000000000, -1.000000000000000000, 0.000000000000000000 ) ) ;
#68112=CARTESIAN_POINT ( 'NONE',  ( 0.000000000000000000, 1.399999999999987699, -20.40202195861970580 ) ) ;
#68134=CARTESIAN_POINT ( 'NONE',  ( 18.87956980810189123, 3.967499999999998916, 6.871911579029510442 ) ) ;
#68141=VERTEX_POINT ( 'NONE', #19158 ) ;
#68159=CARTESIAN_POINT ( 'NONE',  ( 61.46640106136302961, -43.14999999999999147, -34.92499999999998295 ) ) ;
#68167=SURFACE_STYLE_FILL_AREA ( #123233 ) ;
#68168=UNCERTAINTY_MEASURE_WITH_UNIT (LENGTH_MEASURE( 1.000000000000000082E-05 ), #118302, 'distance_accuracy_value', 'NONE');
#68179=CARTESIAN_POINT ( 'NONE',  ( 17.77040314143522082, -7.934999999999989839, 2.126176841940957907 ) ) ;
#68195=CARTESIAN_POINT ( 'NONE',  ( 0.000000000000000000, 0.000000000000000000, 0.000000000000000000 ) ) ;
#68206=CARTESIAN_POINT ( 'NONE',  ( 152.4000000000000057, 25.96999999999993847, 33.92499999999998295 ) ) ;
#68233=TOROIDAL_SURFACE ( 'NONE', #61307, 2.000000000000000000, 1.000000000000000000 ) ;
#68239=ORIENTED_EDGE ( 'NONE', *, *, #113154, .T. ) ;
#68242=( BOUNDED_CURVE ( )  B_SPLINE_CURVE ( 2, ( #125255, #135443, #47049, #17709, #59325, #25947, #36127, #124544, #92606, #25215, #125984, #23806, #136837 ),
 .UNSPECIFIED., .F., .F. ) 
 B_SPLINE_CURVE_WITH_KNOTS ( ( 3, 2, 2, 2, 2, 2, 3 ),
 ( 0.2500000000000000000, 0.2583333333333333592, 0.2666666666666666630, 0.2750000000000000222, 0.2833333333333333814, 0.2916666666666667407, 0.3000000000000000444 ),
 .UNSPECIFIED. ) 
 CURVE ( )  GEOMETRIC_REPRESENTATION_ITEM ( )  RATIONAL_B_SPLINE_CURVE ( ( 1.000000000000000000, 0.9659258262890683122, 1.000000000000000000, 0.9659258262890683122, 1.000000000000000000, 0.9659258262890683122, 1.000000000000000000, 0.9659258262890683122, 1.000000000000000000, 0.9659258262890683122, 1.000000000000000000, 0.9659258262890680902, 1.000000000000000222 ) ) 
 REPRESENTATION_ITEM ( '' )  );
#68254=DIRECTION ( 'NONE',  ( -0.9707728879609285322, 0.000000000000000000, 0.2399999999999971323 ) ) ;
#68280=VERTEX_POINT ( 'NONE', #119861 ) ;
#68287=CARTESIAN_POINT ( 'NONE',  ( 166.3240464593592947, 26.96999999999994557, -33.19920214581096474 ) ) ;
#68295=CARTESIAN_POINT ( 'NONE',  ( 24.12956980810188767, -3.967499999999998028, -6.871911579029511330 ) ) ;
#68301=VECTOR ( 'NONE', #71569, 1000.000000000000000 ) ;
#68341=DIRECTION ( 'NONE',  ( 0.000000000000000000, 0.000000000000000000, 1.000000000000000000 ) ) ;
#68372=DIRECTION ( 'NONE',  ( -1.000000000000000000, -0.000000000000000000, -0.000000000000000000 ) ) ;
#68373=EDGE_CURVE ( 'NONE', #98765, #90432, #49220, .T. ) ;
#68415=FILL_AREA_STYLE_COLOUR ( '', #58570 ) ;
#68420=CARTESIAN_POINT ( 'NONE',  ( 151.4000000000000057, -16.48000000000005016, -34.92499999999998295 ) ) ;
#68450=( LENGTH_UNIT ( ) NAMED_UNIT ( * ) SI_UNIT ( .MILLI., .METRE. ) );
#68458=ADVANCED_FACE ( 'NONE', ( #24157 ), #48283, .T. ) ;
#68460=CARTESIAN_POINT ( 'NONE',  ( 3.421236474768552860, -9.717572351234235426E-16, -7.934999999999990727 ) ) ;
#68488=CARTESIAN_POINT ( 'NONE',  ( -0.02126352523144718967, -5.808823158059033709, 5.808823158059035485 ) ) ;
#68496=MECHANICAL_DESIGN_GEOMETRIC_PRESENTATION_REPRESENTATION('',(#24283),#63818);
#68520=CARTESIAN_POINT ( 'NONE',  ( 0.000000000000000000, 0.000000000000000000, 8.094999999999991758 ) ) ;
#68585=ORIENTED_EDGE ( 'NONE', *, *, #102081, .F. ) ;
#68589=DIRECTION ( 'NONE',  ( 1.000000000000000000, 0.000000000000000000, 0.000000000000000000 ) ) ;
#68617=CARTESIAN_POINT ( 'NONE',  ( 4.420806282870438864, 3.047499999999997655, 5.278424836066143655 ) ) ;
#68629=FACE_OUTER_BOUND ( 'NONE', #2002, .T. ) ;
#68637=DIRECTION ( 'NONE',  ( 0.000000000000000000, -0.000000000000000000, -1.000000000000000000 ) ) ;
#68645=CARTESIAN_POINT ( 'NONE',  ( 23.31206980810188512, 7.934999999999993392, 2.126176841940951689 ) ) ;
#68665=CARTESIAN_POINT ( 'NONE',  ( 152.4000000000000057, 7.919999999999947526, 21.67769999999994113 ) ) ;
#68675=CARTESIAN_POINT ( 'NONE',  ( 25.39999999999999858, -16.48000000000005016, 12.69999999999954632 ) ) ;
#68683=CIRCLE ( 'NONE', #29224, 2.999999999999997780 ) ;
#68686=LINE ( 'NONE', #45517, #83310 ) ;
#68691=CARTESIAN_POINT ( 'NONE',  ( 15.75000000000000000, -7.464222240803106570E-16, -6.094999999999989981 ) ) ;
#68693=( NAMED_UNIT ( * ) PLANE_ANGLE_UNIT ( ) SI_UNIT ( $, .RADIAN. ) );
#68743=DIRECTION ( 'NONE',  ( 0.000000000000000000, 0.000000000000000000, -1.000000000000000000 ) ) ;
#68751=CARTESIAN_POINT ( 'NONE',  ( 22.23373647476855197, 5.808823158059035485, 5.808823158059032821 ) ) ;
#68768=CARTESIAN_POINT ( 'NONE',  ( 24.50000000000000000, 0.000000000000000000, 6.094999999999989981 ) ) ;
#68781=DIRECTION ( 'NONE',  ( 0.000000000000000000, 0.000000000000000000, 1.000000000000000000 ) ) ;
#68798=DIRECTION ( 'NONE',  ( -0.000000000000000000, 1.000000000000000000, -0.000000000000000000 ) ) ;
#68817=SURFACE_STYLE_USAGE ( .BOTH. , #26005 ) ;
#68824=CARTESIAN_POINT ( 'NONE',  ( 32.73373647476854842, 5.808823158059036373, 5.808823158059032821 ) ) ;
#68866=CARTESIAN_POINT ( 'NONE',  ( 17.47873647476855652, -5.808823158059033709, 5.808823158059035485 ) ) ;
#68867=CARTESIAN_POINT ( 'NONE',  ( 1.728736474768552522, 5.808823158059031044, -5.808823158059037262 ) ) ;
#68885=FACE_OUTER_BOUND ( 'NONE', #13163, .T. ) ;
#68907=EDGE_CURVE ( 'NONE', #80864, #121754, #47126, .T. ) ;
#68924=CARTESIAN_POINT ( 'NONE',  ( 25.39999999999999858, -14.29000000000013593, 12.69999999999954632 ) ) ;
#68926=AXIS2_PLACEMENT_3D ( 'NONE', #7383, #130642, #97231 ) ;
#68939=( LENGTH_UNIT ( ) NAMED_UNIT ( * ) SI_UNIT ( .MILLI., .METRE. ) );
#68945=SURFACE_SIDE_STYLE ('',( #36296 ) ) ;
#68970=( NAMED_UNIT ( * ) PLANE_ANGLE_UNIT ( ) SI_UNIT ( $, .RADIAN. ) );
#68983=CARTESIAN_POINT ( 'NONE',  ( 28.06706980810189123, 2.126176841940952134, -7.934999999999993392 ) ) ;
#68984=CARTESIAN_POINT ( 'NONE',  ( 0.06706980810188606368, 2.126176841940952134, -7.934999999999993392 ) ) ;
#68985=VERTEX_POINT ( 'NONE', #76795 ) ;
#68987=VECTOR ( 'NONE', #76441, 1000.000000000000000 ) ;
#69018=LINE ( 'NONE', #12458, #27379 ) ;
#69039=CARTESIAN_POINT ( 'NONE',  ( 0.2751413021719010255, -7.484932044345631752, 2.345161579649363670 ) ) ;
#69054=CARTESIAN_POINT ( 'NONE',  ( 0.6154894137848396785, 7.435533126890685907, -0.9100370299028263110 ) ) ;
#69055=FILL_AREA_STYLE ('',( #113965 ) ) ;
#69154=CARTESIAN_POINT ( 'NONE',  ( 1.525403141435219379, 2.126176841940962348, 7.934999999999989839 ) ) ;
#69165=AXIS2_PLACEMENT_3D ( 'NONE', #26226, #59586, #68341 ) ;
#69193=UNCERTAINTY_MEASURE_WITH_UNIT (LENGTH_MEASURE( 1.000000000000000082E-05 ), #102998, 'distance_accuracy_value', 'NONE');
#69205=CIRCLE ( 'NONE', #122462, 25.00000000000002487 ) ;
#69219=UNCERTAINTY_MEASURE_WITH_UNIT (LENGTH_MEASURE( 1.000000000000000082E-05 ), #31054, 'distance_accuracy_value', 'NONE');
#69233=( GEOMETRIC_REPRESENTATION_CONTEXT ( 3 ) GLOBAL_UNCERTAINTY_ASSIGNED_CONTEXT ( ( #121756 ) ) GLOBAL_UNIT_ASSIGNED_CONTEXT ( ( #136385, #50110, #139278 ) ) REPRESENTATION_CONTEXT ( 'NONE', 'WORKASPACE' ) );
#69242=EDGE_LOOP ( 'NONE', ( #49488, #81289 ) ) ;
#69272=ADVANCED_FACE ( 'NONE', ( #81793 ), #136844, .T. ) ;
#69275=ORIENTED_EDGE ( 'NONE', *, *, #40579, .T. ) ;
#69285=SURFACE_STYLE_FILL_AREA ( #125071 ) ;
#69301=( LENGTH_UNIT ( ) NAMED_UNIT ( * ) SI_UNIT ( .MILLI., .METRE. ) );
#69320=CARTESIAN_POINT ( 'NONE',  ( 1.795806282870439308, -5.278424836066144543, 3.047499999999995879 ) ) ;
#69327=AXIS2_PLACEMENT_3D ( 'NONE', #75070, #53265, #77900 ) ;
#69330=SURFACE_SIDE_STYLE ('',( #2606 ) ) ;
#69343=FACE_BOUND ( 'NONE', #97853, .T. ) ;
#69351=VECTOR ( 'NONE', #86141, 1000.000000000000000 ) ;
#69356=CARTESIAN_POINT ( 'NONE',  ( 25.20790314143522082, -6.871911579029513106, -3.967499999999993587 ) ) ;
#69372=DIRECTION ( 'NONE',  ( -1.000000000000000000, -0.000000000000000000, -0.000000000000000000 ) ) ;
#69399=CARTESIAN_POINT ( 'NONE',  ( 24.20833333333333570, 3.047499999999997655, 5.278424836066143655 ) ) ;
#69400=CARTESIAN_POINT ( 'NONE',  ( 25.39999999999999503, -5.131256043349313067, -6.052638797879072108 ) ) ;
#69413=CARTESIAN_POINT ( 'NONE',  ( 124.4403572661730948, -44.90675832753631624, -35.11767176072513763 ) ) ;
#69422=VERTEX_POINT ( 'NONE', #42569 ) ;
#69449=ORIENTED_EDGE ( 'NONE', *, *, #51783, .F. ) ;
#69463=CARTESIAN_POINT ( 'NONE',  ( 21.50456980810188412, 6.871911579029510442, -3.967499999999998916 ) ) ;
#69498=TOROIDAL_SURFACE ( 'NONE', #81082, 9.000000000000001776, 3.000000000000000000 ) ;
#69517=STYLED_ITEM ( 'NONE', ( #124950 ), #71398 ) ;
#69533=CARTESIAN_POINT ( 'NONE',  ( 25.39999999999999858, 0.000000000000000000, 6.094999999999989093 ) ) ;
#69535=CARTESIAN_POINT ( 'NONE',  ( 24.71290314143521982, 3.967499999999992699, -6.871911579029513994 ) ) ;
#69564=CARTESIAN_POINT ( 'NONE',  ( 56.09195796767219377, -46.73296206246176610, -36.09967824800666136 ) ) ;
#69572=( LENGTH_UNIT ( ) NAMED_UNIT ( * ) SI_UNIT ( .MILLI., .METRE. ) );
#69573=UNCERTAINTY_MEASURE_WITH_UNIT (LENGTH_MEASURE( 1.000000000000000082E-05 ), #63765, 'distance_accuracy_value', 'NONE');
#69584=CARTESIAN_POINT ( 'NONE',  ( 19.52040314143522437, 7.934999999999989839, -2.126176841940961904 ) ) ;
#69586=CARTESIAN_POINT ( 'NONE',  ( 0.1600000000000009748, -7.113645484598424495, 3.515717980648092045 ) ) ;
#69613=CARTESIAN_POINT ( 'NONE',  ( 2.999999999999999112, -43.14999999999999147, 40.92499999999998295 ) ) ;
#69632=CARTESIAN_POINT ( 'NONE',  ( 12.25000000000000000, -7.464222240803106570E-16, -6.094999999999989981 ) ) ;
#69643=FILL_AREA_STYLE_COLOUR ( '', #64630 ) ;
#69662=( LENGTH_UNIT ( ) NAMED_UNIT ( * ) SI_UNIT ( .MILLI., .METRE. ) );
#69663=EDGE_CURVE ( 'NONE', #71793, #47857, #69205, .T. ) ;
#69668=STYLED_ITEM ( 'NONE', ( #55457 ), #82181 ) ;
#69686=SURFACE_STYLE_FILL_AREA ( #59516 ) ;
#69687=EDGE_CURVE ( 'NONE', #62641, #91232, #36643, .T. ) ;
#69689=CARTESIAN_POINT ( 'NONE',  ( 156.1500000000000057, -57.14999999999999147, 45.92499999999998295 ) ) ;
#69706=( BOUNDED_CURVE ( )  B_SPLINE_CURVE ( 2, ( #64795, #54635, #98822, #107562, #64075, #74978, #21979, #141643, #74238, #53180, #140896, #143054, #43745 ),
 .UNSPECIFIED., .F., .T. ) 
 B_SPLINE_CURVE_WITH_KNOTS ( ( 3, 2, 2, 2, 2, 2, 3 ),
 ( 0.4000000000000001332, 0.4083333333333334370, 0.4166666666666667407, 0.4250000000000000444, 0.4333333333333334036, 0.4416666666666666519, 0.4500000000000000111 ),
 .UNSPECIFIED. ) 
 CURVE ( )  GEOMETRIC_REPRESENTATION_ITEM ( )  RATIONAL_B_SPLINE_CURVE ( ( 0.9999999999999995559, 0.9659258262890687563, 1.000000000000000000, 0.9659258262890683122, 1.000000000000000000, 0.9659258262890683122, 1.000000000000000000, 0.9659258262890683122, 1.000000000000000000, 0.9659258262890683122, 1.000000000000000000, 0.9659258262890683122, 1.000000000000000000 ) ) 
 REPRESENTATION_ITEM ( '' )  );
#69710=CARTESIAN_POINT ( 'NONE',  ( 4.296236474768552860, 7.934999999999990727, -1.457635852685135314E-15 ) ) ;
#69757=FACE_OUTER_BOUND ( 'NONE', #58997, .T. ) ;
#69843=STYLED_ITEM ( 'NONE', ( #113755 ), #65144 ) ;
#69867=( GEOMETRIC_REPRESENTATION_CONTEXT ( 3 ) GLOBAL_UNCERTAINTY_ASSIGNED_CONTEXT ( ( #3891 ) ) GLOBAL_UNIT_ASSIGNED_CONTEXT ( ( #7913, #96334, #98514 ) ) REPRESENTATION_CONTEXT ( 'NONE', 'WORKASPACE' ) );
#69892=CARTESIAN_POINT ( 'NONE',  ( 2.400403141435218934, -7.934999999999989839, 2.126176841940957907 ) ) ;
#69930=CARTESIAN_POINT ( 'NONE',  ( 8.437069808101885116, 2.126176841940952134, -7.934999999999993392 ) ) ;
#69947=AXIS2_PLACEMENT_3D ( 'NONE', #68420, #13259, #47400 ) ;
#69948=SURFACE_STYLE_FILL_AREA ( #27099 ) ;
#69961=FILL_AREA_STYLE ('',( #125738 ) ) ;
#69978=EDGE_CURVE ( 'NONE', #136091, #57246, #32953, .T. ) ;
#70028=ADVANCED_FACE ( 'NONE', ( #25407 ), #113859, .F. ) ;
#70030=( NAMED_UNIT ( * ) PLANE_ANGLE_UNIT ( ) SI_UNIT ( $, .RADIAN. ) );
#70045=( GEOMETRIC_REPRESENTATION_CONTEXT ( 3 ) GLOBAL_UNCERTAINTY_ASSIGNED_CONTEXT ( ( #5845 ) ) GLOBAL_UNIT_ASSIGNED_CONTEXT ( ( #115592, #40262, #105460 ) ) REPRESENTATION_CONTEXT ( 'NONE', 'WORKASPACE' ) );
#70067=CARTESIAN_POINT ( 'NONE',  ( 9.816639616203772789, -1.633150327867691987, -6.094999999999989093 ) ) ;
#70077=DIRECTION ( 'NONE',  ( 0.000000000000000000, 1.000000000000000000, 0.000000000000000000 ) ) ;
#70089=SURFACE_SIDE_STYLE ('',( #125866 ) ) ;
#70100=CARTESIAN_POINT ( 'NONE',  ( 24.91623647476855652, -7.934999999999990727, 4.858786175617117713E-16 ) ) ;
#70101=CARTESIAN_POINT ( 'NONE',  ( 122.6835989386367345, -43.14999999999999147, 34.92499999999998295 ) ) ;
#70105=DIRECTION ( 'NONE',  ( 0.000000000000000000, 2.921639538487157626E-15, -1.000000000000000000 ) ) ;
#70138=ADVANCED_FACE ( 'NONE', ( #7935, #31856 ), #86952, .F. ) ;
#70146=CARTESIAN_POINT ( 'NONE',  ( 25.37500000000000000, -6.094999999999989981, 3.732111120401553285E-16 ) ) ;
#70160=AXIS2_PLACEMENT_3D ( 'NONE', #92292, #91599, #58318 ) ;
#70165=( NAMED_UNIT ( * ) PLANE_ANGLE_UNIT ( ) SI_UNIT ( $, .RADIAN. ) );
#70167=ORIENTED_EDGE ( 'NONE', *, *, #79423, .F. ) ;
#70208=CYLINDRICAL_SURFACE ( 'NONE', #6324, 5.999999999999998224 ) ;
#70264=AXIS2_PLACEMENT_3D ( 'NONE', #115256, #80562, #47261 ) ;
#70271=DIRECTION ( 'NONE',  ( -1.000000000000000000, -0.000000000000000000, -0.000000000000000000 ) ) ;
#70276=CARTESIAN_POINT ( 'NONE',  ( 32.15040314143522693, 7.934999999999989839, -2.126176841940961904 ) ) ;
#70304=ORIENTED_EDGE ( 'NONE', *, *, #49536, .T. ) ;
#70317=CARTESIAN_POINT ( 'NONE',  ( 29.29123647476855652, -9.717572351234235426E-16, -7.934999999999990727 ) ) ;
#70318=CARTESIAN_POINT ( 'NONE',  ( 1.582903141435219485, 3.967499999999992699, -6.871911579029513994 ) ) ;
#70348=CARTESIAN_POINT ( 'NONE',  ( 55.62203754808115264, -51.91654526991819552, 39.52330221398159438 ) ) ;
#70370=CARTESIAN_POINT ( 'NONE',  ( 151.4000000000000057, -17.48000000000005016, -12.70000000000043272 ) ) ;
#70372=CARTESIAN_POINT ( 'NONE',  ( 2.546236474768552860, -7.934999999999990727, 4.858786175617117713E-16 ) ) ;
#70378=FILL_AREA_STYLE_COLOUR ( '', #119550 ) ;
#70395=( BOUNDED_SURFACE ( )  B_SPLINE_SURFACE ( 3, 2, ( 
 ( #103714, #116030, #104445 ),
 ( #83437, #25454, #50799 ),
 ( #116757, #105857, #16733 ),
 ( #14598, #26897, #6516 ),
 ( #94985, #48663, #39953 ),
 ( #124783, #113906, #37802 ),
 ( #82036, #105167, #5104 ),
 ( #93593, #137822, #38499 ),
 ( #82720, #85541, #130518 ),
 ( #18120, #95719, #42081 ),
 ( #139971, #128370, #107995 ),
 ( #131211, #129775, #84175 ) ),
 .UNSPECIFIED., .F., .F., .T. ) 
 B_SPLINE_SURFACE_WITH_KNOTS ( ( 4, 2, 2, 2, 2, 4 ),
 ( 3, 3 ),
 ( 0.000000000000000000, 0.001647923167088043627, 0.002471884750632065333, 0.003295846334176087255, 0.004943769501264130665, 0.006591692668352174510 ),
 ( 0.000000000000000000, 1.000000000000000000 ),
 .UNSPECIFIED. ) 
 GEOMETRIC_REPRESENTATION_ITEM ( )  RATIONAL_B_SPLINE_SURFACE ( (
 ( 1.000000000000000000, 0.7071067811865443531, 1.000000000000000000),
 ( 1.000000000000000000, 0.7122033721496183745, 1.000000000000000000),
 ( 1.000000000000000000, 0.7158366153106693330, 1.000000000000000000),
 ( 1.000000000000000000, 0.7192720032940053132, 1.000000000000000000),
 ( 1.000000000000000000, 0.7200809050417178447, 1.000000000000000000),
 ( 1.000000000000000000, 0.7210491446665048265, 1.000000000000000000),
 ( 1.000000000000000000, 0.7212054070303647313, 1.000000000000000000),
 ( 1.000000000000000000, 0.7207522793907679137, 1.000000000000000000),
 ( 1.000000000000000000, 0.7192424821649825439, 1.000000000000000000),
 ( 1.000000000000000000, 0.7143802006614192734, 1.000000000000000000),
 ( 1.000000000000000000, 0.7109884861397230971, 1.000000000000000000),
 ( 1.000000000000000000, 0.7071067811865492381, 1.000000000000000000) ) ) 
 REPRESENTATION_ITEM ( '' )  SURFACE ( )  );
#70423=CIRCLE ( 'NONE', #107409, 17.45000000000002061 ) ;
#70428=VERTEX_POINT ( 'NONE', #62552 ) ;
#70460=FACE_OUTER_BOUND ( 'NONE', #47544, .T. ) ;
#70516=SURFACE_STYLE_USAGE ( .BOTH. , #37857 ) ;
#70609=CARTESIAN_POINT ( 'NONE',  ( 10.85873647476855197, 5.808823158059031044, -5.808823158059038150 ) ) ;
#70616=CARTESIAN_POINT ( 'NONE',  ( 25.08333333333333570, -5.278424836066144543, 3.047499999999995879 ) ) ;
#70633=CARTESIAN_POINT ( 'NONE',  ( 7.629139616203772789, 5.278424836066147208, 3.047499999999990550 ) ) ;
#70638=EDGE_LOOP ( 'NONE', ( #62357, #119145, #29490, #83870 ) ) ;
#70641=CARTESIAN_POINT ( 'NONE',  ( 7.999569808101885116, -3.967499999999998028, -6.871911579029511330 ) ) ;
#70643=DIRECTION ( 'NONE',  ( 0.000000000000000000, -1.000000000000000000, 0.000000000000000000 ) ) ;
#70648=FILL_AREA_STYLE ('',( #80784 ) ) ;
#70664=ORIENTED_EDGE ( 'NONE', *, *, #40922, .F. ) ;
#70692=LINE ( 'NONE', #4610, #9243 ) ;
#70694=CARTESIAN_POINT ( 'NONE',  ( 2.999999999999999112, 1.399999999999987699, -20.40202195861970580 ) ) ;
#70755=EDGE_LOOP ( 'NONE', ( #124930, #123794, #140751, #94621 ) ) ;
#70762=CARTESIAN_POINT ( 'NONE',  ( 13.02497294953710849, -4.461849672132299993, -4.461849672132299105 ) ) ;
#70782=CARTESIAN_POINT ( 'NONE',  ( 25.39999999999999858, -57.15000000000003411, -15.92500000000064730 ) ) ;
#70789=CARTESIAN_POINT ( 'NONE',  ( 24.47873647476856007, -5.808823158059033709, 5.808823158059035485 ) ) ;
#70798=FACE_OUTER_BOUND ( 'NONE', #55826, .T. ) ;
#70800=UNCERTAINTY_MEASURE_WITH_UNIT (LENGTH_MEASURE( 1.000000000000000082E-05 ), #102105, 'distance_accuracy_value', 'NONE');
#70836=CARTESIAN_POINT ( 'NONE',  ( 22.75000000000000355, -7.464222240803106570E-16, -6.094999999999989981 ) ) ;
#70859=SURFACE_STYLE_FILL_AREA ( #125942 ) ;
#70882=DIRECTION ( 'NONE',  ( -1.000000000000000000, -0.000000000000000000, -0.000000000000000000 ) ) ;
#70891=CARTESIAN_POINT ( 'NONE',  ( 25.40000000000000568, -6.165261453458376728, -3.761236098458531796 ) ) ;
#70905=SURFACE_SIDE_STYLE ('',( #17211 ) ) ;
#70937=SURFACE_SIDE_STYLE ('',( #15083 ) ) ;
#70954=CARTESIAN_POINT ( 'NONE',  ( 26.02540314143521982, 2.126176841940962348, 7.934999999999989839 ) ) ;
#70979=SURFACE_STYLE_FILL_AREA ( #37638 ) ;
#70990=UNCERTAINTY_MEASURE_WITH_UNIT (LENGTH_MEASURE( 1.000000000000000082E-05 ), #98940, 'distance_accuracy_value', 'NONE');
#71004=CARTESIAN_POINT ( 'NONE',  ( 27.83290314143522437, -3.967499999999994476, 6.871911579029513106 ) ) ;
#71005=CARTESIAN_POINT ( 'NONE',  ( 4.791236474768552966, -9.717572351234235426E-16, -7.934999999999990727 ) ) ;
#71028=DIRECTION ( 'NONE',  ( -1.000000000000000000, 0.000000000000000000, -0.000000000000000000 ) ) ;
#71032=CARTESIAN_POINT ( 'NONE',  ( 0.000000000000000000, -4.600000000000013856, 20.40202195861967382 ) ) ;
#71034=CARTESIAN_POINT ( 'NONE',  ( 52.83697049268917567, -48.90295371244932454, 39.18578444878559708 ) ) ;
#71059=LINE ( 'NONE', #95630, #532 ) ;
#71060=CARTESIAN_POINT ( 'NONE',  ( 4.733736474768551972, 5.808823158059035485, 5.808823158059032821 ) ) ;
#71070=ORIENTED_EDGE ( 'NONE', *, *, #80668, .F. ) ;
#71079=CARTESIAN_POINT ( 'NONE',  ( 25.39999999999999858, -5.520864266206504263E-14, 0.000000000000000000 ) ) ;
#71104=CARTESIAN_POINT ( 'NONE',  ( 156.1499999999997783, -57.14999999999999147, 34.92500000000004690 ) ) ;
#71131=CARTESIAN_POINT ( 'NONE',  ( 52.60764783923754351, -49.05583548141699168, -39.86617647058817937 ) ) ;
#71158=FACE_OUTER_BOUND ( 'NONE', #40052, .T. ) ;
#71202=( LENGTH_UNIT ( ) NAMED_UNIT ( * ) SI_UNIT ( .MILLI., .METRE. ) );
#71206=DIRECTION ( 'NONE',  ( 0.000000000000000000, 5.075120898959323014E-15, 1.000000000000000000 ) ) ;
#71211=ORIENTED_EDGE ( 'NONE', *, *, #40207, .T. ) ;
#71235=EDGE_CURVE ( 'NONE', #33799, #46517, #29000, .T. ) ;
#71278=CARTESIAN_POINT ( 'NONE',  ( 17.20833333333333570, 3.047499999999997655, 5.278424836066143655 ) ) ;
#71281=VERTEX_POINT ( 'NONE', #20634 ) ;
#71296=( LENGTH_UNIT ( ) NAMED_UNIT ( * ) SI_UNIT ( .MILLI., .METRE. ) );
#71297=CARTESIAN_POINT ( 'NONE',  ( 6.629569808101885897, -3.967499999999998028, -6.871911579029511330 ) ) ;
#71319=PRESENTATION_STYLE_ASSIGNMENT (( #27075 ) ) ;
#71324=CARTESIAN_POINT ( 'NONE',  ( 9.603736474768549414, 5.808823158059036373, 5.808823158059032821 ) ) ;
#71352=CARTESIAN_POINT ( 'NONE',  ( 11.08333333333333393, -5.278424836066144543, 3.047499999999995879 ) ) ;
#71378=FILL_AREA_STYLE_COLOUR ( '', #93935 ) ;
#71380=CIRCLE ( 'NONE', #6427, 8.094999999999991758 ) ;
#71398=ADVANCED_FACE ( 'NONE', ( #112657 ), #79369, .F. ) ;
#71400=SURFACE_STYLE_FILL_AREA ( #27158 ) ;
#71402=ORIENTED_EDGE ( 'NONE', *, *, #16097, .T. ) ;
#71422=( NAMED_UNIT ( * ) PLANE_ANGLE_UNIT ( ) SI_UNIT ( $, .RADIAN. ) );
#71434=CARTESIAN_POINT ( 'NONE',  ( 156.1499999999997783, -49.14999999999999147, 34.92500000000004690 ) ) ;
#71454=CARTESIAN_POINT ( 'NONE',  ( 17.10830628287044064, 1.633150327867687324, -6.094999999999991758 ) ) ;
#71459=SURFACE_STYLE_USAGE ( .BOTH. , #91089 ) ;
#71511=VECTOR ( 'NONE', #143541, 1000.000000000000000 ) ;
#71513=ORIENTED_EDGE ( 'NONE', *, *, #60900, .T. ) ;
#71539=CARTESIAN_POINT ( 'NONE',  ( 22.45833333333333215, -3.047499999999997211, -5.278424836066143655 ) ) ;
#71562=CARTESIAN_POINT ( 'NONE',  ( 1.470220343760034742, -1.488543484705065811, 6.466294286230377608 ) ) ;
#71569=DIRECTION ( 'NONE',  ( 0.000000000000000000, -1.000000000000000000, 0.000000000000000000 ) ) ;
#71585=MECHANICAL_DESIGN_GEOMETRIC_PRESENTATION_REPRESENTATION('',(#103822),#36797);
#71621=CARTESIAN_POINT ( 'NONE',  ( 12.44163961620377101, -6.094999999999989093, 1.633150327867691542 ) ) ;
#71658=CARTESIAN_POINT ( 'NONE',  ( 31.12956980810189478, -3.967499999999998028, -6.871911579029511330 ) ) ;
#71695=DIRECTION ( 'NONE',  ( -1.000000000000000000, -0.000000000000000000, -0.000000000000000000 ) ) ;
#71708=CARTESIAN_POINT ( 'NONE',  ( 34.39540314143521016, 2.126176841940962348, 7.934999999999989839 ) ) ;
#71709=CARTESIAN_POINT ( 'NONE',  ( 3.770403141435219485, -7.934999999999988951, 2.126176841940957907 ) ) ;
#71719=AXIS2_PLACEMENT_3D ( 'NONE', #33251, #50862, #22287 ) ;
#71720=CARTESIAN_POINT ( 'NONE',  ( 25.39999999999998792, 6.130634315452725858, 3.678650144044258941 ) ) ;
#71723=FACE_OUTER_BOUND ( 'NONE', #86475, .T. ) ;
#71724=CARTESIAN_POINT ( 'NONE',  ( 22.79580628287044064, -5.278424836066144543, 3.047499999999995879 ) ) ;
#71753=CARTESIAN_POINT ( 'NONE',  ( 7.437500000000000000, -4.461849672132299105, 4.461849672132299993 ) ) ;
#71770=CARTESIAN_POINT ( 'NONE',  ( 156.1500000000000057, -49.14999999999999147, -49.92499999999968452 ) ) ;
#71772=CARTESIAN_POINT ( 'NONE',  ( 8.671236474768553748, 0.000000000000000000, 7.934999999999990727 ) ) ;
#71786=CARTESIAN_POINT ( 'NONE',  ( 6.708333333333333925, 3.047499999999997655, 5.278424836066143655 ) ) ;
#71793=VERTEX_POINT ( 'NONE', #134252 ) ;
#71813=CARTESIAN_POINT ( 'NONE',  ( 27.99999999999996803, -49.14999999999999147, 49.92499999999997584 ) ) ;
#71815=EDGE_CURVE ( 'NONE', #79053, #51562, #107, .T. ) ;
#71817=VECTOR ( 'NONE', #94333, 1000.000000000000000 ) ;
#71833=VERTEX_POINT ( 'NONE', #10994 ) ;
#71847=MECHANICAL_DESIGN_GEOMETRIC_PRESENTATION_REPRESENTATION('',(#134345),#97239);
#71860=CARTESIAN_POINT ( 'NONE',  ( 53.41205288902393278, -48.51956544822605366, -36.87500513592858198 ) ) ;
#71892=CARTESIAN_POINT ( 'NONE',  ( 25.39999999999999858, 0.000000000000000000, 0.000000000000000000 ) ) ;
#71926=DIRECTION ( 'NONE',  ( 0.000000000000000000, 0.000000000000000000, 1.000000000000000000 ) ) ;
#71931=ORIENTED_EDGE ( 'NONE', *, *, #140716, .T. ) ;
#71939=FILL_AREA_STYLE_COLOUR ( '', #56187 ) ;
#71968=ORIENTED_EDGE ( 'NONE', *, *, #13671, .T. ) ;
#71982=FACE_OUTER_BOUND ( 'NONE', #31866, .T. ) ;
#71983=CARTESIAN_POINT ( 'NONE',  ( 122.6835989386367345, -57.15000000000010516, 40.92499999999998295 ) ) ;
#72029=CARTESIAN_POINT ( 'NONE',  ( 12.02540314143521982, 2.126176841940962348, 7.934999999999989839 ) ) ;
#72067=CARTESIAN_POINT ( 'NONE',  ( 4.353736474768552966, -5.808823158059035485, -5.808823158059033709 ) ) ;
#72070=CARTESIAN_POINT ( 'NONE',  ( 156.1500000000000057, -57.14999999999999147, 49.92499999999997584 ) ) ;
#72084=DIRECTION ( 'NONE',  ( 0.000000000000000000, 0.000000000000000000, -1.000000000000000000 ) ) ;
#72099=UNCERTAINTY_MEASURE_WITH_UNIT (LENGTH_MEASURE( 1.000000000000000082E-05 ), #18386, 'distance_accuracy_value', 'NONE');
#72137=DIRECTION ( 'NONE',  ( 9.912705577010316675E-16, 0.000000000000000000, 1.000000000000000000 ) ) ;
#72138=STYLED_ITEM ( 'NONE', ( #44670 ), #141443 ) ;
#72143=FILL_AREA_STYLE_COLOUR ( '', #107762 ) ;
#72209=CARTESIAN_POINT ( 'NONE',  ( 14.92080628287044064, 3.047499999999997655, 5.278424836066143655 ) ) ;
#72230=ORIENTED_EDGE ( 'NONE', *, *, #107743, .T. ) ;
#72235=AXIS2_PLACEMENT_3D ( 'NONE', #19324, #9865, #109900 ) ;
#72245=CARTESIAN_POINT ( 'NONE',  ( 32.64540314143522437, -2.126176841940958351, -7.934999999999989839 ) ) ;
#72257=CARTESIAN_POINT ( 'NONE',  ( 0.07239000078343528488, -48.13855614193185772, -37.56434003616170969 ) ) ;
#72291=CARTESIAN_POINT ( 'NONE',  ( 27.41666666666666785, 5.278424836066147208, 3.047499999999990550 ) ) ;
#72305=EDGE_LOOP ( 'NONE', ( #36305, #85904 ) ) ;
#72316=CARTESIAN_POINT ( 'NONE',  ( 25.39999999999999858, -18.48000000000005372, -34.92499999999998295 ) ) ;
#72334=CARTESIAN_POINT ( 'NONE',  ( 184.1500000000000057, -14.29000000000013593, -12.70000000000045404 ) ) ;
#72339=EDGE_LOOP ( 'NONE', ( #66610, #13960, #85760, #50116 ) ) ;
#72356=EDGE_LOOP ( 'NONE', ( #113652, #118631, #26277, #10639 ) ) ;
#72404=CARTESIAN_POINT ( 'NONE',  ( 0.6686314397422480349, -52.14999999947626463, 41.03936837847535912 ) ) ;
#72408=CARTESIAN_POINT ( 'NONE',  ( 4.937069808101886004, 2.126176841940952134, -7.934999999999993392 ) ) ;
#72423=COLOUR_RGB ( '', 0.66274510, 0.83137255, 0.94901961) ;
#72429=DIRECTION ( 'NONE',  ( 0.000000000000000000, 0.7453559924999330066, 0.6666666666666630769 ) ) ;
#72435=CARTESIAN_POINT ( 'NONE',  ( 55.71344734891371075, -51.77943056867386673, -39.18578444878554734 ) ) ;
#72441=( NAMED_UNIT ( * ) SI_UNIT ( $, .STERADIAN. ) SOLID_ANGLE_UNIT ( ) );
#72452=CARTESIAN_POINT ( 'NONE',  ( 26.37456980810188867, 6.871911579029510442, -3.967499999999998916 ) ) ;
#72453=CARTESIAN_POINT ( 'NONE',  ( 3.916236474768552522, -7.934999999999990727, 4.858786175617117713E-16 ) ) ;
#72462=PRODUCT ( '1.0 Base', '1.0 Base', '', ( #93870 ) ) ;
#72468=VECTOR ( 'NONE', #107729, 1000.000000000000000 ) ;
#72513=CARTESIAN_POINT ( 'NONE',  ( 12.75456980810188767, -6.871911579029512218, 3.967499999999996252 ) ) ;
#72525=VECTOR ( 'NONE', #96567, 1000.000000000000000 ) ;
#72543=CARTESIAN_POINT ( 'NONE',  ( 25.39999999999998792, -2.682872131610448907, -7.478867202222028610 ) ) ;
#72545=LINE ( 'NONE', #36996, #7471 ) ;
#72581=ORIENTED_EDGE ( 'NONE', *, *, #52881, .T. ) ;
#72590=CARTESIAN_POINT ( 'NONE',  ( 11.44206980810188767, 7.934999999999993392, 2.126176841940951689 ) ) ;
#72594=CARTESIAN_POINT ( 'NONE',  ( 55.56056557994604361, -52.00875322212549179, -39.86617647058817937 ) ) ;
#72641=( NAMED_UNIT ( * ) PLANE_ANGLE_UNIT ( ) SI_UNIT ( $, .RADIAN. ) );
#72677=SURFACE_STYLE_USAGE ( .BOTH. , #50168 ) ;
#72726=CARTESIAN_POINT ( 'NONE',  ( 128.5894344200537773, -57.14999999999999147, -39.86617647058817226 ) ) ;
#72763=CARTESIAN_POINT ( 'NONE',  ( 12.90040314143522160, -7.934999999999989839, 2.126176841940957907 ) ) ;
#72771=CARTESIAN_POINT ( 'NONE',  ( 9.962472949537104938, -7.464222240803106570E-16, -6.094999999999989981 ) ) ;
#72794=CARTESIAN_POINT ( 'NONE',  ( 2.312069808101886448, 7.934999999999993392, 2.126176841940951689 ) ) ;
#72821=CARTESIAN_POINT ( 'NONE',  ( 10.79166666666666785, -3.047499999999994547, 5.278424836066145431 ) ) ;
#72841=STYLED_ITEM ( 'NONE', ( #109578 ), #18383 ) ;
#72866=SURFACE_STYLE_FILL_AREA ( #116314 ) ;
#72894=MECHANICAL_DESIGN_GEOMETRIC_PRESENTATION_REPRESENTATION('',(#137743),#75241);
#72899=COLOUR_RGB ( '', 0.40784314, 0.44705882, 0.49803922) ;
#72923=CARTESIAN_POINT ( 'NONE',  ( 12.44163961620377101, -6.094999999999989093, 1.633150327867691765 ) ) ;
#72932=EDGE_CURVE ( 'NONE', #112055, #24260, #41010, .T. ) ;
#72952=CARTESIAN_POINT ( 'NONE',  ( 34.54123647476855297, 0.000000000000000000, 7.934999999999990727 ) ) ;
#72977=ORIENTED_EDGE ( 'NONE', *, *, #83646, .T. ) ;
#72999=CARTESIAN_POINT ( 'NONE',  ( 29.16666666666667140, -5.278424836066145431, -3.047499999999993658 ) ) ;
#73054=FACE_OUTER_BOUND ( 'NONE', #51012, .T. ) ;
#73057=( LENGTH_UNIT ( ) NAMED_UNIT ( * ) SI_UNIT ( .MILLI., .METRE. ) );
#73070=CARTESIAN_POINT ( 'NONE',  ( 13.31663961620377279, -1.633150327867691765, -6.094999999999989093 ) ) ;
#73084=CARTESIAN_POINT ( 'NONE',  ( 0.000000000000000000, -5.520864266206504263E-14, 0.000000000000000000 ) ) ;
#73085=CARTESIAN_POINT ( 'NONE',  ( 0.000000000000000000, -14.29000000000013593, 12.69999999999954632 ) ) ;
#73100=PRESENTATION_STYLE_ASSIGNMENT (( #41879 ) ) ;
#73102=CARTESIAN_POINT ( 'NONE',  ( 7.853736474768552966, -5.808823158059035485, -5.808823158059033709 ) ) ;
#73132=ORIENTED_EDGE ( 'NONE', *, *, #92748, .T. ) ;
#73145=CARTESIAN_POINT ( 'NONE',  ( 25.64540314143522082, -2.126176841940958351, -7.934999999999989839 ) ) ;
#73146=CARTESIAN_POINT ( 'NONE',  ( 5.957903141435219929, 6.871911579029515771, 3.967499999999989146 ) ) ;
#73175=CARTESIAN_POINT ( 'NONE',  ( 53.41963127661843203, -48.51451318982864080, 38.21513923099880827 ) ) ;
#73176=ORIENTED_EDGE ( 'NONE', *, *, #111786, .F. ) ;
#73178=AXIS2_PLACEMENT_3D ( 'NONE', #40888, #29990, #28594 ) ;
#73180=ORIENTED_EDGE ( 'NONE', *, *, #6994, .T. ) ;
#73181=CIRCLE ( 'NONE', #80122, 5.999999999999998224 ) ;
#73183=CARTESIAN_POINT ( 'NONE',  ( 8.604166666666669627, -1.633150327867691765, -6.094999999999989093 ) ) ;
#73200=CARTESIAN_POINT ( 'NONE',  ( 11.87956980810188767, 3.967499999999998916, 6.871911579029510442 ) ) ;
#73217=SURFACE_STYLE_FILL_AREA ( #118089 ) ;
#73221=EDGE_LOOP ( 'NONE', ( #83106, #1332, #95031 ) ) ;
#73267=CARTESIAN_POINT ( 'NONE',  ( 9.983736474768551972, -5.808823158059035485, -5.808823158059033709 ) ) ;
#73275=CARTESIAN_POINT ( 'NONE',  ( 131.8806778009766276, -49.14999999999999147, -40.92499999999998295 ) ) ;
#73280=LINE ( 'NONE', #29042, #84002 ) ;
#73344=CARTESIAN_POINT ( 'NONE',  ( 174.7500000000000000, 7.919999999999947526, -18.97500000000001918 ) ) ;
#73396=( NAMED_UNIT ( * ) PLANE_ANGLE_UNIT ( ) SI_UNIT ( $, .RADIAN. ) );
#73404=EDGE_LOOP ( 'NONE', ( #84295, #111671, #88684, #77614 ) ) ;
#73410=DIRECTION ( 'NONE',  ( 0.1737853339090542071, 0.1737853339090537907, 0.9693282805305111216 ) ) ;
#73413=CARTESIAN_POINT ( 'NONE',  ( 16.18750000000000000, 4.461849672132297329, -4.461849672132302658 ) ) ;
#73431=CARTESIAN_POINT ( 'NONE',  ( 8.379569808101887674, 3.967499999999998916, 6.871911579029510442 ) ) ;
#73435=AXIS2_PLACEMENT_3D ( 'NONE', #108106, #29852, #119692 ) ;
#73459=CYLINDRICAL_SURFACE ( 'NONE', #99337, 5.999999999999998224 ) ;
#73465=CARTESIAN_POINT ( 'NONE',  ( 14.99956980810188689, -3.967499999999998028, -6.871911579029511330 ) ) ;
#73523=SURFACE_SIDE_STYLE ('',( #63387 ) ) ;
#73555=AXIS2_PLACEMENT_3D ( 'NONE', #27340, #18593, #51272 ) ;
#73560=ORIENTED_EDGE ( 'NONE', *, *, #54836, .F. ) ;
#73585=ADVANCED_FACE ( 'NONE', ( #13843 ), #58869, .F. ) ;
#73595=CARTESIAN_POINT ( 'NONE',  ( 17.54580628287044064, 5.278424836066143655, -3.047499999999997655 ) ) ;
#73625=CARTESIAN_POINT ( 'NONE',  ( 27.39540314143522437, 2.126176841940962348, 7.934999999999989839 ) ) ;
#73692=CARTESIAN_POINT ( 'NONE',  ( 1.369639479247480862, 4.811953009385816285E-13, 6.725360520752516891 ) ) ;
#73731=DIRECTION ( 'NONE',  ( 1.000000000000000000, -0.000000000000000000, -0.000000000000000000 ) ) ;
#73779=CARTESIAN_POINT ( 'NONE',  ( 153.4000000000000057, -16.48000000000005016, -33.92499999999998295 ) ) ;
#73785=CARTESIAN_POINT ( 'NONE',  ( 3.483440076894412041, -49.11775834062188295, 40.20665288735688137 ) ) ;
#73790=CARTESIAN_POINT ( 'NONE',  ( 2.603736474768552522, 5.808823158059036373, 5.808823158059032821 ) ) ;
#73816=CARTESIAN_POINT ( 'NONE',  ( 26.40000000000000568, -16.48000000000005016, 33.92499999999998295 ) ) ;
#73825=FILL_AREA_STYLE ('',( #29588 ) ) ;
#73833=CARTESIAN_POINT ( 'NONE',  ( 4.958333333333333925, -3.047499999999997211, -5.278424836066143655 ) ) ;
#73834=CARTESIAN_POINT ( 'NONE',  ( 5.666236474768552078, 7.934999999999990727, -1.457635852685135314E-15 ) ) ;
#73841=VERTEX_POINT ( 'NONE', #123201 ) ;
#73861=DIRECTION ( 'NONE',  ( 0.000000000000000000, 0.000000000000000000, 1.000000000000000000 ) ) ;
#73873=CARTESIAN_POINT ( 'NONE',  ( 8.750000000000000000, -7.464222240803106570E-16, -6.094999999999989981 ) ) ;
#73889=EDGE_LOOP ( 'NONE', ( #112388, #79715 ) ) ;
#73895=CARTESIAN_POINT ( 'NONE',  ( 11.00456980810188590, 6.871911579029510442, -3.967499999999998916 ) ) ;
#73898=CARTESIAN_POINT ( 'NONE',  ( 21.87500000000000355, -6.094999999999989981, 3.732111120401553285E-16 ) ) ;
#73908=CARTESIAN_POINT ( 'NONE',  ( 7.000000000000000888, 0.000000000000000000, 6.094999999999989981 ) ) ;
#73965=CARTESIAN_POINT ( 'NONE',  ( 6.483736474768551972, -5.808823158059035485, -5.808823158059033709 ) ) ;
#73973=DIRECTION ( 'NONE',  ( -0.5150380749100710309, 0.000000000000000000, 0.8571673007021021196 ) ) ;
#73977=DIRECTION ( 'NONE',  ( 0.000000000000000000, 0.000000000000000000, 1.000000000000000000 ) ) ;
#74000=DIRECTION ( 'NONE',  ( 0.000000000000000000, 0.000000000000000000, 1.000000000000000000 ) ) ;
#74007=CARTESIAN_POINT ( 'NONE',  ( 3.354166666666667407, 1.633150327867690432, 6.094999999999991758 ) ) ;
#74038=CYLINDRICAL_SURFACE ( 'NONE', #22210, 1.000000000000000888 ) ;
#74050=DIRECTION ( 'NONE',  ( 0.000000000000000000, 0.000000000000000000, -1.000000000000000000 ) ) ;
#74121=AXIS2_PLACEMENT_3D ( 'NONE', #47435, #28500, #39379 ) ;
#74130=EDGE_CURVE ( 'NONE', #78350, #105963, #125369, .T. ) ;
#74137=CARTESIAN_POINT ( 'NONE',  ( 18.44206980810188767, 7.934999999999993392, 2.126176841940951689 ) ) ;
#74173=CARTESIAN_POINT ( 'NONE',  ( 10.77040314143521904, -7.934999999999989839, 2.126176841940957907 ) ) ;
#74183=DIRECTION ( 'NONE',  ( -0.000000000000000000, -0.6666666666666656305, -0.7453559924999307862 ) ) ;
#74211=COLOUR_RGB ( '', 0.40784314, 0.44705882, 0.49803922) ;
#74217=CONICAL_SURFACE ( 'NONE', #111233, 8.094999999999991758, 0.7853981633974466137 ) ;
#74238=CARTESIAN_POINT ( 'NONE',  ( 15.16666666666666785, -5.278424836066145431, -3.047499999999993658 ) ) ;
#74240=SURFACE_STYLE_USAGE ( .BOTH. , #7524 ) ;
#74259=COLOUR_RGB ( '', 0.72549020, 0.75294118, 0.79215686) ;
#74269=AXIS2_PLACEMENT_3D ( 'NONE', #41410, #117523, #74794 ) ;
#74270=COLOUR_RGB ( '', 0.72549020, 0.75294118, 0.79215686) ;
#74279=DIRECTION ( 'NONE',  ( 0.000000000000000000, 0.000000000000000000, -1.000000000000000000 ) ) ;
#74301=CARTESIAN_POINT ( 'NONE',  ( 180.5498074873981125, -49.14999999999999858, -40.57313449935461591 ) ) ;
#74317=CARTESIAN_POINT ( 'NONE',  ( 28.62913961620377279, 5.278424836066147208, 3.047499999999990550 ) ) ;
#74352=CARTESIAN_POINT ( 'NONE',  ( 32.20790314143521726, -6.871911579029513106, -3.967499999999993587 ) ) ;
#74364=CARTESIAN_POINT ( 'NONE',  ( 2.837178562577524071E-15, -50.22575108203882621, -35.38524182944816943 ) ) ;
#74386=CARTESIAN_POINT ( 'NONE',  ( 27.99999999999996803, -49.14999999999999147, 45.92499999999999005 ) ) ;
#74412=ORIENTED_EDGE ( 'NONE', *, *, #92308, .F. ) ;
#74424=SURFACE_STYLE_FILL_AREA ( #6238 ) ;
#74429=( GEOMETRIC_REPRESENTATION_CONTEXT ( 3 ) GLOBAL_UNCERTAINTY_ASSIGNED_CONTEXT ( ( #15817 ) ) GLOBAL_UNIT_ASSIGNED_CONTEXT ( ( #94570, #71422, #59151 ) ) REPRESENTATION_CONTEXT ( 'NONE', 'WORKASPACE' ) );
#74448=EDGE_CURVE ( 'NONE', #100283, #143396, #38156, .T. ) ;
#74469=( BOUNDED_SURFACE ( )  B_SPLINE_SURFACE ( 1, 2, ( 
 ( #33843, #88216, #44750, #108482, #75902, #9162, #110634, #120075, #120817, #54188, #11312, #43286, #22207, #55594, #63629, #132466, #77367, #76641, #21524, #33155, #65788, #121530, #66470, #109946, #10615, #99782, #457, #133161, #69320, #91760, #3307, #113505, #36661, #57742, #25063, #92456, #48261, #101209, #14197, #125105, #1849, #45445, #133850, #57036, #46904, #102665, #68617, #58490, #56341, #34541, #46157, #14909, #78767, #122235, #103335, #23658, #100519, #112800, #24370, #90336, #1163, #37394, #124398, #134587, #67927, #22907, #47597, #35284, #79525, #101931, #123712, #13460, #2594, #91083, #89625, #135304, #122976, #135986, #80906, #35985, #80214, #25790, #136690, #70067, #114231, #59182, #3982, #12761, #67171, #111363, #12053, #112114, #18452, #27938, #62021, #81639, #28676, #106178, #49725, #48994, #139594, #72923, #125843, #105478, #26516, #70762, #4696, #61333, #6142, #15585, #59864, #114907, #62735, #104040, #39554, #16317, #127238, #93193, #72209, #137430, #17747, #117070, #38119, #7593, #17070, #82339, #96038, #6855, #106914, #126524, #5443, #27211, #29350, #71454, #83781, #116378, #73595, #83040, #84485, #117762, #140275, #51134, #40279, #115613, #60610, #95330, #104783, #128681, #51852, #50419, #94605, #93900, #138138, #38824, #138860, #127995, #65613, #32229, #98889, #119910, #87327, #11140, #110470, #19899, #76464, #43818, #64150, #107628, #52540, #119217, #109050, #21350, #130852, #131540, #118507, #96722, #108311, #77190, #140965, #40964, #22042, #85883, #19206, #143123, #85162, #55416, #43117, #31515, #75740, #63464, #121363, #130121, #20614, #120633, #109781, #129378, #42417, #8290, #30822, #9740, #10449, #64869, #54709, #88036, #98204, #99596, #132286, #32974, #75048, #66297, #8983, #30066, #74317, #41669, #53243, #54009, #97460, #141712, #86629, #142431, #11874, #111943, #88770, #56163, #35832, #77877, #25617, #12601, #122800, #100347, #132999, #45280, #122069, #57572, #47439, #998, #80054, #56877, #23482, #89453, #112639 ),
 ( #133688, #101757, #134409, #135824, #1690, #3149, #36508, #59028, #124228, #58319, #34371, #274, #113332, #22734, #14015, #24906, #45981, #79349, #101034, #78591, #67749, #90911, #102500, #69154, #135142, #91602, #123551, #46731, #114062, #69892, #90163, #80748, #124935, #35107, #67002, #24213, #68460, #13300, #14752, #2417, #44572, #111187, #33678, #126360, #139425, #59711, #103182, #84327, #4516, #81471, #17584, #3824, #93743, #5275, #27050, #37219, #18284, #105322, #71297, #48827, #48112, #83607, #115449, #16140, #38654, #93027, #127819, #37953, #117595, #106012, #73431, #50253, #137974, #92293, #103872, #26353, #61851, #114750, #60432, #136517, #15424, #138695, #125671, #128524, #104613, #82189, #137258, #70609, #49561, #82885, #16900, #6682, #127074, #39381, #27765, #72029, #116209, #61172, #5975, #28502, #94442, #72763, #116915, #50961, #95156, #40112, #29190, #19741, #86452, #62556, #43641, #108862, #95874, #64692, #108147, #54542, #42241, #106733, #76287, #8813, #53071, #120444, #98720, #7420, #20440, #121189, #51680, #130679, #140121, #87149, #40799, #98032, #141536, #97266, #9556, #30647, #142266, #74878, #53828, #74137, #31351, #42951, #87861, #32794, #77017, #32055, #131371, #75570, #10284, #132100, #85000, #119740, #142950, #63977, #129208, #21172, #65428, #29894, #96555, #119053, #109604, #118330, #140793, #41491, #19033, #107464, #8127, #63297, #52368, #85699, #129945, #24036, #111761, #56710, #88, #58133, #66832, #1525, #68295, #2238, #110297, #23289, #44391, #11690, #134233, #101574, #100870, #46550, #124061, #79168, #135655, #13124, #24736, #90739, #34203, #45807, #89984, #36344, #34926, #134966, #100177, #35663, #55979, #67570, #79889, #68983, #826, #102330, #12427, #113162, #21882, #112471, #13835, #133514, #132828, #2978, #57395, #66132, #123372, #10975, #55243, #88598, #47271, #91443, #99422, #33513, #77712, #80573, #121889, #22563, #45114, #111011, #89290, #78420, #122618, #60994, #16718, #3660, #50783, #60253, #25439 ) ),
 .UNSPECIFIED., .F., .F., .F. ) 
 B_SPLINE_SURFACE_WITH_KNOTS ( ( 2, 2 ),
 ( 3, 2, 2, 2, 2, 2, 2, 2, 2, 2, 2, 2, 2, 2, 2, 2, 2, 2, 2, 2, 2, 2, 2, 2, 2, 2, 2, 2, 2, 2, 2, 2, 2, 2, 2, 2, 2, 2, 2, 2, 2, 2, 2, 2, 2, 2, 2, 2, 2, 2, 2, 2, 2, 2, 2, 2, 2, 2, 2, 2, 2, 2, 2, 2, 2, 2, 2, 2, 2, 2, 2, 2, 2, 2, 2, 2, 2, 2, 2, 2, 2, 2, 2, 2, 2, 2, 2, 2, 2, 2, 2, 2, 2, 2, 2, 2, 2, 2, 2, 2, 2, 2, 2, 2, 2, 2, 2, 2, 2, 2, 2, 2, 2, 2, 2, 2, 2, 2, 2, 2, 3 ),
 ( 0.000000000000000000, 1.000000000000000000 ),
 ( 0.000000000000000000, 0.008333333333333333218, 0.01666666666666666644, 0.02500000000000000139, 0.03333333333333333287, 0.04166666666666666435, 0.05000000000000000278, 0.05833333333333333426, 0.06666666666666666574, 0.07499999999999999722, 0.08333333333333332871, 0.09166666666666666019, 0.1000000000000000056, 0.1083333333333333370, 0.1166666666666666685, 0.1250000000000000000, 0.1333333333333333315, 0.1416666666666666630, 0.1499999999999999944, 0.1583333333333333259, 0.1666666666666666574, 0.1749999999999999889, 0.1833333333333333204, 0.1916666666666666796, 0.2000000000000000111, 0.2083333333333333426, 0.2166666666666666741, 0.2250000000000000056, 0.2333333333333333370, 0.2416666666666666685, 0.2500000000000000000, 0.2583333333333333592, 0.2666666666666666630, 0.2750000000000000222, 0.2833333333333333259, 0.2916666666666666852, 0.2999999999999999889, 0.3083333333333333481, 0.3166666666666666519, 0.3250000000000000111, 0.3333333333333333148, 0.3416666666666666741, 0.3499999999999999778, 0.3583333333333333370, 0.3666666666666666408, 0.3750000000000000000, 0.3833333333333333592, 0.3916666666666666630, 0.4000000000000000222, 0.4083333333333333259, 0.4166666666666666852, 0.4249999999999999889, 0.4333333333333333481, 0.4416666666666666519, 0.4500000000000000111, 0.4583333333333333148, 0.4666666666666666741, 0.4749999999999999778, 0.4833333333333333370, 0.4916666666666666408, 0.5000000000000000000, 0.5083333333333333037, 0.5166666666666667185, 0.5250000000000000222, 0.5333333333333333259, 0.5416666666666666297, 0.5500000000000000444, 0.5583333333333333481, 0.5666666666666666519, 0.5749999999999999556, 0.5833333333333333703, 0.5916666666666666741, 0.5999999999999999778, 0.6083333333333332815, 0.6166666666666666963, 0.6250000000000000000, 0.6333333333333333037, 0.6416666666666667185, 0.6500000000000000222, 0.6583333333333333259, 0.6666666666666666297, 0.6750000000000000444, 0.6833333333333333481, 0.6916666666666666519, 0.6999999999999999556, 0.7083333333333333703, 0.7166666666666666741, 0.7249999999999999778, 0.7333333333333332815, 0.7416666666666666963, 0.7500000000000000000, 0.7583333333333333037, 0.7666666666666667185, 0.7750000000000000222, 0.7833333333333333259, 0.7916666666666666297, 0.8000000000000000444, 0.8083333333333333481, 0.8166666666666666519, 0.8249999999999999556, 0.8333333333333333703, 0.8416666666666666741, 0.8499999999999999778, 0.8583333333333332815, 0.8666666666666666963, 0.8750000000000000000, 0.8833333333333333037, 0.8916666666666667185, 0.9000000000000000222, 0.9083333333333333259, 0.9166666666666666297, 0.9250000000000000444, 0.9333333333333333481, 0.9416666666666666519, 0.9499999999999999556, 0.9583333333333333703, 0.9666666666666666741, 0.9749999999999999778, 0.9833333333333332815, 0.9916666666666666963, 1.000000000000000000 ),
 .UNSPECIFIED. ) 
 GEOMETRIC_REPRESENTATION_ITEM ( )  RATIONAL_B_SPLINE_SURFACE ( (
 ( 1.000000000000000000, 0.9659258262890683122, 1.000000000000000000, 0.9659258262890683122, 1.000000000000000000, 0.9659258262890683122, 1.000000000000000000, 0.9659258262890683122, 1.000000000000000000, 0.9659258262890683122, 1.000000000000000000, 0.9659258262890683122, 1.000000000000000000, 0.9659258262890683122, 1.000000000000000000, 0.9659258262890683122, 1.000000000000000000, 0.9659258262890683122, 1.000000000000000000, 0.9659258262890683122, 1.000000000000000000, 0.9659258262890683122, 1.000000000000000000, 0.9659258262890683122, 1.000000000000000000, 0.9659258262890683122, 1.000000000000000000, 0.9659258262890683122, 1.000000000000000000, 0.9659258262890683122, 1.000000000000000000, 0.9659258262890683122, 1.000000000000000000, 0.9659258262890683122, 1.000000000000000000, 0.9659258262890683122, 1.000000000000000000, 0.9659258262890683122, 1.000000000000000000, 0.9659258262890683122, 1.000000000000000000, 0.9659258262890683122, 1.000000000000000000, 0.9659258262890683122, 1.000000000000000000, 0.9659258262890683122, 1.000000000000000000, 0.9659258262890683122, 1.000000000000000000, 0.9659258262890683122, 1.000000000000000000, 0.9659258262890683122, 1.000000000000000000, 0.9659258262890683122, 1.000000000000000000, 0.9659258262890683122, 1.000000000000000000, 0.9659258262890683122, 1.000000000000000000, 0.9659258262890683122, 1.000000000000000000, 0.9659258262890683122, 1.000000000000000000, 0.9659258262890683122, 1.000000000000000000, 0.9659258262890683122, 1.000000000000000000, 0.9659258262890683122, 1.000000000000000000, 0.9659258262890683122, 1.000000000000000000, 0.9659258262890683122, 1.000000000000000000, 0.9659258262890683122, 1.000000000000000000, 0.9659258262890683122, 1.000000000000000000, 0.9659258262890683122, 1.000000000000000000, 0.9659258262890683122, 1.000000000000000000, 0.9659258262890683122, 1.000000000000000000, 0.9659258262890683122, 1.000000000000000000, 0.9659258262890683122, 1.000000000000000000, 0.9659258262890683122, 1.000000000000000000, 0.9659258262890683122, 1.000000000000000000, 0.9659258262890683122, 1.000000000000000000, 0.9659258262890683122, 1.000000000000000000, 0.9659258262890683122, 1.000000000000000000, 0.9659258262890683122, 1.000000000000000000, 0.9659258262890683122, 1.000000000000000000, 0.9659258262890683122, 1.000000000000000000, 0.9659258262890683122, 1.000000000000000000, 0.9659258262890683122, 1.000000000000000000, 0.9659258262890683122, 1.000000000000000000, 0.9659258262890683122, 1.000000000000000000, 0.9659258262890683122, 1.000000000000000000, 0.9659258262890683122, 1.000000000000000000, 0.9659258262890683122, 1.000000000000000000, 0.9659258262890683122, 1.000000000000000000, 0.9659258262890683122, 1.000000000000000000, 0.9659258262890683122, 1.000000000000000000, 0.9659258262890683122, 1.000000000000000000, 0.9659258262890683122, 1.000000000000000000, 0.9659258262890683122, 1.000000000000000000, 0.9659258262890683122, 1.000000000000000000, 0.9659258262890683122, 1.000000000000000000, 0.9659258262890683122, 1.000000000000000000, 0.9659258262890683122, 1.000000000000000000, 0.9659258262890683122, 1.000000000000000000, 0.9659258262890683122, 1.000000000000000000, 0.9659258262890683122, 1.000000000000000000, 0.9659258262890683122, 1.000000000000000000, 0.9659258262890683122, 1.000000000000000000, 0.9659258262890683122, 1.000000000000000000, 0.9659258262890683122, 1.000000000000000000, 0.9659258262890683122, 1.000000000000000000, 0.9659258262890683122, 1.000000000000000000, 0.9659258262890683122, 1.000000000000000000, 0.9659258262890683122, 1.000000000000000000, 0.9659258262890683122, 1.000000000000000000, 0.9659258262890683122, 1.000000000000000000, 0.9659258262890683122, 1.000000000000000000, 0.9659258262890683122, 1.000000000000000000, 0.9659258262890683122, 1.000000000000000000, 0.9659258262890683122, 1.000000000000000000, 0.9659258262890683122, 1.000000000000000000, 0.9659258262890683122, 1.000000000000000000, 0.9659258262890683122, 1.000000000000000000, 0.9659258262890683122, 1.000000000000000000, 0.9659258262890683122, 1.000000000000000000, 0.9659258262890683122, 1.000000000000000000, 0.9659258262890683122, 1.000000000000000000, 0.9659258262890683122, 1.000000000000000000, 0.9659258262890683122, 1.000000000000000000, 0.9659258262890683122, 1.000000000000000000, 0.9659258262890683122, 1.000000000000000000, 0.9659258262890683122, 1.000000000000000000, 0.9659258262890683122, 1.000000000000000000, 0.9659258262890683122, 1.000000000000000000, 0.9659258262890683122, 1.000000000000000000, 0.9659258262890683122, 1.000000000000000000, 0.9659258262890683122, 1.000000000000000000, 0.9659258262890683122, 1.000000000000000000, 0.9659258262890683122, 1.000000000000000000, 0.9659258262890683122, 1.000000000000000000, 0.9659258262890683122, 1.000000000000000000, 0.9659258262890683122, 1.000000000000000000, 0.9659258262890683122, 1.000000000000000000, 0.9659258262890683122, 1.000000000000000000, 0.9659258262890683122, 1.000000000000000000, 0.9659258262890683122, 1.000000000000000000, 0.9659258262890683122, 1.000000000000000000, 0.9659258262890683122, 1.000000000000000000, 0.9659258262890683122, 1.000000000000000000, 0.9659258262890683122, 1.000000000000000000, 0.9659258262890683122, 1.000000000000000000, 0.9659258262890683122, 1.000000000000000000, 0.9659258262890683122, 1.000000000000000000, 0.9659258262890683122, 1.000000000000000000, 0.9659258262890683122, 1.000000000000000000),
 ( 1.000000000000000000, 0.9659258262890683122, 1.000000000000000000, 0.9659258262890683122, 1.000000000000000000, 0.9659258262890683122, 1.000000000000000000, 0.9659258262890683122, 1.000000000000000000, 0.9659258262890683122, 1.000000000000000000, 0.9659258262890683122, 1.000000000000000000, 0.9659258262890683122, 1.000000000000000000, 0.9659258262890683122, 1.000000000000000000, 0.9659258262890683122, 1.000000000000000000, 0.9659258262890683122, 1.000000000000000000, 0.9659258262890683122, 1.000000000000000000, 0.9659258262890683122, 1.000000000000000000, 0.9659258262890683122, 1.000000000000000000, 0.9659258262890683122, 1.000000000000000000, 0.9659258262890683122, 1.000000000000000000, 0.9659258262890683122, 1.000000000000000000, 0.9659258262890683122, 1.000000000000000000, 0.9659258262890683122, 1.000000000000000000, 0.9659258262890683122, 1.000000000000000000, 0.9659258262890683122, 1.000000000000000000, 0.9659258262890683122, 1.000000000000000000, 0.9659258262890683122, 1.000000000000000000, 0.9659258262890683122, 1.000000000000000000, 0.9659258262890683122, 1.000000000000000000, 0.9659258262890683122, 1.000000000000000000, 0.9659258262890683122, 1.000000000000000000, 0.9659258262890683122, 1.000000000000000000, 0.9659258262890683122, 1.000000000000000000, 0.9659258262890683122, 1.000000000000000000, 0.9659258262890683122, 1.000000000000000000, 0.9659258262890683122, 1.000000000000000000, 0.9659258262890683122, 1.000000000000000000, 0.9659258262890683122, 1.000000000000000000, 0.9659258262890683122, 1.000000000000000000, 0.9659258262890683122, 1.000000000000000000, 0.9659258262890683122, 1.000000000000000000, 0.9659258262890683122, 1.000000000000000000, 0.9659258262890683122, 1.000000000000000000, 0.9659258262890683122, 1.000000000000000000, 0.9659258262890683122, 1.000000000000000000, 0.9659258262890683122, 1.000000000000000000, 0.9659258262890683122, 1.000000000000000000, 0.9659258262890683122, 1.000000000000000000, 0.9659258262890683122, 1.000000000000000000, 0.9659258262890683122, 1.000000000000000000, 0.9659258262890683122, 1.000000000000000000, 0.9659258262890683122, 1.000000000000000000, 0.9659258262890683122, 1.000000000000000000, 0.9659258262890683122, 1.000000000000000000, 0.9659258262890683122, 1.000000000000000000, 0.9659258262890683122, 1.000000000000000000, 0.9659258262890683122, 1.000000000000000000, 0.9659258262890683122, 1.000000000000000000, 0.9659258262890683122, 1.000000000000000000, 0.9659258262890683122, 1.000000000000000000, 0.9659258262890683122, 1.000000000000000000, 0.9659258262890683122, 1.000000000000000000, 0.9659258262890683122, 1.000000000000000000, 0.9659258262890683122, 1.000000000000000000, 0.9659258262890683122, 1.000000000000000000, 0.9659258262890683122, 1.000000000000000000, 0.9659258262890683122, 1.000000000000000000, 0.9659258262890683122, 1.000000000000000000, 0.9659258262890683122, 1.000000000000000000, 0.9659258262890683122, 1.000000000000000000, 0.9659258262890683122, 1.000000000000000000, 0.9659258262890683122, 1.000000000000000000, 0.9659258262890683122, 1.000000000000000000, 0.9659258262890683122, 1.000000000000000000, 0.9659258262890683122, 1.000000000000000000, 0.9659258262890683122, 1.000000000000000000, 0.9659258262890683122, 1.000000000000000000, 0.9659258262890683122, 1.000000000000000000, 0.9659258262890683122, 1.000000000000000000, 0.9659258262890683122, 1.000000000000000000, 0.9659258262890683122, 1.000000000000000000, 0.9659258262890683122, 1.000000000000000000, 0.9659258262890683122, 1.000000000000000000, 0.9659258262890683122, 1.000000000000000000, 0.9659258262890683122, 1.000000000000000000, 0.9659258262890683122, 1.000000000000000000, 0.9659258262890683122, 1.000000000000000000, 0.9659258262890683122, 1.000000000000000000, 0.9659258262890683122, 1.000000000000000000, 0.9659258262890683122, 1.000000000000000000, 0.9659258262890683122, 1.000000000000000000, 0.9659258262890683122, 1.000000000000000000, 0.9659258262890683122, 1.000000000000000000, 0.9659258262890683122, 1.000000000000000000, 0.9659258262890683122, 1.000000000000000000, 0.9659258262890683122, 1.000000000000000000, 0.9659258262890683122, 1.000000000000000000, 0.9659258262890683122, 1.000000000000000000, 0.9659258262890683122, 1.000000000000000000, 0.9659258262890683122, 1.000000000000000000, 0.9659258262890683122, 1.000000000000000000, 0.9659258262890683122, 1.000000000000000000, 0.9659258262890683122, 1.000000000000000000, 0.9659258262890683122, 1.000000000000000000, 0.9659258262890683122, 1.000000000000000000, 0.9659258262890683122, 1.000000000000000000, 0.9659258262890683122, 1.000000000000000000, 0.9659258262890683122, 1.000000000000000000, 0.9659258262890683122, 1.000000000000000000, 0.9659258262890683122, 1.000000000000000000, 0.9659258262890683122, 1.000000000000000000, 0.9659258262890683122, 1.000000000000000000, 0.9659258262890683122, 1.000000000000000000, 0.9659258262890683122, 1.000000000000000000, 0.9659258262890683122, 1.000000000000000000, 0.9659258262890683122, 1.000000000000000000, 0.9659258262890683122, 1.000000000000000000, 0.9659258262890683122, 1.000000000000000000, 0.9659258262890683122, 1.000000000000000000, 0.9659258262890683122, 1.000000000000000000, 0.9659258262890683122, 1.000000000000000000, 0.9659258262890683122, 1.000000000000000000, 0.9659258262890683122, 1.000000000000000000, 0.9659258262890683122, 1.000000000000000000, 0.9659258262890683122, 1.000000000000000000) ) ) 
 REPRESENTATION_ITEM ( '' )  SURFACE ( )  );
#74483=MECHANICAL_DESIGN_GEOMETRIC_PRESENTATION_REPRESENTATION('',(#129692),#99919);
#74510=CARTESIAN_POINT ( 'NONE',  ( 2.999999999999999112, 1.399999999999987699, -20.40202195861970580 ) ) ;
#74514=ORIENTED_EDGE ( 'NONE', *, *, #60106, .T. ) ;
#74521=( NAMED_UNIT ( * ) SI_UNIT ( $, .STERADIAN. ) SOLID_ANGLE_UNIT ( ) );
#74525=CARTESIAN_POINT ( 'NONE',  ( -0.02126352523144730070, -5.808823158059033709, 5.808823158059035485 ) ) ;
#74556=CYLINDRICAL_SURFACE ( 'NONE', #121645, 3.999999999999989786 ) ;
#74562=CARTESIAN_POINT ( 'NONE',  ( 4.812499999999999112, -4.461849672132299993, -4.461849672132299105 ) ) ;
#74563=CARTESIAN_POINT ( 'NONE',  ( 19.52040314143522437, 7.934999999999988951, -2.126176841940961904 ) ) ;
#74579=COLOUR_RGB ( '', 0.09019608, 0.27058824, 0.51372549) ;
#74595=CARTESIAN_POINT ( 'NONE',  ( 57.42758194782751247, -45.84254607569047124, 35.55177538329026277 ) ) ;
#74604=CARTESIAN_POINT ( 'NONE',  ( 124.4403572661728390, -44.90675832754093477, 35.11767176072991248 ) ) ;
#74614=LINE ( 'NONE', #31107, #105477 ) ;
#74618=ORIENTED_EDGE ( 'NONE', *, *, #5682, .F. ) ;
#74623=CARTESIAN_POINT ( 'NONE',  ( 14.35873647476855375, 5.808823158059031044, -5.808823158059037262 ) ) ;
#74641=CYLINDRICAL_SURFACE ( 'NONE', #94681, 6.094999999999989093 ) ;
#74667=DIRECTION ( 'NONE',  ( 1.000000000000000000, 0.000000000000000000, 0.000000000000000000 ) ) ;
#74702=CARTESIAN_POINT ( 'NONE',  ( 14.35873647476855197, 5.808823158059031044, -5.808823158059038150 ) ) ;
#74710=LINE ( 'NONE', #118151, #38077 ) ;
#74728=CARTESIAN_POINT ( 'NONE',  ( 0.3394530118782473349, -51.90335959434331414, -39.28179725402795697 ) ) ;
#74735=CARTESIAN_POINT ( 'NONE',  ( 156.1500000000000057, -49.14999999999999147, 53.92499999999997584 ) ) ;
#74776=DIRECTION ( 'NONE',  ( -8.673617379884025611E-16, 0.000000000000000000, 1.000000000000000000 ) ) ;
#74794=DIRECTION ( 'NONE',  ( 0.000000000000000000, 0.000000000000000000, 1.000000000000000000 ) ) ;
#74851=VERTEX_POINT ( 'NONE', #20475 ) ;
#74861=VERTEX_POINT ( 'NONE', #129243 ) ;
#74878=CARTESIAN_POINT ( 'NONE',  ( 18.15040314143522338, 7.934999999999989839, -2.126176841940961904 ) ) ;
#74885=LINE ( 'NONE', #96562, #44930 ) ;
#74896=DIRECTION ( 'NONE',  ( 0.000000000000000000, 1.000000000000000000, 5.782411586589357244E-15 ) ) ;
#74900=DIRECTION ( 'NONE',  ( -0.000000000000000000, 0.000000000000000000, 1.000000000000000000 ) ) ;
#74903=CARTESIAN_POINT ( 'NONE',  ( 3.645833333333334370, -1.633150327867695095, 6.094999999999987317 ) ) ;
#74911=CARTESIAN_POINT ( 'NONE',  ( 10.04123647476855297, 0.000000000000000000, 7.934999999999990727 ) ) ;
#74917=SURFACE_STYLE_USAGE ( .BOTH. , #10323 ) ;
#74943=SURFACE_STYLE_USAGE ( .BOTH. , #49084 ) ;
#74948=VECTOR ( 'NONE', #93385, 1000.000000000000000 ) ;
#74958=( LENGTH_UNIT ( ) NAMED_UNIT ( * ) SI_UNIT ( .MILLI., .METRE. ) );
#74978=CARTESIAN_POINT ( 'NONE',  ( 14.72916666666666607, -6.094999999999989093, 1.633150327867691542 ) ) ;
#74979=CARTESIAN_POINT ( 'NONE',  ( 52.26932219902318622, -52.14999999999999147, -40.92499999999998295 ) ) ;
#74981=DIRECTION ( 'NONE',  ( 0.000000000000000000, 0.000000000000000000, -1.000000000000000000 ) ) ;
#75045=CARTESIAN_POINT ( 'NONE',  ( 3.500000000000000444, 0.000000000000000000, 6.094999999999989981 ) ) ;
#75048=CARTESIAN_POINT ( 'NONE',  ( 28.04580628287044064, 5.278424836066143655, -3.047499999999997655 ) ) ;
#75070=CARTESIAN_POINT ( 'NONE',  ( 28.00000000000002487, -57.14999999999999147, -34.92499999999976978 ) ) ;
#75093=CARTESIAN_POINT ( 'NONE',  ( 0.6686314397420025646, -52.14999999947626463, -41.03936837847411567 ) ) ;
#75114=PRESENTATION_STYLE_ASSIGNMENT (( #139663 ) ) ;
#75128=CARTESIAN_POINT ( 'NONE',  ( 29.75000000000000355, -7.464222240803106570E-16, -6.094999999999989981 ) ) ;
#75178=CARTESIAN_POINT ( 'NONE',  ( 181.0474453055293793, -48.63825160239814238, 38.47250499286696623 ) ) ;
#75213=COLOUR_RGB ( '', 0.66274510, 0.83137255, 0.94901961) ;
#75214=FILL_AREA_STYLE_COLOUR ( '', #21826 ) ;
#75238=CARTESIAN_POINT ( 'NONE',  ( 3.730677800976790248, -49.14999999999999147, 40.92499999999998295 ) ) ;
#75241=( GEOMETRIC_REPRESENTATION_CONTEXT ( 3 ) GLOBAL_UNCERTAINTY_ASSIGNED_CONTEXT ( ( #55109 ) ) GLOBAL_UNIT_ASSIGNED_CONTEXT ( ( #82033, #124780, #92856 ) ) REPRESENTATION_CONTEXT ( 'NONE', 'WORKASPACE' ) );
#75242=CARTESIAN_POINT ( 'NONE',  ( 33.17123647476855552, 0.000000000000000000, 7.934999999999990727 ) ) ;
#75282=CARTESIAN_POINT ( 'NONE',  ( 6.270833333333333925, 6.094999999999991758, 1.633150327867687102 ) ) ;
#75283=CARTESIAN_POINT ( 'NONE',  ( 21.70790314143522082, -6.871911579029513106, -3.967499999999993587 ) ) ;
#75307=CARTESIAN_POINT ( 'NONE',  ( 57.34909574878652450, -49.32595796886462836, 36.54674188582600181 ) ) ;
#75334=CARTESIAN_POINT ( 'NONE',  ( 19.90040314143522338, -7.934999999999988951, 2.126176841940957907 ) ) ;
#75348=CARTESIAN_POINT ( 'NONE',  ( 17.64583333333333215, -1.633150327867690210, 6.094999999999989981 ) ) ;
#75365=ORIENTED_EDGE ( 'NONE', *, *, #28993, .F. ) ;
#75398=CARTESIAN_POINT ( 'NONE',  ( 7.942069808101886785, 7.934999999999993392, 2.126176841940951689 ) ) ;
#75469=SURFACE_STYLE_FILL_AREA ( #41391 ) ;
#75508=VERTEX_POINT ( 'NONE', #68675 ) ;
#75511=ADVANCED_FACE ( 'NONE', ( #36047 ), #69498, .T. ) ;
#75516=MECHANICAL_DESIGN_GEOMETRIC_PRESENTATION_REPRESENTATION('',(#38462),#26860);
#75570=CARTESIAN_POINT ( 'NONE',  ( 19.60873647476855197, -5.808823158059033709, 5.808823158059035485 ) ) ;
#75585=CARTESIAN_POINT ( 'NONE',  ( 26.40000000000000568, -17.48000000000005016, -12.70000000000045404 ) ) ;
#75638=AXIS2_PLACEMENT_3D ( 'NONE', #142887, #20, #44315 ) ;
#75657=( NAMED_UNIT ( * ) SI_UNIT ( $, .STERADIAN. ) SOLID_ANGLE_UNIT ( ) );
#75724=CYLINDRICAL_SURFACE ( 'NONE', #107065, 6.094999999999989093 ) ;
#75731=VERTEX_POINT ( 'NONE', #65683 ) ;
#75740=CARTESIAN_POINT ( 'NONE',  ( 25.12913961620377279, 5.278424836066147208, 3.047499999999990550 ) ) ;
#75788=( LENGTH_UNIT ( ) NAMED_UNIT ( * ) SI_UNIT ( .MILLI., .METRE. ) );
#75793=LINE ( 'NONE', #64917, #9371 ) ;
#75795=ORIENTED_EDGE ( 'NONE', *, *, #125963, .T. ) ;
#75823=DIRECTION ( 'NONE',  ( 0.000000000000000000, -1.000000000000000000, 0.000000000000000000 ) ) ;
#75836=( GEOMETRIC_REPRESENTATION_CONTEXT ( 3 ) GLOBAL_UNCERTAINTY_ASSIGNED_CONTEXT ( ( #28567 ) ) GLOBAL_UNIT_ASSIGNED_CONTEXT ( ( #62873, #63596, #140401 ) ) REPRESENTATION_CONTEXT ( 'NONE', 'WORKASPACE' ) );
#75882=CARTESIAN_POINT ( 'NONE',  ( 184.1499999999998067, -49.85820393249939286, 34.92500000000001847 ) ) ;
#75892=ORIENTED_EDGE ( 'NONE', *, *, #130295, .F. ) ;
#75902=CARTESIAN_POINT ( 'NONE',  ( -1.704193717129561136, -5.278424836066144543, 3.047499999999995879 ) ) ;
#75933=CARTESIAN_POINT ( 'NONE',  ( 11.79123647476855297, -9.717572351234235426E-16, -7.934999999999990727 ) ) ;
#75968=CARTESIAN_POINT ( 'NONE',  ( 27.99999999999999645, -49.14999999999999147, -49.92499999999968452 ) ) ;
#75977=CARTESIAN_POINT ( 'NONE',  ( 5.687500000000000000, 4.461849672132297329, -4.461849672132302658 ) ) ;
#75978=CARTESIAN_POINT ( 'NONE',  ( 17.77040314143522082, -7.934999999999988951, 2.126176841940957907 ) ) ;
#75980=FILL_AREA_STYLE_COLOUR ( '', #104494 ) ;
#75983=STYLED_ITEM ( 'NONE', ( #83832 ), #37829 ) ;
#75991=CARTESIAN_POINT ( 'NONE',  ( 129.2310344399266739, -47.51495700085919083, -36.79359617903136837 ) ) ;
#75997=DIRECTION ( 'NONE',  ( -1.000000000000000000, -0.000000000000000000, -0.000000000000000000 ) ) ;
#76002=CARTESIAN_POINT ( 'NONE',  ( 28.00000000000002487, -49.14999999999999147, -34.92499999999976978 ) ) ;
#76023=AXIS2_PLACEMENT_3D ( 'NONE', #40417, #26662, #16468 ) ;
#76031=VECTOR ( 'NONE', #34391, 1000.000000000000000 ) ;
#76034=CARTESIAN_POINT ( 'NONE',  ( 16.40040314143521982, -7.934999999999988951, 2.126176841940957907 ) ) ;
#76053=DIRECTION ( 'NONE',  ( -1.000000000000000000, -0.000000000000000000, -0.000000000000000000 ) ) ;
#76060=SURFACE_STYLE_USAGE ( .BOTH. , #107930 ) ;
#76105=CARTESIAN_POINT ( 'NONE',  ( 21.06706980810188412, 2.126176841940952134, -7.934999999999993392 ) ) ;
#76110=CARTESIAN_POINT ( 'NONE',  ( 52.40027281130056735, -49.14999999999999147, -40.57187971032006857 ) ) ;
#76131=AXIS2_PLACEMENT_3D ( 'NONE', #27714, #116153, #118276 ) ;
#76141=( GEOMETRIC_REPRESENTATION_CONTEXT ( 3 ) GLOBAL_UNCERTAINTY_ASSIGNED_CONTEXT ( ( #78095 ) ) GLOBAL_UNIT_ASSIGNED_CONTEXT ( ( #105656, #50594, #136886 ) ) REPRESENTATION_CONTEXT ( 'NONE', 'WORKASPACE' ) );
#76148=CARTESIAN_POINT ( 'NONE',  ( 0.1600000000000010858, -4.972023319592707047, -6.193256324377186317 ) ) ;
#76151=PRESENTATION_STYLE_ASSIGNMENT (( #31928 ) ) ;
#76160=EDGE_LOOP ( 'NONE', ( #38548, #49740, #109969, #20041 ) ) ;
#76182=MECHANICAL_DESIGN_GEOMETRIC_PRESENTATION_REPRESENTATION('',(#140934),#101614);
#76212=DIRECTION ( 'NONE',  ( 0.000000000000000000, -1.000000000000000000, 0.000000000000000000 ) ) ;
#76255=CARTESIAN_POINT ( 'NONE',  ( 151.4000000000000057, -16.48000000000005016, 0.000000000000000000 ) ) ;
#76287=CARTESIAN_POINT ( 'NONE',  ( 15.37956980810188767, 3.967499999999998916, 6.871911579029510442 ) ) ;
#76294=STYLED_ITEM ( 'NONE', ( #71319 ), #20929 ) ;
#76328=ORIENTED_EDGE ( 'NONE', *, *, #21381, .T. ) ;
#76369=FILL_AREA_STYLE_COLOUR ( '', #119681 ) ;
#76402=DIRECTION ( 'NONE',  ( 0.000000000000000000, 0.000000000000000000, -1.000000000000000000 ) ) ;
#76409=ORIENTED_EDGE ( 'NONE', *, *, #117555, .F. ) ;
#76441=DIRECTION ( 'NONE',  ( 0.000000000000000000, 1.000000000000000000, 1.286409696682840916E-16 ) ) ;
#76464=CARTESIAN_POINT ( 'NONE',  ( 21.62913961620377279, 5.278424836066147208, 3.047499999999990550 ) ) ;
#76501=ORIENTED_EDGE ( 'NONE', *, *, #8540, .T. ) ;
#76539=CARTESIAN_POINT ( 'NONE',  ( 15.50413961620377279, -3.047499999999994547, 5.278424836066145431 ) ) ;
#76565=CARTESIAN_POINT ( 'NONE',  ( 55.45418156660456788, -52.10373894832328290, 40.45955814675563289 ) ) ;
#76618=CARTESIAN_POINT ( 'NONE',  ( 183.4386084925739340, -49.19295221407111995, 41.21232802153470942 ) ) ;
#76629=DIRECTION ( 'NONE',  ( 6.895928203464619851E-15, 0.6666666666666692942, 0.7453559924999275665 ) ) ;
#76641=CARTESIAN_POINT ( 'NONE',  ( 0.1916396162037724282, 6.094999999999988205, -1.633150327867694651 ) ) ;
#76651=LINE ( 'NONE', #21533, #26683 ) ;
#76672=CARTESIAN_POINT ( 'NONE',  ( 9.749569808101886892, 3.967499999999998916, 6.871911579029510442 ) ) ;
#76682=UNCERTAINTY_MEASURE_WITH_UNIT (LENGTH_MEASURE( 1.000000000000000082E-05 ), #58354, 'distance_accuracy_value', 'NONE');
#76706=FILL_AREA_STYLE ('',( #57094 ) ) ;
#76709=UNCERTAINTY_MEASURE_WITH_UNIT (LENGTH_MEASURE( 1.000000000000000082E-05 ), #90263, 'distance_accuracy_value', 'NONE');
#76710=ORIENTED_EDGE ( 'NONE', *, *, #49536, .F. ) ;
#76716=SURFACE_STYLE_USAGE ( .BOTH. , #32476 ) ;
#76720=CARTESIAN_POINT ( 'NONE',  ( 2.479166666666666963, 6.094999999999988205, -1.633150327867694651 ) ) ;
#76721=CARTESIAN_POINT ( 'NONE',  ( 15.58290314143522082, 3.967499999999992699, -6.871911579029513994 ) ) ;
#76726=ORIENTED_EDGE ( 'NONE', *, *, #110186, .T. ) ;
#76738=PRESENTATION_STYLE_ASSIGNMENT (( #108576 ) ) ;
#76751=ORIENTED_EDGE ( 'NONE', *, *, #43922, .T. ) ;
#76753=CARTESIAN_POINT ( 'NONE',  ( 126.2665610010944874, -48.52444309369082731, 36.09967824800328628 ) ) ;
#76772=EDGE_LOOP ( 'NONE', ( #74618, #104272 ) ) ;
#76778=CARTESIAN_POINT ( 'NONE',  ( 14.94206980810188590, 7.934999999999992504, 2.126176841940951689 ) ) ;
#76781=CARTESIAN_POINT ( 'NONE',  ( 159.7320121765528711, 26.96999999999993847, 34.92499999999998295 ) ) ;
#76795=CARTESIAN_POINT ( 'NONE',  ( 52.60764783923757193, -49.05583548141699879, 39.86617647058822200 ) ) ;
#76822=AXIS2_PLACEMENT_3D ( 'NONE', #130592, #74050, #118237 ) ;
#76848=CARTESIAN_POINT ( 'NONE',  ( 18.58790314143521982, 6.871911579029515771, 3.967499999999989146 ) ) ;
#76852=DIRECTION ( 'NONE',  ( 1.000000000000000000, 0.000000000000000000, -0.000000000000000000 ) ) ;
#76872=FILL_AREA_STYLE_COLOUR ( '', #21226 ) ;
#76876=ORIENTED_EDGE ( 'NONE', *, *, #43646, .T. ) ;
#76877=EDGE_CURVE ( 'NONE', #137404, #34663, #80472, .T. ) ;
#76893=LINE ( 'NONE', #97903, #87322 ) ;
#76935=EDGE_CURVE ( 'NONE', #81702, #81966, #135928, .T. ) ;
#76973=CIRCLE ( 'NONE', #111710, 3.000000000000000000 ) ;
#76974=DIRECTION ( 'NONE',  ( -1.000000000000000000, -0.000000000000000000, 0.000000000000000000 ) ) ;
#76993=DIRECTION ( 'NONE',  ( 0.000000000000000000, 0.000000000000000000, 1.000000000000000000 ) ) ;
#77011=CARTESIAN_POINT ( 'NONE',  ( 164.1998387378793893, 26.96999999999993491, -34.37854159432827572 ) ) ;
#77017=CARTESIAN_POINT ( 'NONE',  ( 19.17123647476855197, 0.000000000000000000, 7.934999999999990727 ) ) ;
#77033=CARTESIAN_POINT ( 'NONE',  ( 25.39999999999999858, 7.464222240803104598E-16, -6.094999999999989093 ) ) ;
#77059=STYLED_ITEM ( 'NONE', ( #16086 ), #68458 ) ;
#77062=VECTOR ( 'NONE', #119754, 1000.000000000000000 ) ;
#77069=VERTEX_POINT ( 'NONE', #46071 ) ;
#77108=DIRECTION ( 'NONE',  ( -1.000000000000000000, 0.000000000000000000, 0.000000000000000000 ) ) ;
#77120=CARTESIAN_POINT ( 'NONE',  ( 9.087472949537108491, -6.094999999999989981, 3.732111120401553285E-16 ) ) ;
#77149=( BOUNDED_CURVE ( )  B_SPLINE_CURVE ( 3, ( #100963, #1618, #112563, #101678 ),
 .UNSPECIFIED., .F., .F. ) 
 B_SPLINE_CURVE_WITH_KNOTS ( ( 4, 4 ),
 ( 4.712388980384689674, 6.283185307179586232 ),
 .UNSPECIFIED. ) 
 CURVE ( )  GEOMETRIC_REPRESENTATION_ITEM ( )  RATIONAL_B_SPLINE_CURVE ( ( 1.000000000000000000, 0.8047378541243649375, 0.8047378541243649375, 1.000000000000000000 ) ) 
 REPRESENTATION_ITEM ( '' )  );
#77161=ORIENTED_EDGE ( 'NONE', *, *, #128289, .F. ) ;
#77171=DIRECTION ( 'NONE',  ( -0.000000000000000000, -0.000000000000000000, -1.000000000000000000 ) ) ;
#77172=CARTESIAN_POINT ( 'NONE',  ( 52.60764783923757193, -52.00875322212550600, 39.33676470588235219 ) ) ;
#77190=CARTESIAN_POINT ( 'NONE',  ( 23.52497294953710849, -4.461849672132299993, -4.461849672132299105 ) ) ;
#77222=LINE ( 'NONE', #31548, #21634 ) ;
#77226=CARTESIAN_POINT ( 'NONE',  ( 26.40000000000000568, -16.48000000000005016, -33.92499999999998295 ) ) ;
#77239=FILL_AREA_STYLE_COLOUR ( '', #123858 ) ;
#77254=DIRECTION ( 'NONE',  ( -0.000000000000000000, 1.000000000000000000, -0.000000000000000000 ) ) ;
#77353=CARTESIAN_POINT ( 'NONE',  ( 2.000000000000256239, -6.019044215166783118, 0.9592349742722835471 ) ) ;
#77367=CARTESIAN_POINT ( 'NONE',  ( 0.04580628287043911340, 5.278424836066143655, -3.047499999999997655 ) ) ;
#77371=DIRECTION ( 'NONE',  ( 0.000000000000000000, 0.000000000000000000, 1.000000000000000000 ) ) ;
#77388=CARTESIAN_POINT ( 'NONE',  ( 52.51203195997707951, -49.11957940092399610, 40.22172306649563467 ) ) ;
#77392=VECTOR ( 'NONE', #11040, 1000.000000000000000 ) ;
#77393=CARTESIAN_POINT ( 'NONE',  ( 13.97873647476855119, -5.808823158059033709, 5.808823158059035485 ) ) ;
#77402=SURFACE_STYLE_FILL_AREA ( #65822 ) ;
#77409=COLOUR_RGB ( '', 0.31764706, 0.68627451, 0.89019608) ;
#77419=CARTESIAN_POINT ( 'NONE',  ( 17.83747294953710494, 6.094999999999989981, -1.119633336120465690E-15 ) ) ;
#77425=PRESENTATION_STYLE_ASSIGNMENT (( #134650 ) ) ;
#77433=SURFACE_STYLE_USAGE ( .BOTH. , #67999 ) ;
#77435=SURFACE_SIDE_STYLE ('',( #133233 ) ) ;
#77438=CARTESIAN_POINT ( 'NONE',  ( 12.10416666666666607, -1.633150327867691987, -6.094999999999989093 ) ) ;
#77439=CARTESIAN_POINT ( 'NONE',  ( 18.93706980810188867, 2.126176841940952134, -7.934999999999992504 ) ) ;
#77451=CARTESIAN_POINT ( 'NONE',  ( 128.0481121284643962, -51.19676978474259954, -38.21513923099703902 ) ) ;
#77457=( NAMED_UNIT ( * ) SI_UNIT ( $, .STERADIAN. ) SOLID_ANGLE_UNIT ( ) );
#77467=ORIENTED_EDGE ( 'NONE', *, *, #115028, .F. ) ;
#77488=CARTESIAN_POINT ( 'NONE',  ( 19.46290314143521982, -3.967499999999994476, 6.871911579029513106 ) ) ;
#77513=FACE_OUTER_BOUND ( 'NONE', #117957, .T. ) ;
#77541=ORIENTED_EDGE ( 'NONE', *, *, #104332, .T. ) ;
#77555=CARTESIAN_POINT ( 'NONE',  ( 16.98373647476855197, -5.808823158059035485, -5.808823158059033709 ) ) ;
#77594=COLOUR_RGB ( '', 0.72549020, 0.75294118, 0.79215686) ;
#77599=CARTESIAN_POINT ( 'NONE',  ( 17.18706980810188867, -2.126176841940956130, 7.934999999999991616 ) ) ;
#77614=ORIENTED_EDGE ( 'NONE', *, *, #136879, .F. ) ;
#77625=DIRECTION ( 'NONE',  ( -0.000000000000000000, 1.000000000000000000, 1.091707662666338270E-16 ) ) ;
#77639=CARTESIAN_POINT ( 'NONE',  ( 28.00000000000002487, -52.14999999999999147, -34.92499999999976978 ) ) ;
#77655=CARTESIAN_POINT ( 'NONE',  ( 122.6835989386367771, -49.14999999999999147, -40.92499999999998295 ) ) ;
#77668=FILL_AREA_STYLE ('',( #23987 ) ) ;
#77687=FILL_AREA_STYLE ('',( #10254 ) ) ;
#77691=CARTESIAN_POINT ( 'NONE',  ( 2.999999999999999112, -7.600000000000055600, -28.92499999999998650 ) ) ;
#77712=CARTESIAN_POINT ( 'NONE',  ( 31.12956980810189478, -3.967499999999998028, -6.871911579029511330 ) ) ;
#77719=EDGE_CURVE ( 'NONE', #14349, #36041, #121140, .T. ) ;
#77723=EDGE_LOOP ( 'NONE', ( #64871, #41976, #75365, #66570 ) ) ;
#77746=DIRECTION ( 'NONE',  ( 0.000000000000000000, -1.000000000000000000, 0.000000000000000000 ) ) ;
#77748=( BOUNDED_CURVE ( )  B_SPLINE_CURVE ( 2, ( #4220, #26757, #76539, #12666, #21427, #34438, #23557, #87403, #56239, #33052, #133755, #77953, #22802 ),
 .UNSPECIFIED., .F., .T. ) 
 B_SPLINE_CURVE_WITH_KNOTS ( ( 3, 2, 2, 2, 2, 2, 3 ),
 ( 0.5000000000000000000, 0.5083333333333333037, 0.5166666666666667185, 0.5250000000000001332, 0.5333333333333334370, 0.5416666666666667407, 0.5500000000000001554 ),
 .UNSPECIFIED. ) 
 CURVE ( )  GEOMETRIC_REPRESENTATION_ITEM ( )  RATIONAL_B_SPLINE_CURVE ( ( 1.000000000000000000, 0.9659258262890683122, 1.000000000000000000, 0.9659258262890683122, 1.000000000000000000, 0.9659258262890683122, 1.000000000000000000, 0.9659258262890683122, 1.000000000000000000, 0.9659258262890683122, 1.000000000000000000, 0.9659258262890678681, 1.000000000000000444 ) ) 
 REPRESENTATION_ITEM ( '' )  );
#77771=CARTESIAN_POINT ( 'NONE',  ( 25.40000000000000568, 3.739651257385445238, 5.035049619000475651 ) ) ;
#77800=CARTESIAN_POINT ( 'NONE',  ( 0.1600000000000028066, 0.5691893105020771060, -7.934999999999987175 ) ) ;
#77812=( NAMED_UNIT ( * ) SI_UNIT ( $, .STERADIAN. ) SOLID_ANGLE_UNIT ( ) );
#77853=ADVANCED_FACE ( 'NONE', ( #114987 ), #82414, .T. ) ;
#77871=ORIENTED_EDGE ( 'NONE', *, *, #65246, .F. ) ;
#77874=CARTESIAN_POINT ( 'NONE',  ( 174.7500000000000000, 7.919999999999947526, 16.57230000000005532 ) ) ;
#77877=CARTESIAN_POINT ( 'NONE',  ( 30.52497294953710494, -4.461849672132299993, -4.461849672132299105 ) ) ;
#77888=LINE ( 'NONE', #22053, #130247 ) ;
#77899=CARTESIAN_POINT ( 'NONE',  ( 13.46247294953710494, -7.464222240803106570E-16, -6.094999999999989981 ) ) ;
#77900=DIRECTION ( 'NONE',  ( 0.000000000000000000, 0.000000000000000000, -1.000000000000000000 ) ) ;
#77931=FACE_OUTER_BOUND ( 'NONE', #32273, .T. ) ;
#77936=CARTESIAN_POINT ( 'NONE',  ( 61.46640106136307935, -49.14999999999999147, 40.92499999999998295 ) ) ;
#77949=CARTESIAN_POINT ( 'NONE',  ( 18.71247294953710494, 0.000000000000000000, 6.094999999999989981 ) ) ;
#77950=UNCERTAINTY_MEASURE_WITH_UNIT (LENGTH_MEASURE( 1.000000000000000082E-05 ), #117504, 'distance_accuracy_value', 'NONE');
#77953=CARTESIAN_POINT ( 'NONE',  ( 16.81663961620377279, -1.633150327867672447, -6.094999999999999751 ) ) ;
#77968=( BOUNDED_CURVE ( )  B_SPLINE_CURVE ( 3, ( #89306, #13140, #12442, #87874 ),
 .UNSPECIFIED., .F., .F. ) 
 B_SPLINE_CURVE_WITH_KNOTS ( ( 4, 4 ),
 ( 4.712388980384689674, 6.105785702739209064 ),
 .UNSPECIFIED. ) 
 CURVE ( )  GEOMETRIC_REPRESENTATION_ITEM ( )  RATIONAL_B_SPLINE_CURVE ( ( 1.000000000000000000, 0.8446433258982484205, 0.8446433258982484205, 1.000000000000000000 ) ) 
 REPRESENTATION_ITEM ( '' )  );
#77977=( BOUNDED_CURVE ( )  B_SPLINE_CURVE ( 2, ( #64791, #58052, #53175, #2158, #98819, #87959, #77120, #9666, #20534, #8906, #130045, #10379, #30747 ),
 .UNSPECIFIED., .F., .T. ) 
 B_SPLINE_CURVE_WITH_KNOTS ( ( 3, 2, 2, 2, 2, 2, 3 ),
 ( 0.3000000000000000444, 0.3083333333333334036, 0.3166666666666667074, 0.3250000000000000666, 0.3333333333333333703, 0.3416666666666667296, 0.3500000000000000333 ),
 .UNSPECIFIED. ) 
 CURVE ( )  GEOMETRIC_REPRESENTATION_ITEM ( )  RATIONAL_B_SPLINE_CURVE ( ( 0.9999999999999997780, 0.9659258262890685343, 1.000000000000000000, 0.9659258262890683122, 1.000000000000000000, 0.9659258262890683122, 1.000000000000000000, 0.9659258262890683122, 1.000000000000000000, 0.9659258262890683122, 1.000000000000000000, 0.9659258262890680902, 1.000000000000000222 ) ) 
 REPRESENTATION_ITEM ( '' )  );
#78051=ORIENTED_EDGE ( 'NONE', *, *, #120168, .T. ) ;
#78084=CARTESIAN_POINT ( 'NONE',  ( 12.37456980810188512, 6.871911579029510442, -3.967499999999998916 ) ) ;
#78095=UNCERTAINTY_MEASURE_WITH_UNIT (LENGTH_MEASURE( 1.000000000000000082E-05 ), #105656, 'distance_accuracy_value', 'NONE');
#78101=CARTESIAN_POINT ( 'NONE',  ( 27.99999999999999645, -49.14999999999999147, -49.92499999999968452 ) ) ;
#78116=LINE ( 'NONE', #22967, #2106 ) ;
#78119=UNCERTAINTY_MEASURE_WITH_UNIT (LENGTH_MEASURE( 1.000000000000000082E-05 ), #138510, 'distance_accuracy_value', 'NONE');
#78128=DIRECTION ( 'NONE',  ( 0.000000000000000000, 0.000000000000000000, -1.000000000000000000 ) ) ;
#78129=( LENGTH_UNIT ( ) NAMED_UNIT ( * ) SI_UNIT ( .MILLI., .METRE. ) );
#78132=CARTESIAN_POINT ( 'NONE',  ( 18.66666666666666785, -5.278424836066145431, -3.047499999999993658 ) ) ;
#78145=CARTESIAN_POINT ( 'NONE',  ( 126.7224180521723298, -45.84254607569018702, -35.55177538329009224 ) ) ;
#78154=DIRECTION ( 'NONE',  ( 0.000000000000000000, 0.000000000000000000, -1.000000000000000000 ) ) ;
#78188=CARTESIAN_POINT ( 'NONE',  ( 163.1915705344537741, 26.96999999999992781, 34.63378833274251889 ) ) ;
#78259=CARTESIAN_POINT ( 'NONE',  ( 15.67123647476855552, 0.000000000000000000, 7.934999999999990727 ) ) ;
#78263=EDGE_CURVE ( 'NONE', #68280, #84791, #37602, .T. ) ;
#78298=CARTESIAN_POINT ( 'NONE',  ( 19.08290314143522437, 3.967499999999992699, -6.871911579029513994 ) ) ;
#78299=CARTESIAN_POINT ( 'NONE',  ( 2.166236474768552966, 7.934999999999990727, -1.457635852685135314E-15 ) ) ;
#78312=ORIENTED_EDGE ( 'NONE', *, *, #45745, .F. ) ;
#78321=CARTESIAN_POINT ( 'NONE',  ( 17.50000000000000000, 0.000000000000000000, 6.094999999999989981 ) ) ;
#78340=B_SPLINE_CURVE_WITH_KNOTS ( 'NONE', 3,
 ( #65165, #53556, #99907, #12174, #142702, #109354, #42700, #119487, #31801, #64420, #88336, #131832 ),
 .UNSPECIFIED., .F., .F.,
 ( 4, 2, 2, 2, 2, 4 ),
 ( 0.000000000000000000, 0.001837441947543509788, 0.003674883895087019577, 0.004593604868858774254, 0.005512325842630529799, 0.007349767790174039153 ),
 .UNSPECIFIED. ) ;
#78350=VERTEX_POINT ( 'NONE', #88497 ) ;
#78375=EDGE_CURVE ( 'NONE', #140587, #17685, #116504, .T. ) ;
#78392=CARTESIAN_POINT ( 'NONE',  ( 28.00000000000002487, -52.14999999999999147, 34.92500000000003268 ) ) ;
#78406=DIRECTION ( 'NONE',  ( 0.2399999999999954947, -0.000000000000000000, 0.9707728879609288652 ) ) ;
#78412=CARTESIAN_POINT ( 'NONE',  ( 166.0610720213131799, 26.96999999999993847, -33.43488148127461557 ) ) ;
#78420=CARTESIAN_POINT ( 'NONE',  ( 32.15040314143522693, 7.934999999999989839, -2.126176841940961904 ) ) ;
#78433=MECHANICAL_DESIGN_GEOMETRIC_PRESENTATION_REPRESENTATION('',(#59916),#117811);
#78449=ORIENTED_EDGE ( 'NONE', *, *, #102081, .T. ) ;
#78476=ORIENTED_EDGE ( 'NONE', *, *, #1687, .F. ) ;
#78513=( GEOMETRIC_REPRESENTATION_CONTEXT ( 3 ) GLOBAL_UNCERTAINTY_ASSIGNED_CONTEXT ( ( #76709 ) ) GLOBAL_UNIT_ASSIGNED_CONTEXT ( ( #90263, #92392, #79455 ) ) REPRESENTATION_CONTEXT ( 'NONE', 'WORKASPACE' ) );
#78515=LINE ( 'NONE', #121987, #102228 ) ;
#78517=DIRECTION ( 'NONE',  ( -1.000000000000000000, -0.000000000000000000, -0.000000000000000000 ) ) ;
#78522=CARTESIAN_POINT ( 'NONE',  ( 152.4000000000000057, 7.919999999999947526, -16.42230000000002832 ) ) ;
#78538=AXIS2_PLACEMENT_3D ( 'NONE', #124803, #25469, #42102 ) ;
#78548=( GEOMETRIC_REPRESENTATION_CONTEXT ( 3 ) GLOBAL_UNCERTAINTY_ASSIGNED_CONTEXT ( ( #65113 ) ) GLOBAL_UNIT_ASSIGNED_CONTEXT ( ( #87432, #99711, #30173 ) ) REPRESENTATION_CONTEXT ( 'NONE', 'WORKASPACE' ) );
#78581=SURFACE_STYLE_FILL_AREA ( #65601 ) ;
#78590=FACE_OUTER_BOUND ( 'NONE', #49053, .T. ) ;
#78591=CARTESIAN_POINT ( 'NONE',  ( 0.9420698081018860082, 7.934999999999993392, 2.126176841940951689 ) ) ;
#78600=( NAMED_UNIT ( * ) PLANE_ANGLE_UNIT ( ) SI_UNIT ( $, .RADIAN. ) );
#78612=VECTOR ( 'NONE', #53080, 1000.000000000000000 ) ;
#78672=AXIS2_PLACEMENT_3D ( 'NONE', #67066, #111249, #11943 ) ;
#78762=EDGE_CURVE ( 'NONE', #81376, #69422, #53969, .T. ) ;
#78767=CARTESIAN_POINT ( 'NONE',  ( 5.295806282870439752, -5.278424836066144543, 3.047499999999995879 ) ) ;
#78778=FILL_AREA_STYLE ('',( #25074 ) ) ;
#78784=ORIENTED_EDGE ( 'NONE', *, *, #38611, .T. ) ;
#78791=CARTESIAN_POINT ( 'NONE',  ( 52.39921342269828841, -49.14999999999999147, 40.57473644908944976 ) ) ;
#78792=EDGE_LOOP ( 'NONE', ( #6560, #130143, #52800, #116439 ) ) ;
#78796=CARTESIAN_POINT ( 'NONE',  ( 16.31206980810189222, 7.934999999999993392, 2.126176841940951689 ) ) ;
#78810=AXIS2_PLACEMENT_3D ( 'NONE', #102335, #112477, #13842 ) ;
#78822=AXIS2_PLACEMENT_3D ( 'NONE', #120855, #67207, #87531 ) ;
#78827=CIRCLE ( 'NONE', #27895, 6.094999999999989093 ) ;
#78828=CARTESIAN_POINT ( 'NONE',  ( 17.69163961620376568, 6.094999999999988205, -1.633150327867694651 ) ) ;
#78832=SURFACE_SIDE_STYLE ('',( #123042 ) ) ;
#78836=( NAMED_UNIT ( * ) SI_UNIT ( $, .STERADIAN. ) SOLID_ANGLE_UNIT ( ) );
#78844=PLANE ( 'NONE',  #20852 ) ;
#78848=DIRECTION ( 'NONE',  ( 0.000000000000000000, -1.000000000000000000, 0.000000000000000000 ) ) ;
#78851=CARTESIAN_POINT ( 'NONE',  ( 11.66666666666666785, -5.278424836066145431, -3.047499999999993658 ) ) ;
#78852=CARTESIAN_POINT ( 'NONE',  ( 22.43706980810188867, 2.126176841940952134, -7.934999999999992504 ) ) ;
#78872=CARTESIAN_POINT ( 'NONE',  ( 28.00000000000002487, -49.14999999999999147, 34.92500000000003268 ) ) ;
#78873=SURFACE_STYLE_FILL_AREA ( #12151 ) ;
#78876=AXIS2_PLACEMENT_3D ( 'NONE', #91123, #124433, #25104 ) ;
#78898=ORIENTED_EDGE ( 'NONE', *, *, #108905, .T. ) ;
#78914=CARTESIAN_POINT ( 'NONE',  ( 22.81706980810188767, -2.126176841940956130, 7.934999999999990727 ) ) ;
#78917=CARTESIAN_POINT ( 'NONE',  ( 3.102554694470408325, -48.63825160239813528, -38.47250499286691650 ) ) ;
#78918=CARTESIAN_POINT ( 'NONE',  ( 15.21247294953710671, 0.000000000000000000, 6.094999999999989981 ) ) ;
#78925=EDGE_LOOP ( 'NONE', ( #135811, #124049, #138736, #19368 ) ) ;
#78936=AXIS2_PLACEMENT_3D ( 'NONE', #132521, #44809, #142643 ) ;
#78988=CARTESIAN_POINT ( 'NONE',  ( 19.46290314143521982, -3.967499999999994476, 6.871911579029513106 ) ) ;
#79025=FILL_AREA_STYLE_COLOUR ( '', #53566 ) ;
#79028=EDGE_CURVE ( 'NONE', #28418, #15743, #107632, .T. ) ;
#79033=LINE ( 'NONE', #57275, #34566 ) ;
#79039=CARTESIAN_POINT ( 'NONE',  ( 19.37456980810188867, 6.871911579029510442, -3.967499999999998916 ) ) ;
#79040=CARTESIAN_POINT ( 'NONE',  ( 3.041236474768552966, 0.000000000000000000, 7.934999999999990727 ) ) ;
#79053=VERTEX_POINT ( 'NONE', #137532 ) ;
#79080=ADVANCED_FACE ( 'NONE', ( #82434 ), #83889, .F. ) ;
#79101=PRESENTATION_STYLE_ASSIGNMENT (( #14511 ) ) ;
#79139=DIRECTION ( 'NONE',  ( -1.000000000000000000, 0.000000000000000000, 0.000000000000000000 ) ) ;
#79148=CARTESIAN_POINT ( 'NONE',  ( 184.1500000000000057, -3.180000000000061444, -31.92499999999998295 ) ) ;
#79161=CARTESIAN_POINT ( 'NONE',  ( 165.1757173328947772, 26.96999999999993847, -33.99520319345304387 ) ) ;
#79168=CARTESIAN_POINT ( 'NONE',  ( 25.73373647476855552, 5.808823158059036373, 5.808823158059032821 ) ) ;
#79184=ORIENTED_EDGE ( 'NONE', *, *, #28784, .T. ) ;
#79207=EDGE_CURVE ( 'NONE', #63837, #29858, #63396, .T. ) ;
#79225=( LENGTH_UNIT ( ) NAMED_UNIT ( * ) SI_UNIT ( .MILLI., .METRE. ) );
#79231=CARTESIAN_POINT ( 'NONE',  ( 1.325532373446378864, -3.000483569180001808, -6.075707327269213032 ) ) ;
#79235=CARTESIAN_POINT ( 'NONE',  ( 25.40000000000000213, 6.316876854325914614, 3.503673674027464546 ) ) ;
#79242=DIRECTION ( 'NONE',  ( 0.000000000000000000, 0.000000000000000000, 1.000000000000000000 ) ) ;
#79245=CARTESIAN_POINT ( 'NONE',  ( 1.219720151767342609, 2.263774094906783052, 6.495225715523759824 ) ) ;
#79246=PRESENTATION_STYLE_ASSIGNMENT (( #70516 ) ) ;
#79265=CIRCLE ( 'NONE', #69947, 2.000000000000001776 ) ;
#79349=CARTESIAN_POINT ( 'NONE',  ( 0.6504031414352192675, 7.934999999999989839, -2.126176841940961904 ) ) ;
#79369=CYLINDRICAL_SURFACE ( 'NONE', #18544, 6.094999999999989093 ) ;
#79382=( NAMED_UNIT ( * ) PLANE_ANGLE_UNIT ( ) SI_UNIT ( $, .RADIAN. ) );
#79386=CIRCLE ( 'NONE', #42314, 1.000000000000000888 ) ;
#79395=DIRECTION ( 'NONE',  ( 0.000000000000000000, -1.000000000000000000, 0.000000000000000000 ) ) ;
#79404=ORIENTED_EDGE ( 'NONE', *, *, #110303, .T. ) ;
#79408=MECHANICAL_DESIGN_GEOMETRIC_PRESENTATION_REPRESENTATION('',(#19123),#26070);
#79410=MECHANICAL_DESIGN_GEOMETRIC_PRESENTATION_REPRESENTATION('',(#93215),#111749);
#79421=UNCERTAINTY_MEASURE_WITH_UNIT (LENGTH_MEASURE( 1.000000000000000082E-05 ), #126590, 'distance_accuracy_value', 'NONE');
#79423=EDGE_CURVE ( 'NONE', #46517, #75731, #128153, .T. ) ;
#79437=ORIENTED_EDGE ( 'NONE', *, *, #1687, .T. ) ;
#79443=ORIENTED_EDGE ( 'NONE', *, *, #100384, .T. ) ;
#79446=SURFACE_STYLE_FILL_AREA ( #135230 ) ;
#79453=AXIS2_PLACEMENT_3D ( 'NONE', #76002, #141242, #120175 ) ;
#79455=( NAMED_UNIT ( * ) SI_UNIT ( $, .STERADIAN. ) SOLID_ANGLE_UNIT ( ) );
#79507=CARTESIAN_POINT ( 'NONE',  ( 25.39999999999999503, 7.925800835032758229, -0.5567874546942058744 ) ) ;
#79516=ADVANCED_FACE ( 'NONE', ( #87255 ), #67734, .T. ) ;
#79525=CARTESIAN_POINT ( 'NONE',  ( 7.629139616203772789, 5.278424836066147208, 3.047499999999990550 ) ) ;
#79534=ORIENTED_EDGE ( 'NONE', *, *, #35081, .T. ) ;
#79546=DIRECTION ( 'NONE',  ( 0.000000000000000000, 2.556434596176436916E-15, 1.000000000000000000 ) ) ;
#79553=CARTESIAN_POINT ( 'NONE',  ( 25.64540314143522082, -2.126176841940958351, -7.934999999999989839 ) ) ;
#79582=ORIENTED_EDGE ( 'NONE', *, *, #112952, .T. ) ;
#79588=DIRECTION ( 'NONE',  ( 0.000000000000000000, -0.000000000000000000, -1.000000000000000000 ) ) ;
#79599=ORIENTED_EDGE ( 'NONE', *, *, #110687, .T. ) ;
#79600=FILL_AREA_STYLE_COLOUR ( '', #93146 ) ;
#79603=CARTESIAN_POINT ( 'NONE',  ( 13.85416666666666430, 1.633150327867695095, 6.094999999999988205 ) ) ;
#79620=PRESENTATION_STYLE_ASSIGNMENT (( #123080 ) ) ;
#79637=ADVANCED_FACE ( 'NONE', ( #4267 ), #121997, .F. ) ;
#79663=CARTESIAN_POINT ( 'NONE',  ( 3.010806948443980779, -48.09618305010688744, -37.50858089739958956 ) ) ;
#79667=ORIENTED_EDGE ( 'NONE', *, *, #22688, .F. ) ;
#79715=ORIENTED_EDGE ( 'NONE', *, *, #14329, .T. ) ;
#79722=ORIENTED_EDGE ( 'NONE', *, *, #140761, .F. ) ;
#79727=CARTESIAN_POINT ( 'NONE',  ( 26.60873647476855552, -5.808823158059033709, 5.808823158059035485 ) ) ;
#79751=CARTESIAN_POINT ( 'NONE',  ( 57.42758194782751247, -45.84254607569121021, -35.55177538329067488 ) ) ;
#79769=CARTESIAN_POINT ( 'NONE',  ( 16.45790314143522082, 6.871911579029515771, 3.967499999999989146 ) ) ;
#79775=VERTEX_POINT ( 'NONE', #5738 ) ;
#79800=( NAMED_UNIT ( * ) PLANE_ANGLE_UNIT ( ) SI_UNIT ( $, .RADIAN. ) );
#79823=CARTESIAN_POINT ( 'NONE',  ( 2.400403141435219379, -7.934999999999988951, 2.126176841940957907 ) ) ;
#79830=EDGE_LOOP ( 'NONE', ( #14882, #46334, #13148, #92623 ) ) ;
#79879=CARTESIAN_POINT ( 'NONE',  ( 164.5340954016161561, 26.96999999999993847, -34.26735321372807164 ) ) ;
#79889=CARTESIAN_POINT ( 'NONE',  ( 27.92123647476855197, -9.717572351234235426E-16, -7.934999999999990727 ) ) ;
#79930=( NAMED_UNIT ( * ) PLANE_ANGLE_UNIT ( ) SI_UNIT ( $, .RADIAN. ) );
#79934=CARTESIAN_POINT ( 'NONE',  ( 0.000000000000000000, -57.15000000000003411, -15.92500000000064730 ) ) ;
#79939=ORIENTED_EDGE ( 'NONE', *, *, #117555, .T. ) ;
#79942=CARTESIAN_POINT ( 'NONE',  ( 0.6293903851252851123, -7.359378872481451950, -1.291302361894904660 ) ) ;
#79946=CARTESIAN_POINT ( 'NONE',  ( 25.40000000000000568, 5.131534016557159461, 4.434051995216958808 ) ) ;
#80040=EDGE_LOOP ( 'NONE', ( #133338, #61670, #62997, #79939, #134854, #104909, #83803, #98707, #57333, #18810, #65733, #79582, #11893, #6085, #142726 ) ) ;
#80054=CARTESIAN_POINT ( 'NONE',  ( 32.12913961620377989, 5.278424836066147208, 3.047499999999990550 ) ) ;
#80074=CARTESIAN_POINT ( 'NONE',  ( 25.39999999999999858, -57.15000000000003411, 15.92499999999935589 ) ) ;
#80077=CARTESIAN_POINT ( 'NONE',  ( 21.33747294953710849, 6.094999999999989981, -1.119633336120465690E-15 ) ) ;
#80122=AXIS2_PLACEMENT_3D ( 'NONE', #103036, #88610, #22576 ) ;
#80196=SURFACE_STYLE_FILL_AREA ( #59167 ) ;
#80214=CARTESIAN_POINT ( 'NONE',  ( 9.379139616203772789, -5.278424836066145431, -3.047499999999993658 ) ) ;
#80220=FILL_AREA_STYLE ('',( #59189 ) ) ;
#80239=CARTESIAN_POINT ( 'NONE',  ( 23.45790314143522437, 6.871911579029515771, 3.967499999999989146 ) ) ;
#80242=CARTESIAN_POINT ( 'NONE',  ( 0.000000000000000000, -57.14999999999999147, -34.92499999999972715 ) ) ;
#80282=VECTOR ( 'NONE', #89580, 1000.000000000000000 ) ;
#80286=CARTESIAN_POINT ( 'NONE',  ( 13.56250000000000000, 4.461849672132300881, 4.461849672132299105 ) ) ;
#80287=CARTESIAN_POINT ( 'NONE',  ( 21.99956980810188867, -3.967499999999998028, -6.871911579029511330 ) ) ;
#80410=CARTESIAN_POINT ( 'NONE',  ( 31.56706980810188767, 2.126176841940952134, -7.934999999999993392 ) ) ;
#80431=CARTESIAN_POINT ( 'NONE',  ( 56.52198303709688787, -46.44627868284322858, -35.89947574910193850 ) ) ;
#80451=CARTESIAN_POINT ( 'NONE',  ( 25.35373647476855297, -5.808823158059035485, -5.808823158059033709 ) ) ;
#80472=LINE ( 'NONE', #59445, #104425 ) ;
#80482=FILL_AREA_STYLE_COLOUR ( '', #137105 ) ;
#80493=CARTESIAN_POINT ( 'NONE',  ( 0.1600000000000026401, -9.717572351234235426E-16, -7.934999999999990727 ) ) ;
#80508=EDGE_CURVE ( 'NONE', #9588, #91284, #47166, .T. ) ;
#80542=( GEOMETRIC_REPRESENTATION_CONTEXT ( 3 ) GLOBAL_UNCERTAINTY_ASSIGNED_CONTEXT ( ( #111624 ) ) GLOBAL_UNIT_ASSIGNED_CONTEXT ( ( #118874, #63109, #97847 ) ) REPRESENTATION_CONTEXT ( 'NONE', 'WORKASPACE' ) );
#80550=FILL_AREA_STYLE_COLOUR ( '', #112993 ) ;
#80551=EDGE_CURVE ( 'NONE', #98765, #115565, #2278, .T. ) ;
#80562=DIRECTION ( 'NONE',  ( -0.000000000000000000, -0.000000000000000000, 1.000000000000000000 ) ) ;
#80568=EDGE_CURVE ( 'NONE', #2777, #79775, #135012, .T. ) ;
#80573=CARTESIAN_POINT ( 'NONE',  ( 31.27540314143522693, -2.126176841940958351, -7.934999999999989839 ) ) ;
#80574=CARTESIAN_POINT ( 'NONE',  ( 2.692069808101885897, -7.934999999999991616, -2.126176841940955242 ) ) ;
#80586=SURFACE_SIDE_STYLE ('',( #137091 ) ) ;
#80625=ORIENTED_EDGE ( 'NONE', *, *, #71815, .T. ) ;
#80652=VERTEX_POINT ( 'NONE', #3702 ) ;
#80668=EDGE_CURVE ( 'NONE', #47857, #672, #14606, .T. ) ;
#80703=ADVANCED_FACE ( 'NONE', ( #12073 ), #100537, .F. ) ;
#80715=ORIENTED_EDGE ( 'NONE', *, *, #107178, .T. ) ;
#80748=CARTESIAN_POINT ( 'NONE',  ( 2.692069808101885897, -7.934999999999991616, -2.126176841940955242 ) ) ;
#80770=CARTESIAN_POINT ( 'NONE',  ( 27.99999999999999645, -57.14999999999999147, -45.92499999999969873 ) ) ;
#80776=CARTESIAN_POINT ( 'NONE',  ( 4.791236474768552966, -9.717572351234235426E-16, -7.934999999999990727 ) ) ;
#80782=FACE_OUTER_BOUND ( 'NONE', #73404, .T. ) ;
#80784=FILL_AREA_STYLE_COLOUR ( '', #96842 ) ;
#80805=CARTESIAN_POINT ( 'NONE',  ( 128.7663314791381026, -49.19090614206155010, 40.79110616922538668 ) ) ;
#80810=DIRECTION ( 'NONE',  ( 0.000000000000000000, 0.000000000000000000, 1.000000000000000000 ) ) ;
#80812=UNCERTAINTY_MEASURE_WITH_UNIT (LENGTH_MEASURE( 1.000000000000000082E-05 ), #12780, 'distance_accuracy_value', 'NONE');
#80816=EDGE_CURVE ( 'NONE', #63172, #132990, #104933, .T. ) ;
#80826=VECTOR ( 'NONE', #33385, 1000.000000000000000 ) ;
#80836=STYLED_ITEM ( 'NONE', ( #44676 ), #51969 ) ;
#80853=SURFACE_STYLE_USAGE ( .BOTH. , #136626 ) ;
#80859=ORIENTED_EDGE ( 'NONE', *, *, #77719, .T. ) ;
#80864=VERTEX_POINT ( 'NONE', #137449 ) ;
#80886=CARTESIAN_POINT ( 'NONE',  ( 2.962472949537105826, -7.464222240803106570E-16, -6.094999999999989981 ) ) ;
#80904=ORIENTED_EDGE ( 'NONE', *, *, #8812, .T. ) ;
#80906=CARTESIAN_POINT ( 'NONE',  ( 9.087472949537108491, -6.094999999999989981, 3.732111120401553285E-16 ) ) ;
#80911=PRESENTATION_STYLE_ASSIGNMENT (( #71459 ) ) ;
#80941=CARTESIAN_POINT ( 'NONE',  ( 27.24956980810188867, 3.967499999999998916, 6.871911579029510442 ) ) ;
#80967=DIRECTION ( 'NONE',  ( 0.000000000000000000, 0.000000000000000000, 1.000000000000000000 ) ) ;
#80985=CARTESIAN_POINT ( 'NONE',  ( 25.81250000000000000, -4.461849672132299993, -4.461849672132299105 ) ) ;
#81023=CIRCLE ( 'NONE', #90202, 1.000000000000000888 ) ;
#81047=CARTESIAN_POINT ( 'NONE',  ( 23.54623647476855552, -7.934999999999990727, 4.858786175617117713E-16 ) ) ;
#81050=DIRECTION ( 'NONE',  ( 0.000000000000000000, 0.000000000000000000, -1.000000000000000000 ) ) ;
#81055=ORIENTED_EDGE ( 'NONE', *, *, #36533, .T. ) ;
#81082=AXIS2_PLACEMENT_3D ( 'NONE', #25126, #125174, #80967 ) ;
#81114=FACE_OUTER_BOUND ( 'NONE', #107505, .T. ) ;
#81118=CARTESIAN_POINT ( 'NONE',  ( 26.31706980810189123, -2.126176841940956130, 7.934999999999991616 ) ) ;
#81131=CARTESIAN_POINT ( 'NONE',  ( 0.000000000000000000, -14.29000000000013593, 12.69999999999954632 ) ) ;
#81132=VECTOR ( 'NONE', #103967, 1000.000000000000000 ) ;
#81160=CARTESIAN_POINT ( 'NONE',  ( 31.62456980810188867, -6.871911579029512218, 3.967499999999996252 ) ) ;
#81162=CARTESIAN_POINT ( 'NONE',  ( 1.291236474768552966, -9.717572351234235426E-16, -7.934999999999990727 ) ) ;
#81185=CARTESIAN_POINT ( 'NONE',  ( 25.39999999999999858, -14.29000000000013593, -12.70000000000045404 ) ) ;
#81190=CIRCLE ( 'NONE', #62658, 28.00000000000002487 ) ;
#81205=STYLED_ITEM ( 'NONE', ( #12210 ), #116870 ) ;
#81219=ORIENTED_EDGE ( 'NONE', *, *, #33671, .T. ) ;
#81244=DIRECTION ( 'NONE',  ( -1.000000000000000000, -0.000000000000000000, 0.000000000000000000 ) ) ;
#81247=ORIENTED_EDGE ( 'NONE', *, *, #83419, .F. ) ;
#81251=AXIS2_PLACEMENT_3D ( 'NONE', #90207, #46770, #81512 ) ;
#81260=B_SPLINE_CURVE_WITH_KNOTS ( 'NONE', 3,
 ( #73275, #8658, #117442, #29726 ),
 .UNSPECIFIED., .F., .F.,
 ( 4, 4 ),
 ( 0.000000000000000000, 0.001115544020566869386 ),
 .UNSPECIFIED. ) ;
#81262=SURFACE_SIDE_STYLE ('',( #37011 ) ) ;
#81267=CARTESIAN_POINT ( 'NONE',  ( 25.39999999999999858, -30.18000000000009564, 15.92499999999935945 ) ) ;
#81289=ORIENTED_EDGE ( 'NONE', *, *, #50610, .T. ) ;
#81292=CARTESIAN_POINT ( 'NONE',  ( 3.567069808101885897, 2.126176841940952134, -7.934999999999993392 ) ) ;
#81374=( NAMED_UNIT ( * ) SI_UNIT ( $, .STERADIAN. ) SOLID_ANGLE_UNIT ( ) );
#81376=VERTEX_POINT ( 'NONE', #44965 ) ;
#81383=AXIS2_PLACEMENT_3D ( 'NONE', #30557, #140717, #140040 ) ;
#81407=CARTESIAN_POINT ( 'NONE',  ( 25.39999999999999858, 7.464222240803104598E-16, -6.094999999999989093 ) ) ;
#81409=CARTESIAN_POINT ( 'NONE',  ( 183.3316408629058287, -52.14999999999999147, 41.64499999999997470 ) ) ;
#81424=SURFACE_STYLE_FILL_AREA ( #3105 ) ;
#81430=( GEOMETRIC_REPRESENTATION_CONTEXT ( 3 ) GLOBAL_UNCERTAINTY_ASSIGNED_CONTEXT ( ( #131758 ) ) GLOBAL_UNIT_ASSIGNED_CONTEXT ( ( #50087, #126208, #5095 ) ) REPRESENTATION_CONTEXT ( 'NONE', 'WORKASPACE' ) );
#81471=CARTESIAN_POINT ( 'NONE',  ( 5.317069808101885897, -2.126176841940956130, 7.934999999999991616 ) ) ;
#81499=( LENGTH_UNIT ( ) NAMED_UNIT ( * ) SI_UNIT ( .MILLI., .METRE. ) );
#81505=CARTESIAN_POINT ( 'NONE',  ( 1.728736474768552522, 5.808823158059031044, -5.808823158059038150 ) ) ;
#81512=DIRECTION ( 'NONE',  ( 0.000000000000000000, 0.000000000000000000, 1.000000000000000000 ) ) ;
#81517=CARTESIAN_POINT ( 'NONE',  ( 184.0335292699550678, -51.38852430739337507, -37.54101415799217278 ) ) ;
#81536=CARTESIAN_POINT ( 'NONE',  ( 128.8216926156734132, -52.14999999996970814, 41.05175048930652082 ) ) ;
#81595=FACE_OUTER_BOUND ( 'NONE', #46681, .T. ) ;
#81610=CIRCLE ( 'NONE', #56173, 3.999999999999996447 ) ;
#81613=MECHANICAL_DESIGN_GEOMETRIC_PRESENTATION_REPRESENTATION('',(#137180),#12138);
#81639=CARTESIAN_POINT ( 'NONE',  ( 11.56663961620376924, 1.633150327867695095, 6.094999999999988205 ) ) ;
#81672=CARTESIAN_POINT ( 'NONE',  ( 24.04123647476855652, 0.000000000000000000, 7.934999999999990727 ) ) ;
#81686=FACE_OUTER_BOUND ( 'NONE', #112442, .T. ) ;
#81702=VERTEX_POINT ( 'NONE', #40479 ) ;
#81720=CARTESIAN_POINT ( 'NONE',  ( 23.91666666666666785, 5.278424836066147208, 3.047499999999990550 ) ) ;
#81721=PRESENTATION_STYLE_ASSIGNMENT (( #74943 ) ) ;
#81748=CARTESIAN_POINT ( 'NONE',  ( 1.889689338576429289, -5.719221863398560757, 2.436636208257458858 ) ) ;
#81751=EDGE_CURVE ( 'NONE', #125982, #33206, #28156, .T. ) ;
#81780=CARTESIAN_POINT ( 'NONE',  ( 28.00000000000002487, -52.14999999999999147, -62.92499999999978400 ) ) ;
#81790=( BOUNDED_CURVE ( )  B_SPLINE_CURVE ( 2, ( #47462, #3172, #27072, #82213, #90938, #2444, #80077, #91627, #46755, #135165, #104636, #5303, #124252 ),
 .UNSPECIFIED., .F., .F. ) 
 B_SPLINE_CURVE_WITH_KNOTS ( ( 3, 2, 2, 2, 2, 2, 3 ),
 ( 0.6500000000000001332, 0.6583333333333334370, 0.6666666666666667407, 0.6750000000000001554, 0.6833333333333334592, 0.6916666666666667629, 0.7000000000000000666 ),
 .UNSPECIFIED. ) 
 CURVE ( )  GEOMETRIC_REPRESENTATION_ITEM ( )  RATIONAL_B_SPLINE_CURVE ( ( 0.9999999999999995559, 0.9659258262890687563, 1.000000000000000000, 0.9659258262890683122, 1.000000000000000000, 0.9659258262890683122, 1.000000000000000000, 0.9659258262890683122, 1.000000000000000000, 0.9659258262890683122, 1.000000000000000000, 0.9659258262890678681, 1.000000000000000444 ) ) 
 REPRESENTATION_ITEM ( '' )  );
#81793=FACE_OUTER_BOUND ( 'NONE', #76160, .T. ) ;
#81801=DIRECTION ( 'NONE',  ( 0.000000000000000000, 0.000000000000000000, 1.000000000000000000 ) ) ;
#81815=EDGE_CURVE ( 'NONE', #49412, #34663, #11030, .T. ) ;
#81831=ADVANCED_FACE ( 'NONE', ( #12091 ), #110669, .F. ) ;
#81839=CARTESIAN_POINT ( 'NONE',  ( 25.39999999999999858, -2.599999999999900169, -1.445354724476153568E-14 ) ) ;
#81852=CARTESIAN_POINT ( 'NONE',  ( 29.81706980810189478, -2.126176841940956130, 7.934999999999991616 ) ) ;
#81861=PRESENTATION_STYLE_ASSIGNMENT (( #103546 ) ) ;
#81862=ORIENTED_EDGE ( 'NONE', *, *, #142868, .T. ) ;
#81884=LINE ( 'NONE', #36898, #49021 ) ;
#81898=CARTESIAN_POINT ( 'NONE',  ( 26.08290314143522082, 3.967499999999992699, -6.871911579029513994 ) ) ;
#81899=CARTESIAN_POINT ( 'NONE',  ( 7.707903141435219929, -6.871911579029513106, -3.967499999999993587 ) ) ;
#81911=CARTESIAN_POINT ( 'NONE',  ( 22.21247294953710494, 0.000000000000000000, 6.094999999999989981 ) ) ;
#81917=CARTESIAN_POINT ( 'NONE',  ( 131.8806778009766276, -52.14999999999999147, -40.92499999999998295 ) ) ;
#81930=ADVANCED_FACE ( 'NONE', ( #70798 ), #115855, .T. ) ;
#81957=( NAMED_UNIT ( * ) SI_UNIT ( $, .STERADIAN. ) SOLID_ANGLE_UNIT ( ) );
#81966=VERTEX_POINT ( 'NONE', #127282 ) ;
#81974=VECTOR ( 'NONE', #18114, 1000.000000000000000 ) ;
#81978=DIRECTION ( 'NONE',  ( 0.000000000000000000, -1.000000000000000000, 0.000000000000000000 ) ) ;
#82010=( LENGTH_UNIT ( ) NAMED_UNIT ( * ) SI_UNIT ( .MILLI., .METRE. ) );
#82024=( NAMED_UNIT ( * ) SI_UNIT ( $, .STERADIAN. ) SOLID_ANGLE_UNIT ( ) );
#82031=ORIENTED_EDGE ( 'NONE', *, *, #52372, .T. ) ;
#82033=( LENGTH_UNIT ( ) NAMED_UNIT ( * ) SI_UNIT ( .MILLI., .METRE. ) );
#82036=CARTESIAN_POINT ( 'NONE',  ( 180.9625229943972329, -48.82538788374324668, -38.96958855984423309 ) ) ;
#82098=FACE_OUTER_BOUND ( 'NONE', #47340, .T. ) ;
#82109=CYLINDRICAL_SURFACE ( 'NONE', #97838, 3.999999999999996447 ) ;
#82161=AXIS2_PLACEMENT_3D ( 'NONE', #101831, #2484, #35896 ) ;
#82181=ADVANCED_FACE ( 'NONE', ( #11179 ), #124116, .T. ) ;
#82189=CARTESIAN_POINT ( 'NONE',  ( 10.56706980810188945, 2.126176841940952134, -7.934999999999993392 ) ) ;
#82213=CARTESIAN_POINT ( 'NONE',  ( 20.89997294953711204, 4.461849672132297329, -4.461849672132302658 ) ) ;
#82222=CARTESIAN_POINT ( 'NONE',  ( 6.832903141435220817, -3.967499999999994476, 6.871911579029513106 ) ) ;
#82230=( NAMED_UNIT ( * ) SI_UNIT ( $, .STERADIAN. ) SOLID_ANGLE_UNIT ( ) );
#82244=CARTESIAN_POINT ( 'NONE',  ( 1.774971111182638506, 0.9254518332604928510, -6.256315204308075195 ) ) ;
#82275=EDGE_CURVE ( 'NONE', #42602, #127303, #136557, .T. ) ;
#82288=FILL_AREA_STYLE_COLOUR ( '', #1482 ) ;
#82293=ADVANCED_FACE ( 'NONE', ( #80782 ), #134543, .T. ) ;
#82310=EDGE_LOOP ( 'NONE', ( #37002, #37601, #23825, #119823 ) ) ;
#82339=CARTESIAN_POINT ( 'NONE',  ( 15.94163961620377279, -6.094999999999989093, 1.633150327867691765 ) ) ;
#82371=CARTESIAN_POINT ( 'NONE',  ( 21.27040314143522437, -7.934999999999989839, 2.126176841940957907 ) ) ;
#82413=CARTESIAN_POINT ( 'NONE',  ( 18.95833333333333570, -3.047499999999997211, -5.278424836066143655 ) ) ;
#82414=CYLINDRICAL_SURFACE ( 'NONE', #116238, 1.000000000000000888 ) ;
#82432=CARTESIAN_POINT ( 'NONE',  ( 13.85416666666666963, 1.633150327867675555, 6.094999999999998863 ) ) ;
#82434=FACE_OUTER_BOUND ( 'NONE', #106485, .T. ) ;
#82437=ADVANCED_FACE ( 'NONE', ( #128557 ), #86490, .F. ) ;
#82439=AXIS2_PLACEMENT_3D ( 'NONE', #84758, #106466, #63038 ) ;
#82478=CARTESIAN_POINT ( 'NONE',  ( 151.4000000000000057, -16.48000000000005016, 33.92499999999998295 ) ) ;
#82481=( NAMED_UNIT ( * ) SI_UNIT ( $, .STERADIAN. ) SOLID_ANGLE_UNIT ( ) );
#82489=CARTESIAN_POINT ( 'NONE',  ( 25.39999999999999858, 0.000000000000000000, 0.000000000000000000 ) ) ;
#82529=CARTESIAN_POINT ( 'NONE',  ( 24.27540314143521982, -2.126176841940958351, -7.934999999999989839 ) ) ;
#82532=MECHANICAL_DESIGN_GEOMETRIC_PRESENTATION_REPRESENTATION('',(#33909),#6110);
#82552=CARTESIAN_POINT ( 'NONE',  ( 57.34909574878783189, -49.32595796886460704, -36.54674188582485783 ) ) ;
#82572=CARTESIAN_POINT ( 'NONE',  ( 33.52040314143522437, 7.934999999999989839, -2.126176841940961904 ) ) ;
#82573=CARTESIAN_POINT ( 'NONE',  ( 8.874569808101886892, 6.871911579029510442, -3.967499999999998916 ) ) ;
#82631=DIRECTION ( 'NONE',  ( -1.000000000000000000, -0.000000000000000000, -0.000000000000000000 ) ) ;
#82633=CARTESIAN_POINT ( 'NONE',  ( 7.504569808101886785, 6.871911579029510442, -3.967499999999998916 ) ) ;
#82651=CARTESIAN_POINT ( 'NONE',  ( 5.541666666666666963, 3.047499999999993214, -5.278424836066146320 ) ) ;
#82676=CARTESIAN_POINT ( 'NONE',  ( 151.4000000000000057, -17.48000000000005016, 33.92499999999998295 ) ) ;
#82690=EDGE_LOOP ( 'NONE', ( #78312, #117451, #119282, #24308 ) ) ;
#82692=( NAMED_UNIT ( * ) SI_UNIT ( $, .STERADIAN. ) SOLID_ANGLE_UNIT ( ) );
#82696=DIRECTION ( 'NONE',  ( 0.000000000000000000, -1.000000000000000000, 0.000000000000000000 ) ) ;
#82706=CARTESIAN_POINT ( 'NONE',  ( 3.129569808101886341, -3.967499999999998028, -6.871911579029511330 ) ) ;
#82710=CARTESIAN_POINT ( 'NONE',  ( 0.000000000000000000, -30.18000000000009564, 15.92499999999935945 ) ) ;
#82720=CARTESIAN_POINT ( 'NONE',  ( 181.0893910107582201, -48.47007572038016576, -38.12657027910816510 ) ) ;
#82737=CYLINDRICAL_SURFACE ( 'NONE', #78538, 28.00000000000002487 ) ;
#82743=( GEOMETRIC_REPRESENTATION_CONTEXT ( 3 ) GLOBAL_UNCERTAINTY_ASSIGNED_CONTEXT ( ( #124271 ) ) GLOBAL_UNIT_ASSIGNED_CONTEXT ( ( #105053, #50676, #6398 ) ) REPRESENTATION_CONTEXT ( 'NONE', 'WORKASPACE' ) );
#82749=SURFACE_STYLE_USAGE ( .BOTH. , #136394 ) ;
#82855=COLOUR_RGB ( '', 0.72549020, 0.75294118, 0.79215686) ;
#82856=CARTESIAN_POINT ( 'NONE',  ( 26.40000000000000568, -17.48000000000005016, -12.70000000000043272 ) ) ;
#82858=EDGE_CURVE ( 'NONE', #14349, #142647, #44166, .T. ) ;
#82866=CARTESIAN_POINT ( 'NONE',  ( 16.91666666666666785, 5.278424836066147208, 3.047499999999990550 ) ) ;
#82883=( GEOMETRIC_REPRESENTATION_CONTEXT ( 3 ) GLOBAL_UNCERTAINTY_ASSIGNED_CONTEXT ( ( #104081 ) ) GLOBAL_UNIT_ASSIGNED_CONTEXT ( ( #83564, #137934, #38615 ) ) REPRESENTATION_CONTEXT ( 'NONE', 'WORKASPACE' ) );
#82885=CARTESIAN_POINT ( 'NONE',  ( 11.15040314143521982, 7.934999999999989839, -2.126176841940961904 ) ) ;
#82893=CARTESIAN_POINT ( 'NONE',  ( 10.69163961620377279, 6.094999999999988205, -1.633150327867694651 ) ) ;
#82918=CARTESIAN_POINT ( 'NONE',  ( 3.770403141435219041, -7.934999999999989839, 2.126176841940957907 ) ) ;
#82920=DIRECTION ( 'NONE',  ( 0.000000000000000000, 0.000000000000000000, 1.000000000000000000 ) ) ;
#82929=DIRECTION ( 'NONE',  ( 0.000000000000000000, 0.000000000000000000, 1.000000000000000000 ) ) ;
#82939=CARTESIAN_POINT ( 'NONE',  ( 1.693225894565048240, 0.2328265696750401181, -6.401774105435452000 ) ) ;
#83009=SURFACE_SIDE_STYLE ('',( #69285 ) ) ;
#83040=CARTESIAN_POINT ( 'NONE',  ( 17.69163961620376924, 6.094999999999988205, -1.633150327867694651 ) ) ;
#83060=COLOUR_RGB ( '', 0.31764706, 0.68627451, 0.89019608) ;
#83071=ORIENTED_EDGE ( 'NONE', *, *, #93032, .T. ) ;
#83072=COLOUR_RGB ( '', 0.09019608, 0.27058824, 0.51372549) ;
#83075=CARTESIAN_POINT ( 'NONE',  ( 28.70790314143522437, -6.871911579029513106, -3.967499999999993587 ) ) ;
#83086=CARTESIAN_POINT ( 'NONE',  ( 3.340980275924462894, -49.02095135882305499, -39.67421197283063350 ) ) ;
#83106=ORIENTED_EDGE ( 'NONE', *, *, #119198, .F. ) ;
#83116=DIRECTION ( 'NONE',  ( 0.000000000000000000, 0.000000000000000000, -1.000000000000000000 ) ) ;
#83117=ORIENTED_EDGE ( 'NONE', *, *, #38407, .T. ) ;
#83119=EDGE_CURVE ( 'NONE', #71833, #80864, #117836, .T. ) ;
#83121=CARTESIAN_POINT ( 'NONE',  ( 22.16666666666666785, -5.278424836066145431, -3.047499999999993658 ) ) ;
#83137=ADVANCED_FACE ( 'NONE', ( #105545 ), #50483, .T. ) ;
#83174=CARTESIAN_POINT ( 'NONE',  ( 25.40000000000000213, -6.313548140616198623, -3.022842017553198257 ) ) ;
#83175=SURFACE_STYLE_USAGE ( .BOTH. , #62871 ) ;
#83204=CARTESIAN_POINT ( 'NONE',  ( 12.73330628287043886, -6.094999999999989981, -1.633150327867689322 ) ) ;
#83218=CARTESIAN_POINT ( 'NONE',  ( 25.39999999999999858, -7.600000000000061817, 34.92499999999998295 ) ) ;
#83225=FILL_AREA_STYLE ('',( #138318 ) ) ;
#83241=CARTESIAN_POINT ( 'NONE',  ( -0.1670968585647806814, -3.967499999999994476, 6.871911579029513106 ) ) ;
#83260=CARTESIAN_POINT ( 'NONE',  ( 181.1499999999998067, -49.85820393249939286, 34.92500000000001847 ) ) ;
#83268=CARTESIAN_POINT ( 'NONE',  ( 56.65265948608890767, -50.37061236291224020, -37.32649486623387247 ) ) ;
#83286=CARTESIAN_POINT ( 'NONE',  ( 32.64540314143522437, -2.126176841940958351, -7.934999999999989839 ) ) ;
#83287=CARTESIAN_POINT ( 'NONE',  ( 11.49956980810188689, -3.967499999999998028, -6.871911579029511330 ) ) ;
#83310=VECTOR ( 'NONE', #14276, 1000.000000000000000 ) ;
#83328=SURFACE_SIDE_STYLE ('',( #51418 ) ) ;
#83348=CARTESIAN_POINT ( 'NONE',  ( 11.15040314143522160, 7.934999999999988951, -2.126176841940961904 ) ) ;
#83378=FILL_AREA_STYLE_COLOUR ( '', #538 ) ;
#83419=EDGE_CURVE ( 'NONE', #119897, #93928, #13933, .T. ) ;
#83423=SURFACE_STYLE_USAGE ( .BOTH. , #114590 ) ;
#83434=( LENGTH_UNIT ( ) NAMED_UNIT ( * ) SI_UNIT ( .MILLI., .METRE. ) );
#83437=CARTESIAN_POINT ( 'NONE',  ( 180.5530070941699705, -49.14999999999999147, -40.56450646616441702 ) ) ;
#83444=COLOUR_RGB ( '', 0.31764706, 0.68627451, 0.89019608) ;
#83460=CARTESIAN_POINT ( 'NONE',  ( 2.625000000000000000, 6.094999999999989981, -1.119633336120465690E-15 ) ) ;
#83490=FILL_AREA_STYLE ('',( #29091 ) ) ;
#83499=FACE_OUTER_BOUND ( 'NONE', #41988, .T. ) ;
#83543=EDGE_CURVE ( 'NONE', #140063, #19565, #11249, .T. ) ;
#83564=( LENGTH_UNIT ( ) NAMED_UNIT ( * ) SI_UNIT ( .MILLI., .METRE. ) );
#83604=FILL_AREA_STYLE_COLOUR ( '', #21478 ) ;
#83607=CARTESIAN_POINT ( 'NONE',  ( 7.067069808101886785, 2.126176841940952134, -7.934999999999993392 ) ) ;
#83646=EDGE_CURVE ( 'NONE', #63837, #100283, #41551, .T. ) ;
#83647=CARTESIAN_POINT ( 'NONE',  ( 7.124569808101887780, -6.871911579029512218, 3.967499999999996252 ) ) ;
#83678=UNCERTAINTY_MEASURE_WITH_UNIT (LENGTH_MEASURE( 1.000000000000000082E-05 ), #33804, 'distance_accuracy_value', 'NONE');
#83705=MECHANICAL_DESIGN_GEOMETRIC_PRESENTATION_REPRESENTATION('',(#69843),#120695);
#83709=FACE_OUTER_BOUND ( 'NONE', #72339, .T. ) ;
#83745=AXIS2_PLACEMENT_3D ( 'NONE', #25686, #36565, #80810 ) ;
#83759=VECTOR ( 'NONE', #95014, 1000.000000000000000 ) ;
#83769=CARTESIAN_POINT ( 'NONE',  ( 180.4193221990229574, -49.14999999999999147, -40.92499999999998295 ) ) ;
#83781=CARTESIAN_POINT ( 'NONE',  ( 17.25413961620377279, 3.047499999999993214, -5.278424836066146320 ) ) ;
#83793=EDGE_LOOP ( 'NONE', ( #140969, #117044, #71070, #14546 ) ) ;
#83803=ORIENTED_EDGE ( 'NONE', *, *, #15131, .F. ) ;
#83820=CARTESIAN_POINT ( 'NONE',  ( 28.56206980810188512, -7.934999999999991616, -2.126176841940955242 ) ) ;
#83832=PRESENTATION_STYLE_ASSIGNMENT (( #46207 ) ) ;
#83853=ORIENTED_EDGE ( 'NONE', *, *, #38611, .F. ) ;
#83855=PRESENTATION_STYLE_ASSIGNMENT (( #127311 ) ) ;
#83866=CARTESIAN_POINT ( 'NONE',  ( 34.12500000000000000, 6.094999999999989981, -1.119633336120465690E-15 ) ) ;
#83870=ORIENTED_EDGE ( 'NONE', *, *, #76935, .F. ) ;
#83889=CYLINDRICAL_SURFACE ( 'NONE', #91111, 6.094999999999989093 ) ;
#83890=PRESENTATION_STYLE_ASSIGNMENT (( #117169 ) ) ;
#83904=( BOUNDED_CURVE ( )  B_SPLINE_CURVE ( 2, ( #50572, #6291, #84632, #138300, #140427, #71621, #18623, #83204, #127405, #95488, #128150, #73070, #51300 ),
 .UNSPECIFIED., .F., .F. ) 
 B_SPLINE_CURVE_WITH_KNOTS ( ( 3, 2, 2, 2, 2, 2, 3 ),
 ( 0.4000000000000001332, 0.4083333333333334370, 0.4166666666666667407, 0.4250000000000000444, 0.4333333333333334036, 0.4416666666666666519, 0.4500000000000000111 ),
 .UNSPECIFIED. ) 
 CURVE ( )  GEOMETRIC_REPRESENTATION_ITEM ( )  RATIONAL_B_SPLINE_CURVE ( ( 0.9999999999999995559, 0.9659258262890687563, 1.000000000000000000, 0.9659258262890683122, 1.000000000000000000, 0.9659258262890683122, 1.000000000000000000, 0.9659258262890683122, 1.000000000000000000, 0.9659258262890683122, 1.000000000000000000, 0.9659258262890683122, 1.000000000000000000 ) ) 
 REPRESENTATION_ITEM ( '' )  );
#83931=( GEOMETRIC_REPRESENTATION_CONTEXT ( 3 ) GLOBAL_UNCERTAINTY_ASSIGNED_CONTEXT ( ( #125742 ) ) GLOBAL_UNIT_ASSIGNED_CONTEXT ( ( #130108, #8277, #64132 ) ) REPRESENTATION_CONTEXT ( 'NONE', 'WORKASPACE' ) );
#83932=CARTESIAN_POINT ( 'NONE',  ( 25.39999999999999858, 1.399999999999986366, 20.40202195861970580 ) ) ;
#83937=COLOUR_RGB ( '', 0.09019608, 0.27058824, 0.51372549) ;
#83938=DIRECTION ( 'NONE',  ( 0.000000000000000000, 0.000000000000000000, 1.000000000000000000 ) ) ;
#83987=CARTESIAN_POINT ( 'NONE',  ( 7.124569808101886892, -6.871911579029512218, 3.967499999999996252 ) ) ;
#84002=VECTOR ( 'NONE', #5823, 1000.000000000000000 ) ;
#84014=CARTESIAN_POINT ( 'NONE',  ( 55.95337363913751716, -51.41954113333837739, -38.53170190052302502 ) ) ;
#84032=CARTESIAN_POINT ( 'NONE',  ( 31.77040314143522082, -7.934999999999989839, 2.126176841940957907 ) ) ;
#84033=CARTESIAN_POINT ( 'NONE',  ( 4.499569808101886004, -3.967499999999998028, -6.871911579029511330 ) ) ;
#84060=CARTESIAN_POINT ( 'NONE',  ( 61.46640106136305803, -43.15000000000002700, 34.92499999999998295 ) ) ;
#84065=( BOUNDED_CURVE ( )  B_SPLINE_CURVE ( 3, ( #12742, #125647, #15399, #43975 ),
 .UNSPECIFIED., .F., .T. ) 
 B_SPLINE_CURVE_WITH_KNOTS ( ( 4, 4 ),
 ( 0.1773996044403763073, 1.570796326794896558 ),
 .UNSPECIFIED. ) 
 CURVE ( )  GEOMETRIC_REPRESENTATION_ITEM ( )  RATIONAL_B_SPLINE_CURVE ( ( 1.000000000000000000, 0.8446433258982480874, 0.8446433258982480874, 1.000000000000000000 ) ) 
 REPRESENTATION_ITEM ( '' )  );
#84078=DIRECTION ( 'NONE',  ( -1.000000000000000000, -0.000000000000000000, -0.000000000000000000 ) ) ;
#84082=ORIENTED_EDGE ( 'NONE', *, *, #60565, .T. ) ;
#84089=CARTESIAN_POINT ( 'NONE',  ( 11.29623647476855375, 7.934999999999990727, -1.457635852685135314E-15 ) ) ;
#84159=CARTESIAN_POINT ( 'NONE',  ( 7.504569808101886785, 6.871911579029510442, -3.967499999999998916 ) ) ;
#84169=FACE_OUTER_BOUND ( 'NONE', #136509, .T. ) ;
#84172=CARTESIAN_POINT ( 'NONE',  ( 61.46640106136302961, -43.14999999999999147, -34.92499999999998295 ) ) ;
#84175=CARTESIAN_POINT ( 'NONE',  ( 184.1499999999998067, -49.85820393249934313, -34.92499999999997584 ) ) ;
#84193=DIRECTION ( 'NONE',  ( 0.000000000000000000, 1.000000000000000000, 4.625929269271485322E-15 ) ) ;
#84234=SURFACE_STYLE_FILL_AREA ( #143386 ) ;
#84295=ORIENTED_EDGE ( 'NONE', *, *, #66179, .T. ) ;
#84319=ORIENTED_EDGE ( 'NONE', *, *, #40922, .T. ) ;
#84327=CARTESIAN_POINT ( 'NONE',  ( 5.025403141435220711, 2.126176841940962348, 7.934999999999989839 ) ) ;
#84362=CARTESIAN_POINT ( 'NONE',  ( 14.12456980810188689, -6.871911579029512218, 3.967499999999996252 ) ) ;
#84394=DIRECTION ( 'NONE',  ( 0.000000000000000000, 0.000000000000000000, 1.000000000000000000 ) ) ;
#84485=CARTESIAN_POINT ( 'NONE',  ( 17.83747294953710494, 6.094999999999989981, -1.119633336120465690E-15 ) ) ;
#84515=( BOUNDED_SURFACE ( )  B_SPLINE_SURFACE ( 3, 2, ( 
 ( #11247, #63563, #8385 ),
 ( #52634, #53355, #41779 ),
 ( #85991, #130227, #130949 ),
 ( #9847, #54117, #98306 ) ),
 .UNSPECIFIED., .F., .F., .F. ) 
 B_SPLINE_SURFACE_WITH_KNOTS ( ( 4, 4 ),
 ( 3, 3 ),
 ( 0.000000000000000000, 0.001630001914283400570 ),
 ( 0.000000000000000000, 1.000000000000000000 ),
 .UNSPECIFIED. ) 
 GEOMETRIC_REPRESENTATION_ITEM ( )  RATIONAL_B_SPLINE_SURFACE ( (
 ( 1.000000000000000000, 0.7071067811865475727, 1.000000000000000000),
 ( 1.000000000000000000, 0.7121002461815034712, 1.000000000000000000),
 ( 1.000000000000000000, 0.7157206429707760886, 1.000000000000000000),
 ( 1.000000000000000000, 0.7180326832784531543, 1.000000000000000000) ) ) 
 REPRESENTATION_ITEM ( '' )  SURFACE ( )  );
#84517=CARTESIAN_POINT ( 'NONE',  ( 34.39540314143521016, 2.126176841940962348, 7.934999999999989839 ) ) ;
#84540=ORIENTED_EDGE ( 'NONE', *, *, #134827, .F. ) ;
#84560=( GEOMETRIC_REPRESENTATION_CONTEXT ( 3 ) GLOBAL_UNCERTAINTY_ASSIGNED_CONTEXT ( ( #17457 ) ) GLOBAL_UNIT_ASSIGNED_CONTEXT ( ( #68939, #121832, #55190 ) ) REPRESENTATION_CONTEXT ( 'NONE', 'WORKASPACE' ) );
#84581=CARTESIAN_POINT ( 'NONE',  ( 1.743167068800034469, -4.720063557702711243, 4.254651343200441360 ) ) ;
#84582=FILL_AREA_STYLE_COLOUR ( '', #60882 ) ;
#84632=CARTESIAN_POINT ( 'NONE',  ( 12.00413961620377279, -3.047499999999994547, 5.278424836066145431 ) ) ;
#84664=CARTESIAN_POINT ( 'NONE',  ( 128.9683591370938416, -52.14999999999999147, -41.64500000000001023 ) ) ;
#84666=CARTESIAN_POINT ( 'NONE',  ( 0.2480159638834371905, -51.74944211519454740, 38.65549799471352799 ) ) ;
#84668=CARTESIAN_POINT ( 'NONE',  ( 4.207903141435219929, -6.871911579029513106, -3.967499999999993587 ) ) ;
#84673=ORIENTED_EDGE ( 'NONE', *, *, #18839, .F. ) ;
#84678=DIRECTION ( 'NONE',  ( 0.000000000000000000, -1.000000000000000000, 0.000000000000000000 ) ) ;
#84710=CARTESIAN_POINT ( 'NONE',  ( 8.458333333333333925, -3.047499999999997211, -5.278424836066143655 ) ) ;
#84711=CARTESIAN_POINT ( 'NONE',  ( 3.187069808101886448, -2.126176841940956130, 7.934999999999990727 ) ) ;
#84727=CARTESIAN_POINT ( 'NONE',  ( 55.56056557994604361, -52.00875322212549179, -39.86617647058817937 ) ) ;
#84737=CARTESIAN_POINT ( 'NONE',  ( 56.45153347184072601, -50.67230138428463704, 37.61253110040618708 ) ) ;
#84740=STYLED_ITEM ( 'NONE', ( #40204 ), #108314 ) ;
#84746=CARTESIAN_POINT ( 'NONE',  ( 130.2059003229213658, -48.16486758952235903, 37.61253110040621550 ) ) ;
#84748=CARTESIAN_POINT ( 'NONE',  ( 7.000000000000000888, 0.000000000000000000, 6.094999999999989981 ) ) ;
#84758=CARTESIAN_POINT ( 'NONE',  ( 156.1499999999997783, -52.14999999999999147, 34.92500000000004690 ) ) ;
#84768=CARTESIAN_POINT ( 'NONE',  ( 5.900403141435219823, -7.934999999999988951, 2.126176841940957907 ) ) ;
#84776=ORIENTED_EDGE ( 'NONE', *, *, #30632, .T. ) ;
#84779=CARTESIAN_POINT ( 'NONE',  ( 18.08333333333333215, -5.278424836066144543, 3.047499999999995879 ) ) ;
#84781=ORIENTED_EDGE ( 'NONE', *, *, #11689, .F. ) ;
#84791=VERTEX_POINT ( 'NONE', #16893 ) ;
#84826=VECTOR ( 'NONE', #103455, 1000.000000000000000 ) ;
#84837=CARTESIAN_POINT ( 'NONE',  ( 11.87956980810188767, 3.967499999999998916, 6.871911579029510442 ) ) ;
#84846=FACE_OUTER_BOUND ( 'NONE', #56855, .T. ) ;
#84905=SURFACE_STYLE_FILL_AREA ( #140700 ) ;
#84959=CARTESIAN_POINT ( 'NONE',  ( 174.7500000000000000, 7.919999999999947526, -21.52769999999994965 ) ) ;
#84961=ORIENTED_EDGE ( 'NONE', *, *, #40496, .T. ) ;
#84981=STYLED_ITEM ( 'NONE', ( #123586 ), #13691 ) ;
#84998=CARTESIAN_POINT ( 'NONE',  ( 25.39999999999999858, -14.29000000000013593, 12.69999999999954632 ) ) ;
#84999=( NAMED_UNIT ( * ) PLANE_ANGLE_UNIT ( ) SI_UNIT ( $, .RADIAN. ) );
#85000=CARTESIAN_POINT ( 'NONE',  ( 20.04623647476855197, -7.934999999999990727, 4.858786175617117713E-16 ) ) ;
#85006=EDGE_CURVE ( 'NONE', #143110, #70428, #135301, .T. ) ;
#85035=CARTESIAN_POINT ( 'NONE',  ( 11.93706980810188689, 2.126176841940952134, -7.934999999999993392 ) ) ;
#85052=ORIENTED_EDGE ( 'NONE', *, *, #127825, .F. ) ;
#85095=SURFACE_STYLE_USAGE ( .BOTH. , #29993 ) ;
#85107=STYLED_ITEM ( 'NONE', ( #22886 ), #93057 ) ;
#85125=CIRCLE ( 'NONE', #38877, 28.00000000000002487 ) ;
#85162=CARTESIAN_POINT ( 'NONE',  ( 24.54580628287043709, 5.278424836066143655, -3.047499999999997655 ) ) ;
#85183=CIRCLE ( 'NONE', #22657, 8.094999999999991758 ) ;
#85194=CARTESIAN_POINT ( 'NONE',  ( 29.58290314143522082, 3.967499999999992699, -6.871911579029513994 ) ) ;
#85199=VERTEX_POINT ( 'NONE', #63806 ) ;
#85227=( NAMED_UNIT ( * ) PLANE_ANGLE_UNIT ( ) SI_UNIT ( $, .RADIAN. ) );
#85228=DIRECTION ( 'NONE',  ( 0.000000000000000000, -1.000000000000000000, 0.000000000000000000 ) ) ;
#85229=UNCERTAINTY_MEASURE_WITH_UNIT (LENGTH_MEASURE( 1.000000000000000082E-05 ), #73057, 'distance_accuracy_value', 'NONE');
#85276=MECHANICAL_DESIGN_GEOMETRIC_PRESENTATION_REPRESENTATION('',(#62131),#92210);
#85287=( NAMED_UNIT ( * ) PLANE_ANGLE_UNIT ( ) SI_UNIT ( $, .RADIAN. ) );
#85295=CARTESIAN_POINT ( 'NONE',  ( 181.0893910107582485, -48.47007572038052103, 38.12657027910874774 ) ) ;
#85349=AXIS2_PLACEMENT_3D ( 'NONE', #87670, #57215, #10788 ) ;
#85359=CARTESIAN_POINT ( 'NONE',  ( 5.812069808101887780, 7.934999999999993392, 2.126176841940951689 ) ) ;
#85385=CARTESIAN_POINT ( 'NONE',  ( 56.10188787153389711, -51.19676978474460327, -38.21513923099966092 ) ) ;
#85399=CARTESIAN_POINT ( 'NONE',  ( 8.604166666666667851, -1.633150327867691987, -6.094999999999989093 ) ) ;
#85400=CARTESIAN_POINT ( 'NONE',  ( 14.27040314143522082, -7.934999999999988951, 2.126176841940957907 ) ) ;
#85414=( GEOMETRIC_REPRESENTATION_CONTEXT ( 3 ) GLOBAL_UNCERTAINTY_ASSIGNED_CONTEXT ( ( #143354 ) ) GLOBAL_UNIT_ASSIGNED_CONTEXT ( ( #87968, #31452, #11081 ) ) REPRESENTATION_CONTEXT ( 'NONE', 'WORKASPACE' ) );
#85419=CARTESIAN_POINT ( 'NONE',  ( 0.1164707300447353766, -51.38852430739341770, 37.54101415799218699 ) ) ;
#85434=CARTESIAN_POINT ( 'NONE',  ( 125.9798776214791900, -48.09441802426615453, 35.89947574910151928 ) ) ;
#85436=CARTESIAN_POINT ( 'NONE',  ( 7.145833333333334814, -1.633150327867700202, 6.094999999999985540 ) ) ;
#85456=DIRECTION ( 'NONE',  ( -0.000000000000000000, -0.000000000000000000, -1.000000000000000000 ) ) ;
#85457=CARTESIAN_POINT ( 'NONE',  ( 20.04623647476855197, -7.934999999999990727, 4.858786175617117713E-16 ) ) ;
#85482=CARTESIAN_POINT ( 'NONE',  ( 25.40000000000000213, 2.120873585778977333, -7.657087335400156292 ) ) ;
#85483=DIRECTION ( 'NONE',  ( 0.000000000000000000, 0.000000000000000000, -1.000000000000000000 ) ) ;
#85490=ORIENTED_EDGE ( 'NONE', *, *, #11271, .T. ) ;
#85514=PRESENTATION_STYLE_ASSIGNMENT (( #7227 ) ) ;
#85522=CARTESIAN_POINT ( 'NONE',  ( 5.608736474768551972, -5.808823158059033709, 5.808823158059035485 ) ) ;
#85537=AXIS2_PLACEMENT_3D ( 'NONE', #86532, #87233, #97357 ) ;
#85541=CARTESIAN_POINT ( 'NONE',  ( 183.9820196591281842, -48.55783623716401820, -38.28685941347310973 ) ) ;
#85561=CIRCLE ( 'NONE', #62421, 2.552699999999990865 ) ;
#85568=CARTESIAN_POINT ( 'NONE',  ( 152.4000000000000057, -16.48000000000005016, 12.69999999999954632 ) ) ;
#85569=CARTESIAN_POINT ( 'NONE',  ( 0.1600000000000008915, -5.960583198795250226, -5.280645022235340491 ) ) ;
#85647=MECHANICAL_DESIGN_GEOMETRIC_PRESENTATION_REPRESENTATION('',(#44078),#125083);
#85648=LINE ( 'NONE', #9497, #37222 ) ;
#85689=ORIENTED_EDGE ( 'NONE', *, *, #110487, .F. ) ;
#85699=CARTESIAN_POINT ( 'NONE',  ( 22.81706980810188767, -2.126176841940956130, 7.934999999999991616 ) ) ;
#85704=( BOUNDED_CURVE ( )  B_SPLINE_CURVE ( 3, ( #84172, #3677, #71860, #39210 ),
 .UNSPECIFIED., .F., .T. ) 
 B_SPLINE_CURVE_WITH_KNOTS ( ( 4, 4 ),
 ( 4.712388980384689674, 6.105785702739209952 ),
 .UNSPECIFIED. ) 
 CURVE ( )  GEOMETRIC_REPRESENTATION_ITEM ( )  RATIONAL_B_SPLINE_CURVE ( ( 1.000000000000000000, 0.8446433258982480874, 0.8446433258982480874, 1.000000000000000000 ) ) 
 REPRESENTATION_ITEM ( '' )  );
#85709=ORIENTED_EDGE ( 'NONE', *, *, #36533, .F. ) ;
#85718=ORIENTED_EDGE ( 'NONE', *, *, #2153, .T. ) ;
#85741=CARTESIAN_POINT ( 'NONE',  ( 10.33290314143522082, -3.967499999999994476, 6.871911579029513106 ) ) ;
#85746=FILL_AREA_STYLE_COLOUR ( '', #92803 ) ;
#85748=CARTESIAN_POINT ( 'NONE',  ( 6.170806282870438864, -3.047499999999997211, -5.278424836066143655 ) ) ;
#85760=ORIENTED_EDGE ( 'NONE', *, *, #122336, .F. ) ;
#85775=LINE ( 'NONE', #95222, #65381 ) ;
#85776=EDGE_CURVE ( 'NONE', #17549, #59338, #12181, .T. ) ;
#85787=ORIENTED_EDGE ( 'NONE', *, *, #46347, .T. ) ;
#85792=( NAMED_UNIT ( * ) SI_UNIT ( $, .STERADIAN. ) SOLID_ANGLE_UNIT ( ) );
#85835=CIRCLE ( 'NONE', #41873, 5.999999999999998224 ) ;
#85883=CARTESIAN_POINT ( 'NONE',  ( 24.10830628287044419, 1.633150327867687324, -6.094999999999991758 ) ) ;
#85904=ORIENTED_EDGE ( 'NONE', *, *, #69663, .T. ) ;
#85906=COLOUR_RGB ( '', 0.31764706, 0.68627451, 0.89019608) ;
#85920=CARTESIAN_POINT ( 'NONE',  ( 31.91623647476855297, -7.934999999999990727, 4.858786175617117713E-16 ) ) ;
#85927=CARTESIAN_POINT ( 'NONE',  ( 55.38366852087742842, -49.19090614206224643, 40.79110616923198052 ) ) ;
#85956=DIRECTION ( 'NONE',  ( 0.000000000000000000, 0.000000000000000000, 1.000000000000000000 ) ) ;
#85959=DIRECTION ( 'NONE',  ( -1.000000000000000000, -0.000000000000000000, -0.000000000000000000 ) ) ;
#85972=CARTESIAN_POINT ( 'NONE',  ( 28.58333333333333570, -5.278424836066144543, 3.047499999999995879 ) ) ;
#85991=CARTESIAN_POINT ( 'NONE',  ( 128.6956467655712117, -52.10358567238988314, -40.45860062938062640 ) ) ;
#85998=COLOUR_RGB ( '', 0.40784314, 0.44705882, 0.49803922) ;
#86016=ORIENTED_EDGE ( 'NONE', *, *, #60183, .F. ) ;
#86018=ADVANCED_FACE ( 'NONE', ( #101231, #69343, #136712 ), #91781, .F. ) ;
#86035=CARTESIAN_POINT ( 'NONE',  ( 183.9820196591358012, -48.55783623716212105, 38.28685941347691113 ) ) ;
#86046=DIRECTION ( 'NONE',  ( 0.000000000000000000, 0.000000000000000000, -1.000000000000000000 ) ) ;
#86051=EDGE_CURVE ( 'NONE', #81376, #111873, #114017, .T. ) ;
#86054=VECTOR ( 'NONE', #18590, 1000.000000000000000 ) ;
#86068=PRESENTATION_STYLE_ASSIGNMENT (( #41849 ) ) ;
#86083=ORIENTED_EDGE ( 'NONE', *, *, #3010, .T. ) ;
#86097=CARTESIAN_POINT ( 'NONE',  ( 0.4162364747685527444, -7.934999999999990727, 4.858786175617117713E-16 ) ) ;
#86119=MECHANICAL_DESIGN_GEOMETRIC_PRESENTATION_REPRESENTATION('',(#18956),#137027);
#86141=DIRECTION ( 'NONE',  ( -0.000000000000000000, -1.000000000000000000, 0.000000000000000000 ) ) ;
#86142=CARTESIAN_POINT ( 'NONE',  ( 7.000000000000000888, 0.000000000000000000, 6.094999999999989981 ) ) ;
#86143=CARTESIAN_POINT ( 'NONE',  ( 21.41623647476855652, -7.934999999999990727, 4.858786175617117713E-16 ) ) ;
#86151=MECHANICAL_DESIGN_GEOMETRIC_PRESENTATION_REPRESENTATION('',(#30591),#111601);
#86166=CARTESIAN_POINT ( 'NONE',  ( 0.6713702758572441809, -52.14999999999999147, 41.05044666116288710 ) ) ;
#86170=( NAMED_UNIT ( * ) SI_UNIT ( $, .STERADIAN. ) SOLID_ANGLE_UNIT ( ) );
#86179=CARTESIAN_POINT ( 'NONE',  ( 129.2310344399266171, -47.51495700085919083, 36.79359617903138258 ) ) ;
#86202=CARTESIAN_POINT ( 'NONE',  ( 16.69206980810188767, -7.934999999999990727, -2.126176841940955242 ) ) ;
#86232=( LENGTH_UNIT ( ) NAMED_UNIT ( * ) SI_UNIT ( .MILLI., .METRE. ) );
#86234=CARTESIAN_POINT ( 'NONE',  ( 25.40000000000001279, 6.400415038920557187, -4.708210710744500815 ) ) ;
#86255=AXIS2_PLACEMENT_3D ( 'NONE', #27778, #5289, #93758 ) ;
#86280=CARTESIAN_POINT ( 'NONE',  ( 12.17123647476855375, 0.000000000000000000, 7.934999999999990727 ) ) ;
#86288=ORIENTED_EDGE ( 'NONE', *, *, #136879, .T. ) ;
#86304=AXIS2_PLACEMENT_3D ( 'NONE', #20721, #133099, #33781 ) ;
#86306=EDGE_LOOP ( 'NONE', ( #136332, #59740, #127697 ) ) ;
#86307=CARTESIAN_POINT ( 'NONE',  ( 0.8183591370940799248, -52.14999999999999147, -41.64500000000001023 ) ) ;
#86310=ORIENTED_EDGE ( 'NONE', *, *, #126192, .F. ) ;
#86326=( GEOMETRIC_REPRESENTATION_CONTEXT ( 3 ) GLOBAL_UNCERTAINTY_ASSIGNED_CONTEXT ( ( #94125 ) ) GLOBAL_UNIT_ASSIGNED_CONTEXT ( ( #78129, #57108, #54952 ) ) REPRESENTATION_CONTEXT ( 'NONE', 'WORKASPACE' ) );
#86386=PRESENTATION_STYLE_ASSIGNMENT (( #55179 ) ) ;
#86393=EDGE_CURVE ( 'NONE', #6561, #93928, #37765, .T. ) ;
#86412=CARTESIAN_POINT ( 'NONE',  ( 3.345840036506269488, -49.02495722182847260, 39.69341335395905190 ) ) ;
#86439=ORIENTED_EDGE ( 'NONE', *, *, #52929, .F. ) ;
#86451=DIRECTION ( 'NONE',  ( 0.000000000000000000, 0.000000000000000000, 1.000000000000000000 ) ) ;
#86452=CARTESIAN_POINT ( 'NONE',  ( 13.92123647476855197, -9.717572351234235426E-16, -7.934999999999990727 ) ) ;
#86475=EDGE_LOOP ( 'NONE', ( #62531, #23018, #35138, #120675, #116770, #133500, #73180, #13068 ) ) ;
#86476=CARTESIAN_POINT ( 'NONE',  ( 5.104166666666668739, -1.633150327867687102, -6.094999999999992646 ) ) ;
#86480=ORIENTED_EDGE ( 'NONE', *, *, #126945, .T. ) ;
#86484=CARTESIAN_POINT ( 'NONE',  ( 9.895403141435220817, 2.126176841940962348, 7.934999999999989839 ) ) ;
#86490=CYLINDRICAL_SURFACE ( 'NONE', #16415, 2.552699999999959779 ) ;
#86492=CARTESIAN_POINT ( 'NONE',  ( 5.733306282870439752, -6.094999999999989981, -1.633150327867689322 ) ) ;
#86531=CIRCLE ( 'NONE', #56457, 3.000000000000000000 ) ;
#86532=CARTESIAN_POINT ( 'NONE',  ( 61.46640106136302961, -57.15000000000009805, -40.92499999999998295 ) ) ;
#86569=FILL_AREA_STYLE_COLOUR ( '', #74579 ) ;
#86570=VERTEX_POINT ( 'NONE', #104634 ) ;
#86629=CARTESIAN_POINT ( 'NONE',  ( 29.50413961620377279, -3.047499999999994547, 5.278424836066145431 ) ) ;
#86641=ORIENTED_EDGE ( 'NONE', *, *, #34298, .T. ) ;
#86657=DIRECTION ( 'NONE',  ( -1.000000000000000000, -0.000000000000000000, -0.000000000000000000 ) ) ;
#86665=CARTESIAN_POINT ( 'NONE',  ( 122.6835989386367771, -57.15000000000009805, -40.92499999999998295 ) ) ;
#86678=CARTESIAN_POINT ( 'NONE',  ( 122.6835989386367345, -43.14999999999999147, 34.92499999999998295 ) ) ;
#86764=CARTESIAN_POINT ( 'NONE',  ( 181.1395720402183258, -48.08977582060966682, 37.49964900842703486 ) ) ;
#86793=COLOUR_RGB ( '', 0.31764706, 0.68627451, 0.89019608) ;
#86816=CARTESIAN_POINT ( 'NONE',  ( 12.52040314143522082, 7.934999999999989839, -2.126176841940961904 ) ) ;
#86851=UNCERTAINTY_MEASURE_WITH_UNIT (LENGTH_MEASURE( 1.000000000000000082E-05 ), #47663, 'distance_accuracy_value', 'NONE');
#86863=CARTESIAN_POINT ( 'NONE',  ( 9.479166666666666075, 6.094999999999988205, -1.633150327867694651 ) ) ;
#86864=CARTESIAN_POINT ( 'NONE',  ( 20.10373647476855297, 5.808823158059035485, 5.808823158059032821 ) ) ;
#86885=CYLINDRICAL_SURFACE ( 'NONE', #98494, 6.094999999999989093 ) ;
#86910=EDGE_CURVE ( 'NONE', #60012, #117767, #16950, .T. ) ;
#86917=CARTESIAN_POINT ( 'NONE',  ( 17.27540314143521627, -2.126176841940958351, -7.934999999999988951 ) ) ;
#86952=PLANE ( 'NONE',  #27680 ) ;
#86958=DIRECTION ( 'NONE',  ( -0.000000000000000000, -0.000000000000000000, 1.000000000000000000 ) ) ;
#86974=CARTESIAN_POINT ( 'NONE',  ( 7.067069808101886785, 2.126176841940952134, -7.934999999999993392 ) ) ;
#86980=CARTESIAN_POINT ( 'NONE',  ( 55.38366852087663972, -49.19090614207205192, -40.79110616922474719 ) ) ;
#87009=UNCERTAINTY_MEASURE_WITH_UNIT (LENGTH_MEASURE( 1.000000000000000082E-05 ), #60137, 'distance_accuracy_value', 'NONE');
#87018=CARTESIAN_POINT ( 'NONE',  ( 0.1600000000000026401, -9.717572351234235426E-16, -7.934999999999990727 ) ) ;
#87076=CARTESIAN_POINT ( 'NONE',  ( 2.999999999999999112, -5.520864266206504263E-14, 0.000000000000000000 ) ) ;
#87086=SURFACE_SIDE_STYLE ('',( #31985 ) ) ;
#87111=CARTESIAN_POINT ( 'NONE',  ( 24.39997294953710494, 4.461849672132297329, -4.461849672132302658 ) ) ;
#87138=CARTESIAN_POINT ( 'NONE',  ( 20.02497294953710849, -4.461849672132299993, -4.461849672132299105 ) ) ;
#87149=CARTESIAN_POINT ( 'NONE',  ( 16.98373647476855197, -5.808823158059035485, -5.808823158059033709 ) ) ;
#87192=CARTESIAN_POINT ( 'NONE',  ( 5.149972949537104938, -4.461849672132299105, 4.461849672132299993 ) ) ;
#87233=DIRECTION ( 'NONE',  ( 0.000000000000000000, 1.000000000000000000, -2.556434596176436916E-15 ) ) ;
#87240=DIRECTION ( 'NONE',  ( 0.000000000000000000, 0.000000000000000000, 1.000000000000000000 ) ) ;
#87255=FACE_OUTER_BOUND ( 'NONE', #77723, .T. ) ;
#87268=COLOUR_RGB ( '', 0.08235294, 0.09019608, 0.10196078) ;
#87277=DIRECTION ( 'NONE',  ( -1.000000000000000000, -0.000000000000000000, -0.000000000000000000 ) ) ;
#87322=VECTOR ( 'NONE', #8687, 1000.000000000000000 ) ;
#87327=CARTESIAN_POINT ( 'NONE',  ( 21.04580628287044064, 5.278424836066143655, -3.047499999999997655 ) ) ;
#87345=ORIENTED_EDGE ( 'NONE', *, *, #105372, .T. ) ;
#87369=SURFACE_STYLE_USAGE ( .BOTH. , #98246 ) ;
#87383=COLOUR_RGB ( '', 0.40784314, 0.44705882, 0.49803922) ;
#87403=CARTESIAN_POINT ( 'NONE',  ( 16.23330628287043353, -6.094999999999989981, -1.633150327867689322 ) ) ;
#87409=MECHANICAL_DESIGN_GEOMETRIC_PRESENTATION_REPRESENTATION('',(#131377),#82743);
#87420=ADVANCED_FACE ( 'NONE', ( #70460 ), #70395, .T. ) ;
#87432=( LENGTH_UNIT ( ) NAMED_UNIT ( * ) SI_UNIT ( .MILLI., .METRE. ) );
#87437=MECHANICAL_DESIGN_GEOMETRIC_PRESENTATION_REPRESENTATION('',(#131410),#112970);
#87461=CARTESIAN_POINT ( 'NONE',  ( 181.0878408821075709, -48.47815212813055297, 38.14157743968410585 ) ) ;
#87465=PRESENTATION_STYLE_ASSIGNMENT (( #133126 ) ) ;
#87473=SURFACE_STYLE_USAGE ( .BOTH. , #96864 ) ;
#87517=VERTEX_POINT ( 'NONE', #8663 ) ;
#87522=CARTESIAN_POINT ( 'NONE',  ( 12.81206980810188512, 7.934999999999993392, 2.126176841940951689 ) ) ;
#87531=DIRECTION ( 'NONE',  ( 0.000000000000000000, 0.000000000000000000, -1.000000000000000000 ) ) ;
#87546=CARTESIAN_POINT ( 'NONE',  ( 18.42080628287044064, 3.047499999999997655, 5.278424836066143655 ) ) ;
#87558=DIRECTION ( 'NONE',  ( 0.000000000000000000, 0.000000000000000000, -1.000000000000000000 ) ) ;
#87566=CARTESIAN_POINT ( 'NONE',  ( 2.625000000000000000, 6.094999999999989981, -1.119633336120465690E-15 ) ) ;
#87567=CARTESIAN_POINT ( 'NONE',  ( 21.12456980810188867, -6.871911579029512218, 3.967499999999996252 ) ) ;
#87579=( LENGTH_UNIT ( ) NAMED_UNIT ( * ) SI_UNIT ( .MILLI., .METRE. ) );
#87581=SURFACE_STYLE_FILL_AREA ( #27656 ) ;
#87593=DIRECTION ( 'NONE',  ( -0.000000000000000000, 5.559056632600921604E-15, -1.000000000000000000 ) ) ;
#87602=CARTESIAN_POINT ( 'NONE',  ( 127.4973405139117659, -50.37061236291226152, 37.32649486623495960 ) ) ;
#87615=CIRCLE ( 'NONE', #57528, 5.999999999999998224 ) ;
#87623=CARTESIAN_POINT ( 'NONE',  ( 162.1604124744595481, 26.96999999999993491, 34.79688855774463008 ) ) ;
#87649=SURFACE_SIDE_STYLE ('',( #1327 ) ) ;
#87670=CARTESIAN_POINT ( 'NONE',  ( 26.40000000000000568, -16.48000000000005016, -33.92499999999998295 ) ) ;
#87682=ORIENTED_EDGE ( 'NONE', *, *, #110730, .T. ) ;
#87688=CARTESIAN_POINT ( 'NONE',  ( 23.54623647476855552, -7.934999999999990727, 4.858786175617117713E-16 ) ) ;
#87724=MECHANICAL_DESIGN_GEOMETRIC_PRESENTATION_REPRESENTATION('',(#101571),#38777);
#87732=CARTESIAN_POINT ( 'NONE',  ( 0.1600000000000024458, -7.375232382467828529, -3.003213012813335858 ) ) ;
#87733=CARTESIAN_POINT ( 'NONE',  ( 3.208333333333333481, 3.047499999999997655, 5.278424836066143655 ) ) ;
#87761=DIRECTION ( 'NONE',  ( 0.000000000000000000, 0.000000000000000000, -1.000000000000000000 ) ) ;
#87764=CARTESIAN_POINT ( 'NONE',  ( 23.77083333333333570, 6.094999999999991758, 1.633150327867686880 ) ) ;
#87803=AXIS2_PLACEMENT_3D ( 'NONE', #71813, #29003, #105127 ) ;
#87823=ADVANCED_FACE ( 'NONE', ( #115836 ), #114441, .T. ) ;
#87837=CARTESIAN_POINT ( 'NONE',  ( 52.60764783923753640, -52.00875322212549179, -39.33676470588228113 ) ) ;
#87852=CARTESIAN_POINT ( 'NONE',  ( 165.4843069612475119, 26.96999999999994202, -33.83501209545872968 ) ) ;
#87861=CARTESIAN_POINT ( 'NONE',  ( 18.87956980810189123, 3.967499999999998916, 6.871911579029510442 ) ) ;
#87874=CARTESIAN_POINT ( 'NONE',  ( 128.5894344200537773, -52.00875322212549179, -39.86617647058817226 ) ) ;
#87947=CARTESIAN_POINT ( 'NONE',  ( 25.39999999999999858, -7.600000000000061817, 28.92499999999998650 ) ) ;
#87959=CARTESIAN_POINT ( 'NONE',  ( 8.941639616203772789, -6.094999999999989093, 1.633150327867691542 ) ) ;
#87968=( LENGTH_UNIT ( ) NAMED_UNIT ( * ) SI_UNIT ( .MILLI., .METRE. ) );
#87992=DIRECTION ( 'NONE',  ( 0.000000000000000000, -2.556434596176436521E-15, -1.000000000000000000 ) ) ;
#88010=CARTESIAN_POINT ( 'NONE',  ( 25.39999999999999858, -1.600000000000012301, -20.40202195861969514 ) ) ;
#88021=DIRECTION ( 'NONE',  ( 0.000000000000000000, 0.000000000000000000, 1.000000000000000000 ) ) ;
#88022=TOROIDAL_SURFACE ( 'NONE', #16163, 2.000000000000000000, 1.000000000000000000 ) ;
#88036=CARTESIAN_POINT ( 'NONE',  ( 27.31663961620377634, -1.633150327867691987, -6.094999999999989093 ) ) ;
#88075=COLOUR_RGB ( '', 0.09019608, 0.27058824, 0.51372549) ;
#88109=UNCERTAINTY_MEASURE_WITH_UNIT (LENGTH_MEASURE( 1.000000000000000082E-05 ), #116066, 'distance_accuracy_value', 'NONE');
#88119=CARTESIAN_POINT ( 'NONE',  ( 174.7500000000000000, 7.919999999999947526, 21.67769999999990915 ) ) ;
#88124=AXIS2_PLACEMENT_3D ( 'NONE', #1322, #133313, #46326 ) ;
#88135=AXIS2_PLACEMENT_3D ( 'NONE', #55161, #10202, #122533 ) ;
#88140=( LENGTH_UNIT ( ) NAMED_UNIT ( * ) SI_UNIT ( .MILLI., .METRE. ) );
#88146=SURFACE_SIDE_STYLE ('',( #43926 ) ) ;
#88216=CARTESIAN_POINT ( 'NONE',  ( -2.141693717129561136, -1.633150327867689988, 6.094999999999989981 ) ) ;
#88242=CARTESIAN_POINT ( 'NONE',  ( 8.728736474768551190, 5.808823158059031044, -5.808823158059038150 ) ) ;
#88251=DIRECTION ( 'NONE',  ( 0.000000000000000000, -1.000000000000000000, 0.000000000000000000 ) ) ;
#88257=CONICAL_SURFACE ( 'NONE', #95171, 2.552699999999928693, 1.029744258676634772 ) ;
#88258=AXIS2_PLACEMENT_3D ( 'NONE', #66586, #121647, #68743 ) ;
#88277=ORIENTED_EDGE ( 'NONE', *, *, #110487, .T. ) ;
#88281=UNCERTAINTY_MEASURE_WITH_UNIT (LENGTH_MEASURE( 1.000000000000000082E-05 ), #66192, 'distance_accuracy_value', 'NONE');
#88286=AXIS2_PLACEMENT_3D ( 'NONE', #89339, #111814, #67623 ) ;
#88291=CARTESIAN_POINT ( 'NONE',  ( 17.93750000000000355, -4.461849672132299105, 4.461849672132299993 ) ) ;
#88293=CARTESIAN_POINT ( 'NONE',  ( 13.83290314143522082, -3.967499999999994476, 6.871911579029513106 ) ) ;
#88336=CARTESIAN_POINT ( 'NONE',  ( 183.4786297241425927, -52.14999999999999147, 41.05044666116288710 ) ) ;
#88410=AXIS2_PLACEMENT_3D ( 'NONE', #122461, #67414, #10142 ) ;
#88424=ADVANCED_FACE ( 'NONE', ( #25473 ), #126128, .T. ) ;
#88425=CARTESIAN_POINT ( 'NONE',  ( 22.37956980810188767, 3.967499999999998916, 6.871911579029510442 ) ) ;
#88442=CARTESIAN_POINT ( 'NONE',  ( 21.00000000000000000, 0.000000000000000000, 6.094999999999989981 ) ) ;
#88467=CARTESIAN_POINT ( 'NONE',  ( 20.54123647476855652, 0.000000000000000000, 7.934999999999990727 ) ) ;
#88490=ORIENTED_EDGE ( 'NONE', *, *, #48244, .T. ) ;
#88497=CARTESIAN_POINT ( 'NONE',  ( 156.1500000000000057, -57.14999999999999147, -45.92499999999969162 ) ) ;
#88505=ADVANCED_FACE ( 'NONE', ( #77931 ), #13873, .T. ) ;
#88507=DIRECTION ( 'NONE',  ( 0.000000000000000000, 0.000000000000000000, -1.000000000000000000 ) ) ;
#88525=DIRECTION ( 'NONE',  ( 0.000000000000000000, 0.000000000000000000, -1.000000000000000000 ) ) ;
#88557=CARTESIAN_POINT ( 'NONE',  ( 25.39999999999999858, -5.131256043349313067, -6.052638797879072108 ) ) ;
#88578=AXIS2_PLACEMENT_3D ( 'NONE', #46184, #90358, #14227 ) ;
#88598=CARTESIAN_POINT ( 'NONE',  ( 30.40040314143521982, -7.934999999999989839, 2.126176841940957907 ) ) ;
#88610=DIRECTION ( 'NONE',  ( -0.000000000000000000, 1.000000000000000000, 2.921639538487157626E-15 ) ) ;
#88616=ORIENTED_EDGE ( 'NONE', *, *, #33062, .F. ) ;
#88684=ORIENTED_EDGE ( 'NONE', *, *, #54675, .F. ) ;
#88685=CARTESIAN_POINT ( 'NONE',  ( 0.1600000000000007527, 2.771266204237592845, -7.457137036566489741 ) ) ;
#88699=SURFACE_STYLE_USAGE ( .BOTH. , #126133 ) ;
#88724=STYLED_ITEM ( 'NONE', ( #59204 ), #80703 ) ;
#88728=CARTESIAN_POINT ( 'NONE',  ( 181.1500000000000057, -3.180000000000061444, 34.92499999999998295 ) ) ;
#88770=CARTESIAN_POINT ( 'NONE',  ( 30.08747294953710494, -6.094999999999989981, 3.732111120401553285E-16 ) ) ;
#88779=CARTESIAN_POINT ( 'NONE',  ( 2.999999999999999112, -1.600000000000094458, 31.92499999999998295 ) ) ;
#88799=SURFACE_STYLE_USAGE ( .BOTH. , #307 ) ;
#88802=FACE_OUTER_BOUND ( 'NONE', #138252, .T. ) ;
#88811=DIRECTION ( 'NONE',  ( 0.1737853339090460192, -0.1737853339090456029, 0.9693282805305141192 ) ) ;
#88930=CARTESIAN_POINT ( 'NONE',  ( 2.962472949537105826, -7.464222240803106570E-16, -6.094999999999989981 ) ) ;
#88969=CARTESIAN_POINT ( 'NONE',  ( 9.020403141435219041, 7.934999999999989839, -2.126176841940961904 ) ) ;
#89017=CARTESIAN_POINT ( 'NONE',  ( 16.91666666666666785, 5.278424836066147208, 3.047499999999990550 ) ) ;
#89093=LINE ( 'NONE', #47066, #122168 ) ;
#89109=AXIS2_PLACEMENT_3D ( 'NONE', #6998, #40415, #94047 ) ;
#89126=CARTESIAN_POINT ( 'NONE',  ( 14.77497294953710494, 4.461849672132300881, 4.461849672132299105 ) ) ;
#89134=CARTESIAN_POINT ( 'NONE',  ( 23.69206980810188057, -7.934999999999991616, -2.126176841940955242 ) ) ;
#89171=ADVANCED_FACE ( 'NONE', ( #30317 ), #74556, .F. ) ;
#89173=CARTESIAN_POINT ( 'NONE',  ( 19.22873647476855652, 5.808823158059031044, -5.808823158059038150 ) ) ;
#89222=LINE ( 'NONE', #133444, #32303 ) ;
#89244=( LENGTH_UNIT ( ) NAMED_UNIT ( * ) SI_UNIT ( .MILLI., .METRE. ) );
#89249=DIRECTION ( 'NONE',  ( -0.2399999999999972433, 3.469446951953571048E-17, -0.9707728879609286432 ) ) ;
#89280=ORIENTED_EDGE ( 'NONE', *, *, #39622, .F. ) ;
#89286=ORIENTED_EDGE ( 'NONE', *, *, #37132, .F. ) ;
#89290=CARTESIAN_POINT ( 'NONE',  ( 32.00456980810188412, 6.871911579029510442, -3.967499999999998916 ) ) ;
#89306=CARTESIAN_POINT ( 'NONE',  ( 122.6835989386367771, -43.14999999999999147, -34.92499999999998295 ) ) ;
#89339=CARTESIAN_POINT ( 'NONE',  ( 153.4000000000000057, 25.96999999999993847, 34.92499999999998295 ) ) ;
#89342=CARTESIAN_POINT ( 'NONE',  ( 1.292751919595855004, -3.287470007381915860, -5.962884502238249951 ) ) ;
#89354=PRESENTATION_STYLE_ASSIGNMENT (( #100935 ) ) ;
#89356=CARTESIAN_POINT ( 'NONE',  ( 0.5043781857168800897, 7.083145261826254035, -2.736640815332766596 ) ) ;
#89407=SHAPE_REPRESENTATION_RELATIONSHIP ( 'NONE' , 'NONE' ,  #40289, #18911 ) ;
#89420=ORIENTED_EDGE ( 'NONE', *, *, #83646, .F. ) ;
#89423=ORIENTED_EDGE ( 'NONE', *, *, #124796, .F. ) ;
#89452=FILL_AREA_STYLE_COLOUR ( '', #56290 ) ;
#89453=CARTESIAN_POINT ( 'NONE',  ( 32.56663961620377989, 1.633150327867695095, 6.094999999999988205 ) ) ;
#89473=SURFACE_STYLE_FILL_AREA ( #133709 ) ;
#89488=( NAMED_UNIT ( * ) SI_UNIT ( $, .STERADIAN. ) SOLID_ANGLE_UNIT ( ) );
#89491=VERTEX_POINT ( 'NONE', #39630 ) ;
#89497=SURFACE_STYLE_USAGE ( .BOTH. , #124981 ) ;
#89508=CYLINDRICAL_SURFACE ( 'NONE', #139098, 5.999999999999998224 ) ;
#89525=UNCERTAINTY_MEASURE_WITH_UNIT (LENGTH_MEASURE( 1.000000000000000082E-05 ), #61011, 'distance_accuracy_value', 'NONE');
#89580=DIRECTION ( 'NONE',  ( 0.000000000000000000, -5.559056632600921604E-15, 1.000000000000000000 ) ) ;
#89583=DIRECTION ( 'NONE',  ( -0.000000000000000000, 1.000000000000000000, -0.000000000000000000 ) ) ;
#89590=VERTEX_POINT ( 'NONE', #106250 ) ;
#89598=CARTESIAN_POINT ( 'NONE',  ( 4.566639616203773677, 1.633150327867685103, 6.094999999999992646 ) ) ;
#89605=CARTESIAN_POINT ( 'NONE',  ( 25.39999999999999858, -43.14999999999999147, 40.92499999999998295 ) ) ;
#89625=CARTESIAN_POINT ( 'NONE',  ( 8.504139616203772789, -3.047499999999994547, 5.278424836066145431 ) ) ;
#89632=( GEOMETRIC_REPRESENTATION_CONTEXT ( 3 ) GLOBAL_UNCERTAINTY_ASSIGNED_CONTEXT ( ( #63850 ) ) GLOBAL_UNIT_ASSIGNED_CONTEXT ( ( #46762, #45311, #135170 ) ) REPRESENTATION_CONTEXT ( 'NONE', 'WORKASPACE' ) );
#89642=EDGE_LOOP ( 'NONE', ( #6160, #58650 ) ) ;
#89647=CIRCLE ( 'NONE', #55007, 1.000000000000000888 ) ;
#89653=CARTESIAN_POINT ( 'NONE',  ( 12.66623647476855297, 7.934999999999990727, -1.457635852685135314E-15 ) ) ;
#89654=DIRECTION ( 'NONE',  ( 1.000000000000000000, 0.000000000000000000, -0.000000000000000000 ) ) ;
#89662=CARTESIAN_POINT ( 'NONE',  ( 19.39583333333333570, 1.633150327867706864, -6.094999999999981100 ) ) ;
#89678=ORIENTED_EDGE ( 'NONE', *, *, #27897, .T. ) ;
#89683=STYLED_ITEM ( 'NONE', ( #87465 ), #112081 ) ;
#89687=VERTEX_POINT ( 'NONE', #68520 ) ;
#89688=CARTESIAN_POINT ( 'NONE',  ( 151.4000000000000057, -17.48000000000005016, -33.92499999999998295 ) ) ;
#89695=FILL_AREA_STYLE_COLOUR ( '', #101790 ) ;
#89698=FACE_OUTER_BOUND ( 'NONE', #44080, .T. ) ;
#89701=CARTESIAN_POINT ( 'NONE',  ( 10.93750000000000178, -4.461849672132299105, 4.461849672132299993 ) ) ;
#89713=DIRECTION ( 'NONE',  ( -1.000000000000000000, -0.000000000000000000, -0.000000000000000000 ) ) ;
#89756=CARTESIAN_POINT ( 'NONE',  ( 184.1500000000000057, -30.18000000000009564, -12.70000000000045404 ) ) ;
#89771=CARTESIAN_POINT ( 'NONE',  ( 26.40000000000000568, -16.48000000000005016, -34.92499999999998295 ) ) ;
#89778=EDGE_CURVE ( 'NONE', #68985, #62041, #30568, .T. ) ;
#89815=STYLED_ITEM ( 'NONE', ( #58838 ), #5117 ) ;
#89820=CARTESIAN_POINT ( 'NONE',  ( 22.96290314143522338, -3.967499999999994476, 6.871911579029513106 ) ) ;
#89849=( NAMED_UNIT ( * ) SI_UNIT ( $, .STERADIAN. ) SOLID_ANGLE_UNIT ( ) );
#89850=UNCERTAINTY_MEASURE_WITH_UNIT (LENGTH_MEASURE( 1.000000000000000082E-05 ), #3278, 'distance_accuracy_value', 'NONE');
#89861=DIRECTION ( 'NONE',  ( 0.000000000000000000, -5.559056632600921604E-15, 1.000000000000000000 ) ) ;
#89862=CARTESIAN_POINT ( 'NONE',  ( 18.79123647476855652, -9.717572351234235426E-16, -7.934999999999990727 ) ) ;
#89863=CARTESIAN_POINT ( 'NONE',  ( 2.895403141435219485, 2.126176841940962348, 7.934999999999988951 ) ) ;
#89884=EDGE_CURVE ( 'NONE', #68280, #15118, #47412, .T. ) ;
#89921=CARTESIAN_POINT ( 'NONE',  ( 3.858736474768553304, 5.808823158059031044, -5.808823158059037262 ) ) ;
#89930=SURFACE_SIDE_STYLE ('',( #102275 ) ) ;
#89960=( LENGTH_UNIT ( ) NAMED_UNIT ( * ) SI_UNIT ( .MILLI., .METRE. ) );
#89984=CARTESIAN_POINT ( 'NONE',  ( 26.75456980810189123, -6.871911579029512218, 3.967499999999996252 ) ) ;
#89990=DIRECTION ( 'NONE',  ( -1.000000000000000000, -0.000000000000000000, -0.000000000000000000 ) ) ;
#89996=AXIS2_PLACEMENT_3D ( 'NONE', #17662, #59270, #107543 ) ;
#90015=ORIENTED_EDGE ( 'NONE', *, *, #27226, .F. ) ;
#90031=DIRECTION ( 'NONE',  ( 0.2399999999999954947, 0.000000000000000000, -0.9707728879609288652 ) ) ;
#90042=CARTESIAN_POINT ( 'NONE',  ( 1.529293640529030496, -1.216522783188787482, -6.459157641439147390 ) ) ;
#90045=CARTESIAN_POINT ( 'NONE',  ( 25.39999999999999858, 7.568741776763671325, 1.931219224265529055 ) ) ;
#90075=( LENGTH_UNIT ( ) NAMED_UNIT ( * ) SI_UNIT ( .MILLI., .METRE. ) );
#90084=MECHANICAL_DESIGN_GEOMETRIC_PRESENTATION_REPRESENTATION('',(#9009),#57632);
#90127=AXIS2_PLACEMENT_3D ( 'NONE', #98287, #75823, #106995 ) ;
#90163=CARTESIAN_POINT ( 'NONE',  ( 2.546236474768552860, -7.934999999999990727, 4.858786175617117713E-16 ) ) ;
#90173=PRESENTATION_STYLE_ASSIGNMENT (( #67763 ) ) ;
#90180=( LENGTH_UNIT ( ) NAMED_UNIT ( * ) SI_UNIT ( .MILLI., .METRE. ) );
#90202=AXIS2_PLACEMENT_3D ( 'NONE', #32815, #74900, #31369 ) ;
#90207=CARTESIAN_POINT ( 'NONE',  ( 2.999999999999999112, -7.600000000000055600, -28.92499999999998650 ) ) ;
#90242=MANIFOLD_SOLID_BREP ( 'Fillet5', #113437 ) ;
#90251=VERTEX_POINT ( 'NONE', #137157 ) ;
#90263=( LENGTH_UNIT ( ) NAMED_UNIT ( * ) SI_UNIT ( .MILLI., .METRE. ) );
#90329=COLOUR_RGB ( '', 0.09019608, 0.27058824, 0.51372549) ;
#90336=CARTESIAN_POINT ( 'NONE',  ( 6.316639616203774565, -1.633150327867691987, -6.094999999999989093 ) ) ;
#90358=DIRECTION ( 'NONE',  ( -1.000000000000000000, -0.000000000000000000, -0.000000000000000000 ) ) ;
#90366=ADVANCED_FACE ( 'NONE', ( #17497, #83499 ), #94347, .T. ) ;
#90367=CARTESIAN_POINT ( 'NONE',  ( 24.18706980810188867, -2.126176841940956130, 7.934999999999991616 ) ) ;
#90402=CARTESIAN_POINT ( 'NONE',  ( 152.4000000000000057, -17.48000000000005016, 34.92499999999998295 ) ) ;
#90405=AXIS2_PLACEMENT_3D ( 'NONE', #103600, #126785, #51401 ) ;
#90413=SURFACE_STYLE_USAGE ( .BOTH. , #77435 ) ;
#90417=CARTESIAN_POINT ( 'NONE',  ( 9.770833333333335702, 6.094999999999991758, 1.633150327867687102 ) ) ;
#90431=CARTESIAN_POINT ( 'NONE',  ( 122.6835989386367913, -43.15000000000001990, -34.92499999999998295 ) ) ;
#90432=VERTEX_POINT ( 'NONE', #54970 ) ;
#90457=COLOUR_RGB ( '', 0.66274510, 0.83137255, 0.94901961) ;
#90458=ORIENTED_EDGE ( 'NONE', *, *, #33006, .T. ) ;
#90472=CARTESIAN_POINT ( 'NONE',  ( 2.999999999999999112, -7.600000000000055600, -34.92499999999998295 ) ) ;
#90477=ORIENTED_EDGE ( 'NONE', *, *, #142448, .T. ) ;
#90480=CYLINDRICAL_SURFACE ( 'NONE', #24670, 6.094999999999989093 ) ;
#90492=ORIENTED_EDGE ( 'NONE', *, *, #55455, .F. ) ;
#90529=EDGE_CURVE ( 'NONE', #68141, #66768, #62123, .T. ) ;
#90553=ADVANCED_FACE ( 'NONE', ( #116489 ), #29033, .T. ) ;
#90560=CARTESIAN_POINT ( 'NONE',  ( 32.29623647476855552, 7.934999999999990727, -1.457635852685135314E-15 ) ) ;
#90601=CARTESIAN_POINT ( 'NONE',  ( 21.12456980810188867, -6.871911579029512218, 3.967499999999996252 ) ) ;
#90603=CARTESIAN_POINT ( 'NONE',  ( 151.4000000000000057, -16.48000000000005016, 33.92499999999998295 ) ) ;
#90633=CARTESIAN_POINT ( 'NONE',  ( 25.39999999999999858, -14.29000000000013593, 12.69999999999954632 ) ) ;
#90655=( GEOMETRIC_REPRESENTATION_CONTEXT ( 3 ) GLOBAL_UNCERTAINTY_ASSIGNED_CONTEXT ( ( #11209 ) ) GLOBAL_UNIT_ASSIGNED_CONTEXT ( ( #69662, #113118, #113841 ) ) REPRESENTATION_CONTEXT ( 'NONE', 'WORKASPACE' ) );
#90669=COLOUR_RGB ( '', 0.40784314, 0.44705882, 0.49803922) ;
#90671=CARTESIAN_POINT ( 'NONE',  ( 2.254569808101886341, -6.871911579029512218, 3.967499999999996252 ) ) ;
#90689=AXIS2_PLACEMENT_3D ( 'NONE', #91466, #16741, #105175 ) ;
#90725=STYLED_ITEM ( 'NONE', ( #83855 ), #65678 ) ;
#90731=CARTESIAN_POINT ( 'NONE',  ( 166.8575281714868481, 26.96999999999994202, -31.92499999999998295 ) ) ;
#90739=CARTESIAN_POINT ( 'NONE',  ( 26.31706980810189123, -2.126176841940956130, 7.934999999999991616 ) ) ;
#90757=CIRCLE ( 'NONE', #132475, 1.000000000000000888 ) ;
#90759=CIRCLE ( 'NONE', #28236, 3.000000000000002665 ) ;
#90798=CARTESIAN_POINT ( 'NONE',  ( 131.5423521607622490, -49.05583548141700589, 39.86617647058822911 ) ) ;
#90807=CARTESIAN_POINT ( 'NONE',  ( 0.9430526776243700615, 5.848452262106093258, 4.137244182379782309 ) ) ;
#90858=ORIENTED_EDGE ( 'NONE', *, *, #15785, .T. ) ;
#90864=AXIS2_PLACEMENT_3D ( 'NONE', #73779, #117954, #52032 ) ;
#90899=ORIENTED_EDGE ( 'NONE', *, *, #107815, .T. ) ;
#90911=CARTESIAN_POINT ( 'NONE',  ( 1.233736474768552860, 5.808823158059036373, 5.808823158059032821 ) ) ;
#90938=CARTESIAN_POINT ( 'NONE',  ( 21.04580628287044064, 5.278424836066143655, -3.047499999999997655 ) ) ;
#90943=ADVANCED_FACE ( 'NONE', ( #93846 ), #4627, .F. ) ;
#90946=FACE_OUTER_BOUND ( 'NONE', #133744, .T. ) ;
#90978=UNCERTAINTY_MEASURE_WITH_UNIT (LENGTH_MEASURE( 1.000000000000000082E-05 ), #122113, 'distance_accuracy_value', 'NONE');
#90986=CARTESIAN_POINT ( 'NONE',  ( 180.4193221990229574, -52.14999999999999147, -40.92499999999998295 ) ) ;
#91017=SURFACE_SIDE_STYLE ('',( #42521 ) ) ;
#91068=CARTESIAN_POINT ( 'NONE',  ( 25.40000000000001634, 7.525090494501557536, -2.550389573741807858 ) ) ;
#91083=CARTESIAN_POINT ( 'NONE',  ( 8.358306282870437087, -1.633150327867689988, 6.094999999999989981 ) ) ;
#91089=SURFACE_SIDE_STYLE ('',( #104044 ) ) ;
#91111=AXIS2_PLACEMENT_3D ( 'NONE', #96134, #62117, #43928 ) ;
#91114=CARTESIAN_POINT ( 'NONE',  ( 24.33290314143522437, -3.967499999999994476, 6.871911579029513106 ) ) ;
#91123=CARTESIAN_POINT ( 'NONE',  ( 28.00000000000002487, -52.14999999999999147, -34.92499999999976978 ) ) ;
#91125=UNCERTAINTY_MEASURE_WITH_UNIT (LENGTH_MEASURE( 1.000000000000000082E-05 ), #138315, 'distance_accuracy_value', 'NONE');
#91162=CARTESIAN_POINT ( 'NONE',  ( 16.18750000000000000, 4.461849672132297329, -4.461849672132302658 ) ) ;
#91172=COLOUR_RGB ( '', 0.08235294, 0.09019608, 0.10196078) ;
#91225=SURFACE_STYLE_FILL_AREA ( #58629 ) ;
#91232=VERTEX_POINT ( 'NONE', #128977 ) ;
#91258=CARTESIAN_POINT ( 'NONE',  ( 56.00000000000004974, -49.14999999999999147, -40.92499999999998295 ) ) ;
#91259=LINE ( 'NONE', #100689, #118992 ) ;
#91271=STYLED_ITEM ( 'NONE', ( #81861 ), #87823 ) ;
#91284=VERTEX_POINT ( 'NONE', #137739 ) ;
#91291=CARTESIAN_POINT ( 'NONE',  ( 29.37956980810188412, 3.967499999999998916, 6.871911579029510442 ) ) ;
#91313=CARTESIAN_POINT ( 'NONE',  ( 58.17012237851979961, -48.09441802426614032, -35.89947574910193850 ) ) ;
#91320=FILL_AREA_STYLE ('',( #692 ) ) ;
#91330=CARTESIAN_POINT ( 'NONE',  ( 24.62456980810188867, -6.871911579029512218, 3.967499999999996252 ) ) ;
#91338=ORIENTED_EDGE ( 'NONE', *, *, #60565, .F. ) ;
#91353=EDGE_CURVE ( 'NONE', #56501, #8328, #55722, .T. ) ;
#91385=CARTESIAN_POINT ( 'NONE',  ( 1.379569808101885897, 3.967499999999998916, 6.871911579029510442 ) ) ;
#91405=CARTESIAN_POINT ( 'NONE',  ( 184.1500000000000057, -30.18000000000009564, 15.92499999999935945 ) ) ;
#91436=ORIENTED_EDGE ( 'NONE', *, *, #132256, .T. ) ;
#91443=CARTESIAN_POINT ( 'NONE',  ( 30.69206980810189123, -7.934999999999991616, -2.126176841940955242 ) ) ;
#91444=CARTESIAN_POINT ( 'NONE',  ( -1.245430191898114103, -6.871911579029512218, 3.967499999999996252 ) ) ;
#91451=SURFACE_SIDE_STYLE ('',( #47278 ) ) ;
#91461=EDGE_CURVE ( 'NONE', #47238, #132969, #143421, .T. ) ;
#91466=CARTESIAN_POINT ( 'NONE',  ( 174.7500000000000000, 7.919999999999947526, 19.12499999999998224 ) ) ;
#91477=SURFACE_STYLE_FILL_AREA ( #98249 ) ;
#91485=SURFACE_STYLE_FILL_AREA ( #26223 ) ;
#91487=CARTESIAN_POINT ( 'NONE',  ( 2.999999999999999112, -1.600000000000012301, -20.40202195861969514 ) ) ;
#91493=ORIENTED_EDGE ( 'NONE', *, *, #46934, .T. ) ;
#91500=CARTESIAN_POINT ( 'NONE',  ( 0.8141326222277666114, -6.652716765028095836, -2.974119808974657886 ) ) ;
#91512=CARTESIAN_POINT ( 'NONE',  ( 0.4200025801390303015, 6.514529779848684754, -4.079159782690128466 ) ) ;
#91558=ADVANCED_FACE ( 'NONE', ( #2739 ), #90480, .F. ) ;
#91567=CARTESIAN_POINT ( 'NONE',  ( 152.4000000000000057, 0.000000000000000000, 0.000000000000000000 ) ) ;
#91583=CARTESIAN_POINT ( 'NONE',  ( 0.000000000000000000, -43.14999999999999147, 31.92499999999998295 ) ) ;
#91599=DIRECTION ( 'NONE',  ( 0.000000000000000000, 0.000000000000000000, -1.000000000000000000 ) ) ;
#91602=CARTESIAN_POINT ( 'NONE',  ( 1.817069808101886341, -2.126176841940956130, 7.934999999999991616 ) ) ;
#91626=DIRECTION ( 'NONE',  ( 0.9707728879609285322, 0.000000000000000000, 0.2399999999999971323 ) ) ;
#91627=CARTESIAN_POINT ( 'NONE',  ( 21.48330628287043709, 6.094999999999991758, 1.633150327867686880 ) ) ;
#91634=FACE_OUTER_BOUND ( 'NONE', #21476, .T. ) ;
#91637=CARTESIAN_POINT ( 'NONE',  ( 6.541236474768553855, 0.000000000000000000, 7.934999999999990727 ) ) ;
#91700=EDGE_CURVE ( 'NONE', #47857, #90251, #95930, .T. ) ;
#91727=PRESENTATION_STYLE_ASSIGNMENT (( #99748 ) ) ;
#91760=CARTESIAN_POINT ( 'NONE',  ( 1.941639616203772123, -6.094999999999989093, 1.633150327867691765 ) ) ;
#91781=PLANE ( 'NONE',  #102455 ) ;
#91789=CARTESIAN_POINT ( 'NONE',  ( 27.10373647476855652, 5.808823158059036373, 5.808823158059032821 ) ) ;
#91800=AXIS2_PLACEMENT_3D ( 'NONE', #53741, #118234, #88507 ) ;
#91811=AXIS2_PLACEMENT_3D ( 'NONE', #14804, #106063, #61907 ) ;
#91824=( NAMED_UNIT ( * ) PLANE_ANGLE_UNIT ( ) SI_UNIT ( $, .RADIAN. ) );
#91837=CARTESIAN_POINT ( 'NONE',  ( 23.47916666666666785, 6.094999999999988205, -1.633150327867694651 ) ) ;
#91839=( LENGTH_UNIT ( ) NAMED_UNIT ( * ) SI_UNIT ( .MILLI., .METRE. ) );
#91848=LINE ( 'NONE', #135395, #9873 ) ;
#91886=CARTESIAN_POINT ( 'NONE',  ( 156.1500000000000057, -57.14999999999999147, -49.92499999999968452 ) ) ;
#91940=EDGE_CURVE ( 'NONE', #97576, #23170, #133811, .T. ) ;
#91954=COLOUR_RGB ( '', 0.09019608, 0.27058824, 0.51372549) ;
#91966=CARTESIAN_POINT ( 'NONE',  ( 28.21290314143522338, 3.967499999999992699, -6.871911579029513994 ) ) ;
#91988=PRESENTATION_STYLE_ASSIGNMENT (( #34777 ) ) ;
#92004=CARTESIAN_POINT ( 'NONE',  ( 25.39999999999999858, 7.464222240803104598E-16, -6.094999999999989093 ) ) ;
#92008=CARTESIAN_POINT ( 'NONE',  ( 30.74956980810188867, 3.967499999999998916, 6.871911579029510442 ) ) ;
#92009=CARTESIAN_POINT ( 'NONE',  ( 0.2890851266676670583, -7.934999999999988951, 1.853802869168066358 ) ) ;
#92020=DIRECTION ( 'NONE',  ( 0.000000000000000000, -2.921639538487157626E-15, 1.000000000000000000 ) ) ;
#92034=SURFACE_STYLE_FILL_AREA ( #126795 ) ;
#92059=( LENGTH_UNIT ( ) NAMED_UNIT ( * ) SI_UNIT ( .MILLI., .METRE. ) );
#92061=TOROIDAL_SURFACE ( 'NONE', #68926, 9.000000000000001776, 3.000000000000000000 ) ;
#92082=SURFACE_STYLE_FILL_AREA ( #103656 ) ;
#92104=CARTESIAN_POINT ( 'NONE',  ( 156.1499999999997783, -49.14999999999999147, -34.92499999999975557 ) ) ;
#92123=CARTESIAN_POINT ( 'NONE',  ( 4.879569808101885897, 3.967499999999998916, 6.871911579029510442 ) ) ;
#92129=SURFACE_STYLE_USAGE ( .BOTH. , #91451 ) ;
#92177=DIRECTION ( 'NONE',  ( 0.000000000000000000, -1.000000000000000000, 0.000000000000000000 ) ) ;
#92191=CARTESIAN_POINT ( 'NONE',  ( 1.179137009529055646, 2.860328551334985203, 6.310333628962586872 ) ) ;
#92197=( NAMED_UNIT ( * ) PLANE_ANGLE_UNIT ( ) SI_UNIT ( $, .RADIAN. ) );
#92205=( NAMED_UNIT ( * ) PLANE_ANGLE_UNIT ( ) SI_UNIT ( $, .RADIAN. ) );
#92210=( GEOMETRIC_REPRESENTATION_CONTEXT ( 3 ) GLOBAL_UNCERTAINTY_ASSIGNED_CONTEXT ( ( #126078 ) ) GLOBAL_UNIT_ASSIGNED_CONTEXT ( ( #1733, #13347, #82230 ) ) REPRESENTATION_CONTEXT ( 'NONE', 'WORKASPACE' ) );
#92227=DIRECTION ( 'NONE',  ( -1.000000000000000000, -0.000000000000000000, -0.000000000000000000 ) ) ;
#92248=AXIS2_PLACEMENT_3D ( 'NONE', #109559, #76974, #122561 ) ;
#92275=CARTESIAN_POINT ( 'NONE',  ( 16.04166666666666785, 3.047499999999993214, -5.278424836066146320 ) ) ;
#92283=CIRCLE ( 'NONE', #18170, 1.000000000000000888 ) ;
#92292=CARTESIAN_POINT ( 'NONE',  ( 26.40000000000000568, -16.48000000000005016, -12.70000000000043272 ) ) ;
#92293=CARTESIAN_POINT ( 'NONE',  ( 8.817069808101885897, -2.126176841940956130, 7.934999999999991616 ) ) ;
#92298=CARTESIAN_POINT ( 'NONE',  ( 25.38743044895410961, -6.094999999999989093, -0.1392054293825079614 ) ) ;
#92302=ORIENTED_EDGE ( 'NONE', *, *, #96098, .F. ) ;
#92308=EDGE_CURVE ( 'NONE', #9331, #122655, #45239, .T. ) ;
#92323=CARTESIAN_POINT ( 'NONE',  ( 3.624569808101886448, -6.871911579029512218, 3.967499999999996252 ) ) ;
#92345=STYLED_ITEM ( 'NONE', ( #22667 ), #63034 ) ;
#92352=CARTESIAN_POINT ( 'NONE',  ( 11.95833333333333393, -3.047499999999997211, -5.278424836066143655 ) ) ;
#92356=UNCERTAINTY_MEASURE_WITH_UNIT (LENGTH_MEASURE( 1.000000000000000082E-05 ), #54916, 'distance_accuracy_value', 'NONE');
#92376=FACE_OUTER_BOUND ( 'NONE', #83793, .T. ) ;
#92392=( NAMED_UNIT ( * ) PLANE_ANGLE_UNIT ( ) SI_UNIT ( $, .RADIAN. ) );
#92439=COLOUR_RGB ( '', 0.08235294, 0.09019608, 0.10196078) ;
#92456=CARTESIAN_POINT ( 'NONE',  ( 2.816639616203772789, -1.633150327867691987, -6.094999999999989093 ) ) ;
#92479=CARTESIAN_POINT ( 'NONE',  ( 184.1500000000000057, 26.96999999999993847, 34.92499999999998295 ) ) ;
#92493=CARTESIAN_POINT ( 'NONE',  ( 18.79123647476855652, -9.717572351234235426E-16, -7.934999999999990727 ) ) ;
#92535=CARTESIAN_POINT ( 'NONE',  ( 21.14583333333333570, -1.633150327867689988, 6.094999999999989981 ) ) ;
#92566=EDGE_CURVE ( 'NONE', #125982, #132969, #45728, .T. ) ;
#92585=CARTESIAN_POINT ( 'NONE',  ( 52.39921342269823867, -49.14999999999999147, -40.57473644908944266 ) ) ;
#92606=CARTESIAN_POINT ( 'NONE',  ( 9.916666666666667851, 5.278424836066147208, 3.047499999999990550 ) ) ;
#92623=ORIENTED_EDGE ( 'NONE', *, *, #5030, .T. ) ;
#92665=CARTESIAN_POINT ( 'NONE',  ( 27.77540314143521982, -2.126176841940958351, -7.934999999999989839 ) ) ;
#92670=EDGE_LOOP ( 'NONE', ( #87345, #85787, #85689, #131823 ) ) ;
#92689=CIRCLE ( 'NONE', #111210, 2.999999999999997335 ) ;
#92713=CARTESIAN_POINT ( 'NONE',  ( 32.79123647476855297, -9.717572351234235426E-16, -7.934999999999990727 ) ) ;
#92715=CARTESIAN_POINT ( 'NONE',  ( 8.145403141435220817, -2.126176841940958351, -7.934999999999988951 ) ) ;
#92736=FACE_OUTER_BOUND ( 'NONE', #65004, .T. ) ;
#92748=EDGE_CURVE ( 'NONE', #58595, #138592, #24879, .T. ) ;
#92768=AXIS2_PLACEMENT_3D ( 'NONE', #1857, #47603, #35290 ) ;
#92775=CARTESIAN_POINT ( 'NONE',  ( 0.3587364747685527488, 5.808823158059031044, -5.808823158059037262 ) ) ;
#92803=COLOUR_RGB ( '', 0.08235294, 0.09019608, 0.10196078) ;
#92804=CARTESIAN_POINT ( 'NONE',  ( 27.99999999999999645, -49.14999999999999147, -49.92499999999968452 ) ) ;
#92844=LINE ( 'NONE', #47957, #19538 ) ;
#92845=CARTESIAN_POINT ( 'NONE',  ( 0.3587364747685527488, 5.808823158059031044, -5.808823158059038150 ) ) ;
#92856=( NAMED_UNIT ( * ) SI_UNIT ( $, .STERADIAN. ) SOLID_ANGLE_UNIT ( ) );
#92899=AXIS2_PLACEMENT_3D ( 'NONE', #135100, #57527, #93702 ) ;
#92907=VERTEX_POINT ( 'NONE', #91405 ) ;
#92973=VECTOR ( 'NONE', #70105, 1000.000000000000000 ) ;
#92984=( GEOMETRIC_REPRESENTATION_CONTEXT ( 3 ) GLOBAL_UNCERTAINTY_ASSIGNED_CONTEXT ( ( #123048 ) ) GLOBAL_UNIT_ASSIGNED_CONTEXT ( ( #57990, #93435, #72441 ) ) REPRESENTATION_CONTEXT ( 'NONE', 'WORKASPACE' ) );
#92986=AXIS2_PLACEMENT_3D ( 'NONE', #106307, #118646, #38247 ) ;
#93007=AXIS2_PLACEMENT_3D ( 'NONE', #71079, #81244, #124722 ) ;
#93025=LINE ( 'NONE', #30644, #131986 ) ;
#93027=CARTESIAN_POINT ( 'NONE',  ( 7.650403141435218934, 7.934999999999989839, -2.126176841940961904 ) ) ;
#93032=EDGE_CURVE ( 'NONE', #36041, #106598, #651, .T. ) ;
#93053=CARTESIAN_POINT ( 'NONE',  ( 8.212472949537106715, 0.000000000000000000, 6.094999999999989981 ) ) ;
#93057=ADVANCED_FACE ( 'NONE', ( #58473 ), #45430, .F. ) ;
#93060=COLOUR_RGB ( '', 0.72549020, 0.75294118, 0.79215686) ;
#93065=CARTESIAN_POINT ( 'NONE',  ( 2.603736474768552522, 5.808823158059036373, 5.808823158059032821 ) ) ;
#93085=ORIENTED_EDGE ( 'NONE', *, *, #95752, .F. ) ;
#93131=DIRECTION ( 'NONE',  ( -1.000000000000000000, -0.000000000000000000, -0.000000000000000000 ) ) ;
#93146=COLOUR_RGB ( '', 0.31764706, 0.68627451, 0.89019608) ;
#93193=CARTESIAN_POINT ( 'NONE',  ( 14.77497294953710494, 4.461849672132300881, 4.461849672132299105 ) ) ;
#93214=CIRCLE ( 'NONE', #51535, 3.000000000000002665 ) ;
#93215=STYLED_ITEM ( 'NONE', ( #83890 ), #62638 ) ;
#93226=CARTESIAN_POINT ( 'NONE',  ( 20.54123647476855652, 0.000000000000000000, 7.934999999999990727 ) ) ;
#93240=SURFACE_STYLE_FILL_AREA ( #134629 ) ;
#93259=CARTESIAN_POINT ( 'NONE',  ( 180.4193221990230143, -49.14999999999999147, 40.92499999999998295 ) ) ;
#93267=FILL_AREA_STYLE ('',( #106253 ) ) ;
#93271=CARTESIAN_POINT ( 'NONE',  ( 26.97916666666666785, 6.094999999999988205, -1.633150327867694651 ) ) ;
#93273=DIRECTION ( 'NONE',  ( 0.000000000000000000, 0.000000000000000000, 1.000000000000000000 ) ) ;
#93280=EDGE_CURVE ( 'NONE', #117911, #92907, #19882, .T. ) ;
#93288=CARTESIAN_POINT ( 'NONE',  ( 24.39999999999999858, 1.399999999999986366, 20.40202195861970580 ) ) ;
#93298=CARTESIAN_POINT ( 'NONE',  ( 12.83333333333333393, 5.278424836066143655, -3.047499999999997655 ) ) ;
#93300=CARTESIAN_POINT ( 'NONE',  ( 1.971958729986437842, -5.986773400458673677, 1.339903956443486477 ) ) ;
#93309=( LENGTH_UNIT ( ) NAMED_UNIT ( * ) SI_UNIT ( .MILLI., .METRE. ) );
#93331=SURFACE_SIDE_STYLE ('',( #115044 ) ) ;
#93348=SURFACE_SIDE_STYLE ('',( #17213 ) ) ;
#93378=PLANE ( 'NONE',  #132442 ) ;
#93385=DIRECTION ( 'NONE',  ( 0.000000000000000000, -5.559056632600921604E-15, 1.000000000000000000 ) ) ;
#93393=SURFACE_STYLE_FILL_AREA ( #49204 ) ;
#93399=CARTESIAN_POINT ( 'NONE',  ( 25.00456980810188767, 6.871911579029510442, -3.967499999999998916 ) ) ;
#93427=CARTESIAN_POINT ( 'NONE',  ( 56.45153347184069759, -50.67230138428258357, -37.61253110040615866 ) ) ;
#93434=VERTEX_POINT ( 'NONE', #91583 ) ;
#93435=( NAMED_UNIT ( * ) PLANE_ANGLE_UNIT ( ) SI_UNIT ( $, .RADIAN. ) );
#93448=CARTESIAN_POINT ( 'NONE',  ( 32.93706980810188156, 2.126176841940952134, -7.934999999999993392 ) ) ;
#93449=CARTESIAN_POINT ( 'NONE',  ( 3.478736474768552078, -5.808823158059033709, 5.808823158059035485 ) ) ;
#93451=CARTESIAN_POINT ( 'NONE',  ( 25.39999999999999858, -1.600000000000055600, -28.92500000000001492 ) ) ;
#93460=FILL_AREA_STYLE ('',( #4228 ) ) ;
#93504=CARTESIAN_POINT ( 'NONE',  ( 9.546236474768553748, -7.934999999999990727, 4.858786175617117713E-16 ) ) ;
#93506=CARTESIAN_POINT ( 'NONE',  ( 21.58333333333333570, -5.278424836066144543, 3.047499999999995879 ) ) ;
#93519=ORIENTED_EDGE ( 'NONE', *, *, #8288, .T. ) ;
#93524=FACE_OUTER_BOUND ( 'NONE', #36075, .T. ) ;
#93535=ORIENTED_EDGE ( 'NONE', *, *, #52881, .F. ) ;
#93575=CARTESIAN_POINT ( 'NONE',  ( 4.004569808101885897, 6.871911579029510442, -3.967499999999998916 ) ) ;
#93580=CARTESIAN_POINT ( 'NONE',  ( 55.45435323442900710, -52.10358567239661198, -40.45860062937833845 ) ) ;
#93581=( LENGTH_UNIT ( ) NAMED_UNIT ( * ) SI_UNIT ( .MILLI., .METRE. ) );
#93593=CARTESIAN_POINT ( 'NONE',  ( 181.0498351327038336, -48.63026969829239476, -38.45492102172726590 ) ) ;
#93609=SURFACE_SIDE_STYLE ('',( #16000 ) ) ;
#93614=( NAMED_UNIT ( * ) PLANE_ANGLE_UNIT ( ) SI_UNIT ( $, .RADIAN. ) );
#93633=ORIENTED_EDGE ( 'NONE', *, *, #30482, .F. ) ;
#93636=SURFACE_SIDE_STYLE ('',( #26936 ) ) ;
#93651=FILL_AREA_STYLE_COLOUR ( '', #77594 ) ;
#93659=SURFACE_STYLE_USAGE ( .BOTH. , #16041 ) ;
#93702=DIRECTION ( 'NONE',  ( 0.000000000000000000, 0.000000000000000000, 1.000000000000000000 ) ) ;
#93743=CARTESIAN_POINT ( 'NONE',  ( 5.754569808101886785, -6.871911579029512218, 3.967499999999996252 ) ) ;
#93758=DIRECTION ( 'NONE',  ( 0.000000000000000000, 0.000000000000000000, -1.000000000000000000 ) ) ;
#93772=SURFACE_SIDE_STYLE ('',( #49588 ) ) ;
#93777=FACE_OUTER_BOUND ( 'NONE', #57370, .T. ) ;
#93778=CARTESIAN_POINT ( 'NONE',  ( 4.645403141435220817, -2.126176841940958351, -7.934999999999989839 ) ) ;
#93784=VERTEX_POINT ( 'NONE', #132809 ) ;
#93800=CARTESIAN_POINT ( 'NONE',  ( 11.22916666666666430, -6.094999999999989093, 1.633150327867691542 ) ) ;
#93804=UNCERTAINTY_MEASURE_WITH_UNIT (LENGTH_MEASURE( 1.000000000000000082E-05 ), #39029, 'distance_accuracy_value', 'NONE');
#93846=FACE_OUTER_BOUND ( 'NONE', #109445, .T. ) ;
#93863=DIRECTION ( 'NONE',  ( -0.000000000000000000, 1.000000000000000000, 0.000000000000000000 ) ) ;
#93870=PRODUCT_CONTEXT ( 'NONE', #53097, 'mechanical' ) ;
#93900=CARTESIAN_POINT ( 'NONE',  ( 19.73330628287043709, -6.094999999999989981, -1.633150327867689100 ) ) ;
#93928=VERTEX_POINT ( 'NONE', #26856 ) ;
#93935=COLOUR_RGB ( '', 0.31764706, 0.68627451, 0.89019608) ;
#93945=UNCERTAINTY_MEASURE_WITH_UNIT (LENGTH_MEASURE( 1.000000000000000082E-05 ), #44005, 'distance_accuracy_value', 'NONE');
#93950=CARTESIAN_POINT ( 'NONE',  ( 0.8183591370940836995, -52.14999999999999147, -41.64500000000001023 ) ) ;
#93958=ORIENTED_EDGE ( 'NONE', *, *, #98585, .F. ) ;
#93974=PRESENTATION_STYLE_ASSIGNMENT (( #28748 ) ) ;
#93979=CARTESIAN_POINT ( 'NONE',  ( 20.56250000000000000, 4.461849672132300881, 4.461849672132299105 ) ) ;
#93981=CARTESIAN_POINT ( 'NONE',  ( 24.39999999999999858, -7.600000000000055600, -34.92499999999998295 ) ) ;
#94006=SURFACE_SIDE_STYLE ('',( #49835 ) ) ;
#94018=DIRECTION ( 'NONE',  ( 0.000000000000000000, 0.000000000000000000, -1.000000000000000000 ) ) ;
#94045=SURFACE_SIDE_STYLE ('',( #28813 ) ) ;
#94047=DIRECTION ( 'NONE',  ( 0.000000000000000000, 0.000000000000000000, 1.000000000000000000 ) ) ;
#94092=LINE ( 'NONE', #129575, #111349 ) ;
#94095=CARTESIAN_POINT ( 'NONE',  ( 5.520403141435219929, 7.934999999999989839, -2.126176841940961904 ) ) ;
#94100=ORIENTED_EDGE ( 'NONE', *, *, #127825, .T. ) ;
#94119=CARTESIAN_POINT ( 'NONE',  ( 55.57593013779389679, -49.04047092357291149, -39.41690992498757140 ) ) ;
#94125=UNCERTAINTY_MEASURE_WITH_UNIT (LENGTH_MEASURE( 1.000000000000000082E-05 ), #78129, 'distance_accuracy_value', 'NONE');
#94139=CARTESIAN_POINT ( 'NONE',  ( 28.12456980810188867, -6.871911579029512218, 3.967499999999996252 ) ) ;
#94140=CARTESIAN_POINT ( 'NONE',  ( 5.374569808101886892, 6.871911579029510442, -3.967499999999998916 ) ) ;
#94169=CARTESIAN_POINT ( 'NONE',  ( 55.47768537940099520, -49.13871568195843764, 40.16438383193126072 ) ) ;
#94178=CARTESIAN_POINT ( 'NONE',  ( 8.166666666666667851, -5.278424836066145431, -3.047499999999993658 ) ) ;
#94199=CARTESIAN_POINT ( 'NONE',  ( 6.337903141435219823, -6.871911579029513106, -3.967499999999993587 ) ) ;
#94219=CARTESIAN_POINT ( 'NONE',  ( 6.125000000000000000, 6.094999999999989981, -1.119633336120465690E-15 ) ) ;
#94220=DIRECTION ( 'NONE',  ( 1.000000000000000000, -0.000000000000000000, -0.000000000000000000 ) ) ;
#94221=DIRECTION ( 'NONE',  ( -1.000000000000000000, 0.000000000000000000, 0.000000000000000000 ) ) ;
#94239=VECTOR ( 'NONE', #110775, 1000.000000000000000 ) ;
#94244=( LENGTH_UNIT ( ) NAMED_UNIT ( * ) SI_UNIT ( .MILLI., .METRE. ) );
#94248=( GEOMETRIC_REPRESENTATION_CONTEXT ( 3 ) GLOBAL_UNCERTAINTY_ASSIGNED_CONTEXT ( ( #59226 ) ) GLOBAL_UNIT_ASSIGNED_CONTEXT ( ( #90075, #56798, #75657 ) ) REPRESENTATION_CONTEXT ( 'NONE', 'WORKASPACE' ) );
#94274=CARTESIAN_POINT ( 'NONE',  ( 0.7962364747685526378, 7.934999999999990727, -1.457635852685135314E-15 ) ) ;
#94285=SURFACE_STYLE_FILL_AREA ( #49401 ) ;
#94307=UNCERTAINTY_MEASURE_WITH_UNIT (LENGTH_MEASURE( 1.000000000000000082E-05 ), #16617, 'distance_accuracy_value', 'NONE');
#94312=COLOUR_RGB ( '', 0.08235294, 0.09019608, 0.10196078) ;
#94333=DIRECTION ( 'NONE',  ( 1.000000000000000000, -0.000000000000000000, -0.000000000000000000 ) ) ;
#94337=FACE_OUTER_BOUND ( 'NONE', #14700, .T. ) ;
#94338=COLOUR_RGB ( '', 0.40784314, 0.44705882, 0.49803922) ;
#94347=PLANE ( 'NONE',  #33621 ) ;
#94442=CARTESIAN_POINT ( 'NONE',  ( 12.75456980810188767, -6.871911579029512218, 3.967499999999996252 ) ) ;
#94448=CARTESIAN_POINT ( 'NONE',  ( 24.64583333333333925, -1.633150327867709528, 6.094999999999979323 ) ) ;
#94473=CARTESIAN_POINT ( 'NONE',  ( 174.7500000000000000, 7.919999999999947526, -18.97500000000001918 ) ) ;
#94474=CARTESIAN_POINT ( 'NONE',  ( 0.9995698081018862258, -3.967499999999998028, -6.871911579029511330 ) ) ;
#94498=CARTESIAN_POINT ( 'NONE',  ( 12.25000000000000000, -7.464222240803106570E-16, -6.094999999999989981 ) ) ;
#94536=VECTOR ( 'NONE', #86958, 1000.000000000000000 ) ;
#94546=FACE_OUTER_BOUND ( 'NONE', #36517, .T. ) ;
#94553=EDGE_CURVE ( 'NONE', #90432, #52479, #112844, .T. ) ;
#94567=CARTESIAN_POINT ( 'NONE',  ( 184.1500000000000057, -14.29000000000013593, 12.69999999999954632 ) ) ;
#94570=( LENGTH_UNIT ( ) NAMED_UNIT ( * ) SI_UNIT ( .MILLI., .METRE. ) );
#94576=ORIENTED_EDGE ( 'NONE', *, *, #125526, .F. ) ;
#94580=AXIS2_PLACEMENT_3D ( 'NONE', #130877, #31544, #10475 ) ;
#94605=CARTESIAN_POINT ( 'NONE',  ( 19.58747294953710849, -6.094999999999989981, 3.732111120401553285E-16 ) ) ;
#94621=ORIENTED_EDGE ( 'NONE', *, *, #20545, .T. ) ;
#94637=CARTESIAN_POINT ( 'NONE',  ( 34.10373647476854586, 5.808823158059036373, 5.808823158059032821 ) ) ;
#94660=VECTOR ( 'NONE', #69372, 1000.000000000000000 ) ;
#94663=EDGE_LOOP ( 'NONE', ( #42475, #39459, #50836, #36328, #112415, #71968, #3707, #33132, #10071, #3633, #31335, #118713, #143, #132477, #86641 ) ) ;
#94667=ORIENTED_EDGE ( 'NONE', *, *, #66597, .F. ) ;
#94670=FILL_AREA_STYLE ('',( #7666 ) ) ;
#94680=CARTESIAN_POINT ( 'NONE',  ( 19.10416666666666430, -1.633150327867691987, -6.094999999999989093 ) ) ;
#94681=AXIS2_PLACEMENT_3D ( 'NONE', #44147, #76053, #143435 ) ;
#94693=DIRECTION ( 'NONE',  ( -1.000000000000000000, -0.000000000000000000, -0.000000000000000000 ) ) ;
#94700=( NAMED_UNIT ( * ) SI_UNIT ( $, .STERADIAN. ) SOLID_ANGLE_UNIT ( ) );
#94701=SURFACE_SIDE_STYLE ('',( #74424 ) ) ;
#94719=( GEOMETRIC_REPRESENTATION_CONTEXT ( 3 ) GLOBAL_UNCERTAINTY_ASSIGNED_CONTEXT ( ( #140341 ) ) GLOBAL_UNIT_ASSIGNED_CONTEXT ( ( #94244, #39905, #127605 ) ) REPRESENTATION_CONTEXT ( 'NONE', 'WORKASPACE' ) );
#94730=CARTESIAN_POINT ( 'NONE',  ( 25.39999999999999858, -5.938110122598772023, -4.485947909153642499 ) ) ;
#94743=DIRECTION ( 'NONE',  ( 0.000000000000000000, 0.000000000000000000, 1.000000000000000000 ) ) ;
#94760=ORIENTED_EDGE ( 'NONE', *, *, #142429, .F. ) ;
#94792=CARTESIAN_POINT ( 'NONE',  ( 0.3818979091348736477, -51.95642703808907470, 39.54367611436850893 ) ) ;
#94794=CARTESIAN_POINT ( 'NONE',  ( 3.187069808101886448, -2.126176841940956130, 7.934999999999991616 ) ) ;
#94816=ORIENTED_EDGE ( 'NONE', *, *, #43473, .T. ) ;
#94840=CARTESIAN_POINT ( 'NONE',  ( 27.54123647476855652, 0.000000000000000000, 7.934999999999990727 ) ) ;
#94841=CARTESIAN_POINT ( 'NONE',  ( 12.22873647476855119, 5.808823158059031044, -5.808823158059037262 ) ) ;
#94854=VERTEX_POINT ( 'NONE', #11929 ) ;
#94855=PLANE ( 'NONE',  #98944 ) ;
#94875=CARTESIAN_POINT ( 'NONE',  ( 59.37656097284888546, -44.54322672567602837, 35.04755940937982217 ) ) ;
#94881=FACE_OUTER_BOUND ( 'NONE', #37824, .T. ) ;
#94899=VERTEX_POINT ( 'NONE', #113929 ) ;
#94904=CARTESIAN_POINT ( 'NONE',  ( 6.483736474768551972, -5.808823158059035485, -5.808823158059033709 ) ) ;
#94972=CARTESIAN_POINT ( 'NONE',  ( 11.73373647476855197, 5.808823158059036373, 5.808823158059032821 ) ) ;
#94985=CARTESIAN_POINT ( 'NONE',  ( 180.8518557880187245, -48.98056306480257405, -39.49745726092499609 ) ) ;
#95014=DIRECTION ( 'NONE',  ( 1.000000000000000000, 0.000000000000000000, 0.000000000000000000 ) ) ;
#95025=( GEOMETRIC_REPRESENTATION_CONTEXT ( 3 ) GLOBAL_UNCERTAINTY_ASSIGNED_CONTEXT ( ( #70800 ) ) GLOBAL_UNIT_ASSIGNED_CONTEXT ( ( #102105, #56497, #100674 ) ) REPRESENTATION_CONTEXT ( 'NONE', 'WORKASPACE' ) );
#95030=VERTEX_POINT ( 'NONE', #85568 ) ;
#95031=ORIENTED_EDGE ( 'NONE', *, *, #120959, .F. ) ;
#95037=CIRCLE ( 'NONE', #74269, 1.000000000000000888 ) ;
#95042=SURFACE_STYLE_USAGE ( .BOTH. , #28388 ) ;
#95090=DIRECTION ( 'NONE',  ( 0.000000000000000000, -1.000000000000000000, 0.000000000000000000 ) ) ;
#95107=STYLED_ITEM ( 'NONE', ( #73100 ), #27925 ) ;
#95115=( LENGTH_UNIT ( ) NAMED_UNIT ( * ) SI_UNIT ( .MILLI., .METRE. ) );
#95136=CARTESIAN_POINT ( 'NONE',  ( 17.06250000000000000, 4.461849672132300881, 4.461849672132299105 ) ) ;
#95144=CARTESIAN_POINT ( 'NONE',  ( 20.17080628287043709, -3.047499999999997211, -5.278424836066143655 ) ) ;
#95156=CARTESIAN_POINT ( 'NONE',  ( 13.33790314143522160, -6.871911579029513106, -3.967499999999993587 ) ) ;
#95171=AXIS2_PLACEMENT_3D ( 'NONE', #41443, #19692, #129891 ) ;
#95189=CARTESIAN_POINT ( 'NONE',  ( 11.06206980810188689, -7.934999999999991616, -2.126176841940955242 ) ) ;
#95222=CARTESIAN_POINT ( 'NONE',  ( 24.39999999999999858, -1.599999999999997202, -17.44999999999996732 ) ) ;
#95236=SURFACE_STYLE_FILL_AREA ( #134677 ) ;
#95252=CIRCLE ( 'NONE', #32783, 5.000000000000000888 ) ;
#95275=EDGE_LOOP ( 'NONE', ( #66491, #127069, #92302, #67426, #70167 ) ) ;
#95314=DIRECTION ( 'NONE',  ( -1.000000000000000000, -0.000000000000000000, 0.000000000000000000 ) ) ;
#95325=EDGE_CURVE ( 'NONE', #95030, #100698, #79033, .T. ) ;
#95330=CARTESIAN_POINT ( 'NONE',  ( 18.85830628287044419, -1.633150327867689988, 6.094999999999989981 ) ) ;
#95336=CIRCLE ( 'NONE', #139372, 1.000000000000000888 ) ;
#95361=CARTESIAN_POINT ( 'NONE',  ( 28.85373647476855652, -5.808823158059035485, -5.808823158059033709 ) ) ;
#95405=CARTESIAN_POINT ( 'NONE',  ( 2.000000000000011546, 2.638703287232806449, -5.494203305479936184 ) ) ;
#95410=CARTESIAN_POINT ( 'NONE',  ( 31.20833333333333570, 3.047499999999997655, 5.278424836066143655 ) ) ;
#95433=CARTESIAN_POINT ( 'NONE',  ( 1.495847097294773720, -1.845811315201534741, 6.347071198332229436 ) ) ;
#95434=( LENGTH_UNIT ( ) NAMED_UNIT ( * ) SI_UNIT ( .MILLI., .METRE. ) );
#95447=VECTOR ( 'NONE', #20626, 1000.000000000000000 ) ;
#95465=ORIENTED_EDGE ( 'NONE', *, *, #131364, .F. ) ;
#95470=CARTESIAN_POINT ( 'NONE',  ( 184.1383206845090967, -50.55966373067078479, 35.89041033429542438 ) ) ;
#95488=CARTESIAN_POINT ( 'NONE',  ( 13.02497294953710849, -4.461849672132299993, -4.461849672132299105 ) ) ;
#95520=FILL_AREA_STYLE ('',( #138331 ) ) ;
#95523=CARTESIAN_POINT ( 'NONE',  ( -0.3129301918981140518, -2.126176841940956130, 7.934999999999991616 ) ) ;
#95567=EDGE_CURVE ( 'NONE', #117948, #62641, #57549, .T. ) ;
#95569=VECTOR ( 'NONE', #132328, 1000.000000000000000 ) ;
#95575=CARTESIAN_POINT ( 'NONE',  ( 8.312500000000000000, -4.461849672132299993, -4.461849672132299105 ) ) ;
#95576=CARTESIAN_POINT ( 'NONE',  ( 11.64540314143521904, -2.126176841940958351, -7.934999999999988951 ) ) ;
#95604=CARTESIAN_POINT ( 'NONE',  ( 57.88343899890263344, -48.52444309369084863, 36.09967824800554581 ) ) ;
#95612=CARTESIAN_POINT ( 'NONE',  ( 128.1415536296147195, -48.60795469097357113, 38.18754904899810754 ) ) ;
#95630=CARTESIAN_POINT ( 'NONE',  ( 25.39999999999999858, 0.000000000000000000, 6.094999999999989093 ) ) ;
#95632=CARTESIAN_POINT ( 'NONE',  ( 5.754569808101886785, -6.871911579029512218, 3.967499999999996252 ) ) ;
#95635=ORIENTED_EDGE ( 'NONE', *, *, #57603, .F. ) ;
#95688=ADVANCED_FACE ( 'NONE', ( #22265 ), #131787, .T. ) ;
#95704=CARTESIAN_POINT ( 'NONE',  ( 13.77540314143521982, -2.126176841940958351, -7.934999999999989839 ) ) ;
#95715=DIRECTION ( 'NONE',  ( -0.000000000000000000, 0.000000000000000000, 1.000000000000000000 ) ) ;
#95719=CARTESIAN_POINT ( 'NONE',  ( 184.0776099992117167, -48.13855614192994636, -37.56434003616361395 ) ) ;
#95752=EDGE_CURVE ( 'NONE', #31597, #75508, #68686, .T. ) ;
#95814=VECTOR ( 'NONE', #110818, 1000.000000000000227 ) ;
#95820=AXIS2_PLACEMENT_3D ( 'NONE', #116445, #114291, #14965 ) ;
#95852=MECHANICAL_DESIGN_GEOMETRIC_PRESENTATION_REPRESENTATION('',(#72841),#58879);
#95871=ADVANCED_FACE ( 'NONE', ( #59949 ), #38894, .F. ) ;
#95874=CARTESIAN_POINT ( 'NONE',  ( 14.50456980810188767, 6.871911579029510442, -3.967499999999998916 ) ) ;
#95911=CARTESIAN_POINT ( 'NONE',  ( 16.16623647476855652, 7.934999999999990727, -1.457635852685135314E-15 ) ) ;
#95913=STYLED_ITEM ( 'NONE', ( #90173 ), #44362 ) ;
#95926=CARTESIAN_POINT ( 'NONE',  ( 61.46640106136307935, -1.600000000000094458, 34.92499999999998295 ) ) ;
#95930=B_SPLINE_CURVE_WITH_KNOTS ( 'NONE', 3,
 ( #128802, #48392, #54147, #54839, #33116, #42548, #129505, #75178, #87461, #131678, #141854, #20751 ),
 .UNSPECIFIED., .F., .F.,
 ( 4, 2, 2, 2, 2, 4 ),
 ( 0.000000000000000000, 0.001108890051515397813, 0.001663335077273096719, 0.002217780103030795626, 0.003326670154546186500, 0.004435560206061577374 ),
 .UNSPECIFIED. ) ;
#95954=CIRCLE ( 'NONE', #133044, 34.93000000000001393 ) ;
#95982=DIRECTION ( 'NONE',  ( 0.000000000000000000, -1.000000000000000000, 0.000000000000000000 ) ) ;
#95991=ORIENTED_EDGE ( 'NONE', *, *, #111780, .F. ) ;
#96004=ORIENTED_EDGE ( 'NONE', *, *, #34298, .F. ) ;
#96008=COLOUR_RGB ( '', 0.72549020, 0.75294118, 0.79215686) ;
#96033=VERTEX_POINT ( 'NONE', #130925 ) ;
#96038=CARTESIAN_POINT ( 'NONE',  ( 16.08747294953710849, -6.094999999999989981, 3.732111120401553285E-16 ) ) ;
#96055=DIRECTION ( 'NONE',  ( -1.504632769052527134E-30, -3.469446951953615372E-15, -1.000000000000000000 ) ) ;
#96066=CARTESIAN_POINT ( 'NONE',  ( 29.29123647476855652, -9.717572351234235426E-16, -7.934999999999990727 ) ) ;
#96072=STYLED_ITEM ( 'NONE', ( #131807 ), #90366 ) ;
#96080=CARTESIAN_POINT ( 'NONE',  ( 3.596992905804716756, -49.14999999999999147, -40.56450646617317801 ) ) ;
#96098=EDGE_CURVE ( 'NONE', #134905, #65308, #64563, .T. ) ;
#96099=CARTESIAN_POINT ( 'NONE',  ( 24.39999999999999858, -5.520864266206504263E-14, 0.000000000000000000 ) ) ;
#96132=CARTESIAN_POINT ( 'NONE',  ( 12.68750000000000000, 4.461849672132297329, -4.461849672132302658 ) ) ;
#96134=CARTESIAN_POINT ( 'NONE',  ( 25.39999999999999858, 0.000000000000000000, 0.000000000000000000 ) ) ;
#96156=CARTESIAN_POINT ( 'NONE',  ( 25.39999999999999147, -6.343664649937126754, -2.773223721129034480 ) ) ;
#96170=CARTESIAN_POINT ( 'NONE',  ( 180.6665599231111230, -49.11775834062249402, 40.20665288736022802 ) ) ;
#96191=EDGE_LOOP ( 'NONE', ( #29216, #80625, #132984 ) ) ;
#96212=EDGE_LOOP ( 'NONE', ( #88490, #64002, #104639, #54181 ) ) ;
#96217=CARTESIAN_POINT ( 'NONE',  ( 0.06788206741516134013, -51.13011358081639912, 36.94363806876511802 ) ) ;
#96219=CARTESIAN_POINT ( 'NONE',  ( 8.582903141435219041, 3.967499999999992699, -6.871911579029513994 ) ) ;
#96242=CARTESIAN_POINT ( 'NONE',  ( 57.10144406050384447, -49.69743550128772114, -36.79359617903136126 ) ) ;
#96259=CARTESIAN_POINT ( 'NONE',  ( 3.208333333333333481, 3.047499999999997655, 5.278424836066143655 ) ) ;
#96260=CARTESIAN_POINT ( 'NONE',  ( 13.54123647476855474, 0.000000000000000000, 7.934999999999990727 ) ) ;
#96287=CARTESIAN_POINT ( 'NONE',  ( 61.46640106136305093, -43.15000000000001990, 34.92499999999998295 ) ) ;
#96295=CARTESIAN_POINT ( 'NONE',  ( 123.7287633665994804, -43.84677628532046612, 34.92499999999998295 ) ) ;
#96313=CARTESIAN_POINT ( 'NONE',  ( 5.025403141435219823, 2.126176841940962348, 7.934999999999988951 ) ) ;
#96323=STYLED_ITEM ( 'NONE', ( #119995 ), #12766 ) ;
#96334=( NAMED_UNIT ( * ) PLANE_ANGLE_UNIT ( ) SI_UNIT ( $, .RADIAN. ) );
#96340=CARTESIAN_POINT ( 'NONE',  ( 25.39999999999999858, -3.814127886917791255, -7.006053345101936891 ) ) ;
#96355=COLOUR_RGB ( '', 0.66274510, 0.83137255, 0.94901961) ;
#96390=CARTESIAN_POINT ( 'NONE',  ( 10.27540314143522160, -2.126176841940958351, -7.934999999999989839 ) ) ;
#96438=VERTEX_POINT ( 'NONE', #8195 ) ;
#96447=VECTOR ( 'NONE', #94220, 1000.000000000000000 ) ;
#96479=EDGE_CURVE ( 'NONE', #61213, #45028, #117909, .T. ) ;
#96493=MECHANICAL_DESIGN_GEOMETRIC_PRESENTATION_REPRESENTATION('',(#40963),#128908);
#96555=CARTESIAN_POINT ( 'NONE',  ( 21.21290314143522338, 3.967499999999992699, -6.871911579029513994 ) ) ;
#96562=CARTESIAN_POINT ( 'NONE',  ( 25.39999999999999858, -30.18000000000009564, 15.92499999999935945 ) ) ;
#96567=DIRECTION ( 'NONE',  ( 0.000000000000000000, 0.000000000000000000, 1.000000000000000000 ) ) ;
#96585=CARTESIAN_POINT ( 'NONE',  ( 11.64540314143521904, -2.126176841940958351, -7.934999999999989839 ) ) ;
#96593=CARTESIAN_POINT ( 'NONE',  ( 5.441639616203772789, -6.094999999999989093, 1.633150327867691542 ) ) ;
#96599=FILL_AREA_STYLE ('',( #8174 ) ) ;
#96610=CARTESIAN_POINT ( 'NONE',  ( 128.9683591370937847, -49.14999999999998437, 41.64499999999998181 ) ) ;
#96614=CARTESIAN_POINT ( 'NONE',  ( 2.000000000000011546, 2.638703287232806449, -5.494203305479936184 ) ) ;
#96653=( NAMED_UNIT ( * ) SI_UNIT ( $, .STERADIAN. ) SOLID_ANGLE_UNIT ( ) );
#96698=VERTEX_POINT ( 'NONE', #104513 ) ;
#96712=CYLINDRICAL_SURFACE ( 'NONE', #123110, 5.999999999999998224 ) ;
#96714=ADVANCED_FACE ( 'NONE', ( #82098 ), #114665, .T. ) ;
#96722=CARTESIAN_POINT ( 'NONE',  ( 23.23330628287043709, -6.094999999999989981, -1.633150327867689100 ) ) ;
#96733=AXIS2_PLACEMENT_3D ( 'NONE', #128560, #62598, #27813 ) ;
#96753=CARTESIAN_POINT ( 'NONE',  ( 33.37456980810188156, 6.871911579029510442, -3.967499999999998916 ) ) ;
#96762=CARTESIAN_POINT ( 'NONE',  ( 0.3818979091347701749, -51.95642703809002683, -39.54367611436767760 ) ) ;
#96776=EDGE_CURVE ( 'NONE', #90432, #98765, #55567, .T. ) ;
#96783=CARTESIAN_POINT ( 'NONE',  ( 181.1500000000000057, -43.14999999999999147, -40.92499999999998295 ) ) ;
#96794=ADVANCED_FACE ( 'NONE', ( #29802 ), #32503, .F. ) ;
#96804=CARTESIAN_POINT ( 'NONE',  ( 33.83333333333333570, 5.278424836066143655, -3.047499999999997655 ) ) ;
#96842=COLOUR_RGB ( '', 0.09019608, 0.27058824, 0.51372549) ;
#96856=FACE_OUTER_BOUND ( 'NONE', #31239, .T. ) ;
#96864=SURFACE_SIDE_STYLE ('',( #9888 ) ) ;
#96891=VERTEX_POINT ( 'NONE', #34638 ) ;
#96921=CARTESIAN_POINT ( 'NONE',  ( 0.3339215173232504275, -51.89584459748879652, 39.24672819827910786 ) ) ;
#96925=CARTESIAN_POINT ( 'NONE',  ( 1.145403141435219263, -2.126176841940958351, -7.934999999999989839 ) ) ;
#96957=EDGE_CURVE ( 'NONE', #8723, #121754, #138229, .T. ) ;
#96965=CARTESIAN_POINT ( 'NONE',  ( 6.125000000000000000, 6.094999999999989981, -1.119633336120465690E-15 ) ) ;
#96966=CARTESIAN_POINT ( 'NONE',  ( 15.72873647476855297, 5.808823158059031044, -5.808823158059037262 ) ) ;
#96977=CARTESIAN_POINT ( 'NONE',  ( 128.5740698622078071, -49.04047092356724136, -39.41690992498752877 ) ) ;
#96994=CARTESIAN_POINT ( 'NONE',  ( 59.70964273383167153, -44.90675832753628782, 35.11767176072511631 ) ) ;
#97000=CARTESIAN_POINT ( 'NONE',  ( 127.5247579190790219, -47.99115898043997674, 37.22402166429051817 ) ) ;
#97022=CARTESIAN_POINT ( 'NONE',  ( 16.10873647476855552, -5.808823158059033709, 5.808823158059035485 ) ) ;
#97044=CARTESIAN_POINT ( 'NONE',  ( 25.40000000000000924, 5.606709230119133025, -5.629648409862730851 ) ) ;
#97053=ORIENTED_EDGE ( 'NONE', *, *, #51233, .T. ) ;
#97057=( NAMED_UNIT ( * ) PLANE_ANGLE_UNIT ( ) SI_UNIT ( $, .RADIAN. ) );
#97069=AXIS2_PLACEMENT_3D ( 'NONE', #68924, #1462, #100812 ) ;
#97090=CARTESIAN_POINT ( 'NONE',  ( 13.62956980810188767, -3.967499999999998028, -6.871911579029511330 ) ) ;
#97095=CARTESIAN_POINT ( 'NONE',  ( 52.26932219902319332, -49.14999999999999147, -40.92499999999997584 ) ) ;
#97102=CARTESIAN_POINT ( 'NONE',  ( 174.7500000000000000, 7.919999999999947526, -18.97500000000001918 ) ) ;
#97108=COLOUR_RGB ( '', 0.08235294, 0.09019608, 0.10196078) ;
#97117=AXIS2_PLACEMENT_3D ( 'NONE', #42657, #97715, #9229 ) ;
#97228=CARTESIAN_POINT ( 'NONE',  ( 3.010806948443976339, -48.09618305010691586, 37.50858089739961798 ) ) ;
#97231=DIRECTION ( 'NONE',  ( 0.000000000000000000, 0.000000000000000000, -1.000000000000000000 ) ) ;
#97238=ORIENTED_EDGE ( 'NONE', *, *, #79028, .T. ) ;
#97239=( GEOMETRIC_REPRESENTATION_CONTEXT ( 3 ) GLOBAL_UNCERTAINTY_ASSIGNED_CONTEXT ( ( #89850 ) ) GLOBAL_UNIT_ASSIGNED_CONTEXT ( ( #3278, #70030, #48227 ) ) REPRESENTATION_CONTEXT ( 'NONE', 'WORKASPACE' ) );
#97266=CARTESIAN_POINT ( 'NONE',  ( 17.56706980810188767, 2.126176841940952134, -7.934999999999993392 ) ) ;
#97283=STYLED_ITEM ( 'NONE', ( #52846 ), #116793 ) ;
#97304=CARTESIAN_POINT ( 'NONE',  ( 15.72873647476855297, 5.808823158059031044, -5.808823158059038150 ) ) ;
#97305=DIRECTION ( 'NONE',  ( 0.000000000000000000, 0.000000000000000000, -1.000000000000000000 ) ) ;
#97311=CARTESIAN_POINT ( 'NONE',  ( 6.462472949537106715, -7.464222240803106570E-16, -6.094999999999989981 ) ) ;
#97357=DIRECTION ( 'NONE',  ( 0.000000000000000000, 2.312964634635743450E-15, 1.000000000000000000 ) ) ;
#97359=EDGE_CURVE ( 'NONE', #20435, #91284, #138059, .T. ) ;
#97399=VECTOR ( 'NONE', #10070, 1000.000000000000000 ) ;
#97401=VERTEX_POINT ( 'NONE', #139522 ) ;
#97406=VECTOR ( 'NONE', #100890, 1000.000000000000000 ) ;
#97459=EDGE_CURVE ( 'NONE', #132990, #116882, #70692, .T. ) ;
#97460=CARTESIAN_POINT ( 'NONE',  ( 29.21247294953710494, 0.000000000000000000, 6.094999999999989981 ) ) ;
#97475=EDGE_CURVE ( 'NONE', #87517, #94899, #114841, .T. ) ;
#97502=DIRECTION ( 'NONE',  ( 0.000000000000000000, 2.312964634635743450E-15, 1.000000000000000000 ) ) ;
#97549=CARTESIAN_POINT ( 'NONE',  ( 33.10416666666667140, -1.633150327867691987, -6.094999999999989093 ) ) ;
#97557=FILL_AREA_STYLE_COLOUR ( '', #43094 ) ;
#97571=FILL_AREA_STYLE_COLOUR ( '', #129403 ) ;
#97576=VERTEX_POINT ( 'NONE', #51776 ) ;
#97597=( NAMED_UNIT ( * ) PLANE_ANGLE_UNIT ( ) SI_UNIT ( $, .RADIAN. ) );
#97606=AXIS2_PLACEMENT_3D ( 'NONE', #26876, #63114, #6501 ) ;
#97608=VECTOR ( 'NONE', #8280, 1000.000000000000000 ) ;
#97639=ADVANCED_FACE ( 'NONE', ( #20529 ), #119835, .F. ) ;
#97670=CARTESIAN_POINT ( 'NONE',  ( 52.26932219902325727, -49.14999999999999147, 40.92499999999998295 ) ) ;
#97671=ORIENTED_EDGE ( 'NONE', *, *, #32380, .T. ) ;
#97674=CARTESIAN_POINT ( 'NONE',  ( 17.91623647476855652, -7.934999999999990727, 4.858786175617117713E-16 ) ) ;
#97684=SURFACE_STYLE_USAGE ( .BOTH. , #64352 ) ;
#97700=ORIENTED_EDGE ( 'NONE', *, *, #67089, .T. ) ;
#97705=EDGE_LOOP ( 'NONE', ( #77467, #85718, #99912, #10899 ) ) ;
#97709=STYLED_ITEM ( 'NONE', ( #81721 ), #77853 ) ;
#97715=DIRECTION ( 'NONE',  ( -0.000000000000000000, 1.000000000000000000, 0.000000000000000000 ) ) ;
#97720=CARTESIAN_POINT ( 'NONE',  ( 7.729166666666666075, -6.094999999999989093, 1.633150327867691765 ) ) ;
#97721=CARTESIAN_POINT ( 'NONE',  ( 14.12456980810188689, -6.871911579029512218, 3.967499999999996252 ) ) ;
#97725=SURFACE_STYLE_FILL_AREA ( #53518 ) ;
#97729=MECHANICAL_DESIGN_GEOMETRIC_PRESENTATION_REPRESENTATION('',(#56070),#35259);
#97739=STYLED_ITEM ( 'NONE', ( #40912 ), #18911 ) ;
#97740=CARTESIAN_POINT ( 'NONE',  ( 127.0485559394951025, -49.69743550128988829, -36.79359617903030966 ) ) ;
#97746=FACE_OUTER_BOUND ( 'NONE', #62805, .T. ) ;
#97753=CARTESIAN_POINT ( 'NONE',  ( 56.09195796767451014, -46.73296206246043738, 36.09967824800554581 ) ) ;
#97759=CARTESIAN_POINT ( 'NONE',  ( 131.3130295073144396, -48.90295371244932454, 39.18578444878558287 ) ) ;
#97763=LINE ( 'NONE', #20903, #32675 ) ;
#97779=CARTESIAN_POINT ( 'NONE',  ( 16.25456980810188767, -6.871911579029512218, 3.967499999999996252 ) ) ;
#97781=COLOUR_RGB ( '', 0.31764706, 0.68627451, 0.89019608) ;
#97782=CARTESIAN_POINT ( 'NONE',  ( 164.5367464035145133, 26.96999999999993847, 34.26648380511346659 ) ) ;
#97797=DIRECTION ( 'NONE',  ( 0.000000000000000000, 0.000000000000000000, 1.000000000000000000 ) ) ;
#97817=CARTESIAN_POINT ( 'NONE',  ( 24.39999999999999858, -1.600000000000060929, 28.92500000000001847 ) ) ;
#97820=FILL_AREA_STYLE ('',( #42034 ) ) ;
#97838=AXIS2_PLACEMENT_3D ( 'NONE', #109527, #65347, #43558 ) ;
#97843=LINE ( 'NONE', #55784, #95814 ) ;
#97847=( NAMED_UNIT ( * ) SI_UNIT ( $, .STERADIAN. ) SOLID_ANGLE_UNIT ( ) );
#97853=EDGE_LOOP ( 'NONE', ( #143003, #118361 ) ) ;
#97858=CARTESIAN_POINT ( 'NONE',  ( 6.337903141435219823, -6.871911579029513106, -3.967499999999993587 ) ) ;
#97867=ORIENTED_EDGE ( 'NONE', *, *, #16833, .T. ) ;
#97902=FILL_AREA_STYLE ('',( #9413 ) ) ;
#97903=CARTESIAN_POINT ( 'NONE',  ( 0.000000000000000000, -30.18000000000009564, -12.70000000000045404 ) ) ;
#97922=DIRECTION ( 'NONE',  ( 1.000000000000000000, 0.000000000000000000, 0.000000000000000000 ) ) ;
#97928=PLANE ( 'NONE',  #112142 ) ;
#97945=LINE ( 'NONE', #4, #28154 ) ;
#97965=FILL_AREA_STYLE_COLOUR ( '', #4324 ) ;
#98032=CARTESIAN_POINT ( 'NONE',  ( 17.27540314143521627, -2.126176841940958351, -7.934999999999989839 ) ) ;
#98035=ORIENTED_EDGE ( 'NONE', *, *, #93280, .T. ) ;
#98065=DIRECTION ( 'NONE',  ( 0.000000000000000000, -1.000000000000000000, 0.000000000000000000 ) ) ;
#98098=CARTESIAN_POINT ( 'NONE',  ( 0.2069207719830578884, 4.031931619714366200, -6.831241579940219744 ) ) ;
#98117=EDGE_CURVE ( 'NONE', #103874, #59558, #111313, .T. ) ;
#98124=CARTESIAN_POINT ( 'NONE',  ( 15.75000000000000000, -7.464222240803106570E-16, -6.094999999999989981 ) ) ;
#98192=VERTEX_POINT ( 'NONE', #78918 ) ;
#98204=CARTESIAN_POINT ( 'NONE',  ( 27.46247294953710849, -7.464222240803106570E-16, -6.094999999999989981 ) ) ;
#98244=ORIENTED_EDGE ( 'NONE', *, *, #18097, .T. ) ;
#98246=SURFACE_SIDE_STYLE ('',( #66344 ) ) ;
#98249=FILL_AREA_STYLE ('',( #142473 ) ) ;
#98274=UNCERTAINTY_MEASURE_WITH_UNIT (LENGTH_MEASURE( 1.000000000000000082E-05 ), #2621, 'distance_accuracy_value', 'NONE');
#98280=VECTOR ( 'NONE', #136251, 1000.000000000000000 ) ;
#98287=CARTESIAN_POINT ( 'NONE',  ( 156.1500000000000057, -49.14999999999999147, -49.92499999999968452 ) ) ;
#98288=CARTESIAN_POINT ( 'NONE',  ( 32.66666666666667140, -5.278424836066145431, -3.047499999999993658 ) ) ;
#98289=ORIENTED_EDGE ( 'NONE', *, *, #124570, .T. ) ;
#98296=VERTEX_POINT ( 'NONE', #89756 ) ;
#98306=CARTESIAN_POINT ( 'NONE',  ( 131.5423521607622774, -49.05583548141699168, -39.86617647058817226 ) ) ;
#98350=CARTESIAN_POINT ( 'NONE',  ( 184.1499999999998352, -47.62213595499959951, 36.92500000000000426 ) ) ;
#98389=MECHANICAL_DESIGN_GEOMETRIC_PRESENTATION_REPRESENTATION('',(#5732),#45132);
#98403=CARTESIAN_POINT ( 'NONE',  ( 13.54123647476855474, 0.000000000000000000, 7.934999999999990727 ) ) ;
#98436=FILL_AREA_STYLE_COLOUR ( '', #13824 ) ;
#98437=CYLINDRICAL_SURFACE ( 'NONE', #46938, 28.00000000000003197 ) ;
#98440=CARTESIAN_POINT ( 'NONE',  ( 6.708333333333333925, 3.047499999999997655, 5.278424836066143655 ) ) ;
#98441=CARTESIAN_POINT ( 'NONE',  ( 13.39540314143521904, 2.126176841940962348, 7.934999999999988951 ) ) ;
#98442=PRESENTATION_STYLE_ASSIGNMENT (( #9998 ) ) ;
#98449=CARTESIAN_POINT ( 'NONE',  ( 128.4365526510861173, -51.77943056867387384, -39.18578444878555445 ) ) ;
#98461=SURFACE_SIDE_STYLE ('',( #107877 ) ) ;
#98475=CARTESIAN_POINT ( 'NONE',  ( 126.7224180521722730, -45.84254607569121731, 35.55177538329068909 ) ) ;
#98477=VERTEX_POINT ( 'NONE', #53963 ) ;
#98494=AXIS2_PLACEMENT_3D ( 'NONE', #41954, #130395, #73861 ) ;
#98514=( NAMED_UNIT ( * ) SI_UNIT ( $, .STERADIAN. ) SOLID_ANGLE_UNIT ( ) );
#98558=CARTESIAN_POINT ( 'NONE',  ( 15.37956980810188767, 3.967499999999998916, 6.871911579029510442 ) ) ;
#98580=CARTESIAN_POINT ( 'NONE',  ( 153.4000000000000057, -16.48000000000005016, 34.92499999999998295 ) ) ;
#98585=EDGE_CURVE ( 'NONE', #109345, #119897, #46602, .T. ) ;
#98592=MECHANICAL_DESIGN_GEOMETRIC_PRESENTATION_REPRESENTATION('',(#84740),#119374);
#98603=LINE ( 'NONE', #21033, #71511 ) ;
#98611=ORIENTED_EDGE ( 'NONE', *, *, #118760, .T. ) ;
#98626=CARTESIAN_POINT ( 'NONE',  ( 23.04166666666666785, 3.047499999999993214, -5.278424836066146320 ) ) ;
#98641=MECHANICAL_DESIGN_GEOMETRIC_PRESENTATION_REPRESENTATION('',(#96323),#24649);
#98659=FILL_AREA_STYLE ('',( #97965 ) ) ;
#98679=VERTEX_POINT ( 'NONE', #5931 ) ;
#98707=ORIENTED_EDGE ( 'NONE', *, *, #82275, .T. ) ;
#98714=ADVANCED_FACE ( 'NONE', ( #105966 ), #88257, .F. ) ;
#98720=CARTESIAN_POINT ( 'NONE',  ( 15.96290314143521805, -3.967499999999994476, 6.871911579029513106 ) ) ;
#98752=AXIS2_PLACEMENT_3D ( 'NONE', #87837, #73410, #8790 ) ;
#98765=VERTEX_POINT ( 'NONE', #84959 ) ;
#98781=FILL_AREA_STYLE ('',( #120513 ) ) ;
#98819=CARTESIAN_POINT ( 'NONE',  ( 8.795806282870438864, -5.278424836066144543, 3.047499999999995879 ) ) ;
#98822=CARTESIAN_POINT ( 'NONE',  ( 14.29166666666666785, -3.047499999999994547, 5.278424836066145431 ) ) ;
#98824=CARTESIAN_POINT ( 'NONE',  ( 2.999999999999999112, -7.600000000000061817, 28.92499999999998650 ) ) ;
#98827=SURFACE_STYLE_FILL_AREA ( #121300 ) ;
#98834=CARTESIAN_POINT ( 'NONE',  ( 156.1500000000000057, -49.14999999999999147, 49.92499999999997584 ) ) ;
#98853=CARTESIAN_POINT ( 'NONE',  ( 0.000000000000000000, 0.000000000000000000, 0.000000000000000000 ) ) ;
#98888=CIRCLE ( 'NONE', #117399, 28.00000000000001776 ) ;
#98889=CARTESIAN_POINT ( 'NONE',  ( 20.75413961620377279, 3.047499999999993214, -5.278424836066146320 ) ) ;
#98923=CARTESIAN_POINT ( 'NONE',  ( 25.39999999999999858, -16.48000000000005016, -33.92499999999998295 ) ) ;
#98940=( LENGTH_UNIT ( ) NAMED_UNIT ( * ) SI_UNIT ( .MILLI., .METRE. ) );
#98944=AXIS2_PLACEMENT_3D ( 'NONE', #3558, #102917, #92020 ) ;
#98950=PRESENTATION_STYLE_ASSIGNMENT (( #65681 ) ) ;
#98963=AXIS2_PLACEMENT_3D ( 'NONE', #24692, #110255, #13084 ) ;
#98966=ADVANCED_FACE ( 'NONE', ( #93524, #24687 ), #102978, .F. ) ;
#98990=FILL_AREA_STYLE_COLOUR ( '', #101602 ) ;
#98999=ORIENTED_EDGE ( 'NONE', *, *, #79423, .T. ) ;
#99039=CARTESIAN_POINT ( 'NONE',  ( 181.1499999999998067, -49.85820393249933602, -34.92499999999995453 ) ) ;
#99049=( NAMED_UNIT ( * ) PLANE_ANGLE_UNIT ( ) SI_UNIT ( $, .RADIAN. ) );
#99077=CARTESIAN_POINT ( 'NONE',  ( 8.874569808101886892, 6.871911579029510442, -3.967499999999998916 ) ) ;
#99085=CARTESIAN_POINT ( 'NONE',  ( 19.68750000000000000, 4.461849672132297329, -4.461849672132302658 ) ) ;
#99119=CARTESIAN_POINT ( 'NONE',  ( 17.79166666666666785, -3.047499999999994547, 5.278424836066145431 ) ) ;
#99120=CARTESIAN_POINT ( 'NONE',  ( 17.62456980810188867, -6.871911579029512218, 3.967499999999996252 ) ) ;
#99134=PRESENTATION_STYLE_ASSIGNMENT (( #99881 ) ) ;
#99140=ADVANCED_FACE ( 'NONE', ( #38435 ), #140578, .F. ) ;
#99147=PRESENTATION_STYLE_ASSIGNMENT (( #32508 ) ) ;
#99175=CARTESIAN_POINT ( 'NONE',  ( 19.31706980810189123, -2.126176841940956130, 7.934999999999990727 ) ) ;
#99179=CARTESIAN_POINT ( 'NONE',  ( 3.302882771356463465, -48.98543874033774159, -39.51758185027075143 ) ) ;
#99191=COLOUR_RGB ( '', 0.31764706, 0.68627451, 0.89019608) ;
#99222=DIRECTION ( 'NONE',  ( -0.000000000000000000, 1.000000000000000000, -0.000000000000000000 ) ) ;
#99246=CARTESIAN_POINT ( 'NONE',  ( 15.23373647476855375, 5.808823158059036373, 5.808823158059032821 ) ) ;
#99293=( LENGTH_UNIT ( ) NAMED_UNIT ( * ) SI_UNIT ( .MILLI., .METRE. ) );
#99334=EDGE_CURVE ( 'NONE', #130484, #112167, #120825, .T. ) ;
#99337=AXIS2_PLACEMENT_3D ( 'NONE', #19767, #64004, #119770 ) ;
#99366=PRESENTATION_STYLE_ASSIGNMENT (( #44336 ) ) ;
#99369=AXIS2_PLACEMENT_3D ( 'NONE', #58418, #26452, #15526 ) ;
#99392=AXIS2_PLACEMENT_3D ( 'NONE', #90402, #46221, #79588 ) ;
#99422=CARTESIAN_POINT ( 'NONE',  ( 30.83790314143522338, -6.871911579029513106, -3.967499999999993587 ) ) ;
#99475=AXIS2_PLACEMENT_3D ( 'NONE', #56368, #89654, #133883 ) ;
#99577=EDGE_CURVE ( 'NONE', #119311, #111908, #109244, .T. ) ;
#99586=VECTOR ( 'NONE', #19380, 1000.000000000000000 ) ;
#99596=CARTESIAN_POINT ( 'NONE',  ( 27.60830628287043709, 1.633150327867687324, -6.094999999999991758 ) ) ;
#99637=FILL_AREA_STYLE ('',( #56901 ) ) ;
#99666=CARTESIAN_POINT ( 'NONE',  ( 25.39999999999999858, -18.48000000000005372, 34.92499999999998295 ) ) ;
#99673=UNCERTAINTY_MEASURE_WITH_UNIT (LENGTH_MEASURE( 1.000000000000000082E-05 ), #104116, 'distance_accuracy_value', 'NONE');
#99708=DIRECTION ( 'NONE',  ( -0.000000000000000000, -0.9976538855070752332, -0.06845965770171358322 ) ) ;
#99711=( NAMED_UNIT ( * ) PLANE_ANGLE_UNIT ( ) SI_UNIT ( $, .RADIAN. ) );
#99719=ORIENTED_EDGE ( 'NONE', *, *, #125526, .T. ) ;
#99734=EDGE_CURVE ( 'NONE', #55981, #136091, #90757, .T. ) ;
#99737=LINE ( 'NONE', #33797, #115104 ) ;
#99745=CARTESIAN_POINT ( 'NONE',  ( 0.000000000000000000, -4.600000000000061817, 28.92500000000000426 ) ) ;
#99748=SURFACE_STYLE_USAGE ( .BOTH. , #55555 ) ;
#99756=COLOUR_RGB ( '', 0.08235294, 0.09019608, 0.10196078) ;
#99782=CARTESIAN_POINT ( 'NONE',  ( 1.358306282870439308, -1.633150327867689988, 6.094999999999989981 ) ) ;
#99786=VERTEX_POINT ( 'NONE', #134573 ) ;
#99819=CARTESIAN_POINT ( 'NONE',  ( 16.60373647476855297, 5.808823158059036373, 5.808823158059032821 ) ) ;
#99861=PRESENTATION_STYLE_ASSIGNMENT (( #76716 ) ) ;
#99865=CARTESIAN_POINT ( 'NONE',  ( 14.00000000000000178, 0.000000000000000000, 6.094999999999989981 ) ) ;
#99867=CARTESIAN_POINT ( 'NONE',  ( 25.30244920428738453, -6.182694495602187423, -5.161259005940558531 ) ) ;
#99881=SURFACE_STYLE_USAGE ( .BOTH. , #54967 ) ;
#99907=CARTESIAN_POINT ( 'NONE',  ( 184.1374510928294512, -50.57777258831012546, 35.91905586107260717 ) ) ;
#99912=ORIENTED_EDGE ( 'NONE', *, *, #1454, .F. ) ;
#99919=( GEOMETRIC_REPRESENTATION_CONTEXT ( 3 ) GLOBAL_UNCERTAINTY_ASSIGNED_CONTEXT ( ( #67965 ) ) GLOBAL_UNIT_ASSIGNED_CONTEXT ( ( #30207, #85287, #28804 ) ) REPRESENTATION_CONTEXT ( 'NONE', 'WORKASPACE' ) );
#99927=CARTESIAN_POINT ( 'NONE',  ( 17.71290314143521982, 3.967499999999992699, -6.871911579029513994 ) ) ;
#99930=CARTESIAN_POINT ( 'NONE',  ( 165.4899822245387782, 26.96999999999994202, 33.83144603466802636 ) ) ;
#99968=SURFACE_STYLE_FILL_AREA ( #97820 ) ;
#99981=CARTESIAN_POINT ( 'NONE',  ( 152.4000000000000057, -16.48000000000005016, -33.92499999999998295 ) ) ;
#100002=CARTESIAN_POINT ( 'NONE',  ( 19.90040314143521982, -7.934999999999989839, 2.126176841940957907 ) ) ;
#100016=ADVANCED_FACE ( 'NONE', ( #109767 ), #75724, .F. ) ;
#100022=CYLINDRICAL_SURFACE ( 'NONE', #10944, 1.000000000000000888 ) ;
#100041=FACE_OUTER_BOUND ( 'NONE', #94663, .T. ) ;
#100050=CARTESIAN_POINT ( 'NONE',  ( 21.70790314143522082, -6.871911579029513106, -3.967499999999993587 ) ) ;
#100081=ORIENTED_EDGE ( 'NONE', *, *, #32387, .F. ) ;
#100126=SURFACE_STYLE_USAGE ( .BOTH. , #112423 ) ;
#100177=CARTESIAN_POINT ( 'NONE',  ( 27.33790314143521982, -6.871911579029513106, -3.967499999999993587 ) ) ;
#100204=ORIENTED_EDGE ( 'NONE', *, *, #124972, .F. ) ;
#100213=ORIENTED_EDGE ( 'NONE', *, *, #2569, .F. ) ;
#100240=CARTESIAN_POINT ( 'NONE',  ( 0.4678577423086575093, 6.868554027058086042, -3.322579193147489285 ) ) ;
#100261=SURFACE_STYLE_USAGE ( .BOTH. , #110389 ) ;
#100277=SURFACE_STYLE_FILL_AREA ( #5009 ) ;
#100279=SURFACE_SIDE_STYLE ('',( #98827 ) ) ;
#100283=VERTEX_POINT ( 'NONE', #60972 ) ;
#100347=CARTESIAN_POINT ( 'NONE',  ( 31.10830628287042998, 1.633150327867687324, -6.094999999999991758 ) ) ;
#100382=FILL_AREA_STYLE ('',( #22075 ) ) ;
#100384=EDGE_CURVE ( 'NONE', #143396, #34958, #44931, .T. ) ;
#100390=ORIENTED_EDGE ( 'NONE', *, *, #26776, .F. ) ;
#100414=STYLED_ITEM ( 'NONE', ( #100974 ), #79637 ) ;
#100466=CIRCLE ( 'NONE', #114313, 2.999999999999999112 ) ;
#100496=CARTESIAN_POINT ( 'NONE',  ( 4.274972949537105826, 4.461849672132300881, 4.461849672132299105 ) ) ;
#100519=CARTESIAN_POINT ( 'NONE',  ( 5.879139616203772789, -5.278424836066145431, -3.047499999999993658 ) ) ;
#100537=PLANE ( 'NONE',  #44770 ) ;
#100541=CARTESIAN_POINT ( 'NONE',  ( 52.60764783923757193, -49.05583548141699879, 39.86617647058822200 ) ) ;
#100546=CARTESIAN_POINT ( 'NONE',  ( 14.41623647476855297, -7.934999999999990727, 4.858786175617117713E-16 ) ) ;
#100557=CARTESIAN_POINT ( 'NONE',  ( 21.00000000000000000, 0.000000000000000000, 6.094999999999989981 ) ) ;
#100569=ORIENTED_EDGE ( 'NONE', *, *, #105631, .T. ) ;
#100581=SURFACE_STYLE_FILL_AREA ( #76706 ) ;
#100589=SURFACE_STYLE_FILL_AREA ( #112873 ) ;
#100597=CARTESIAN_POINT ( 'NONE',  ( 14.14583333333333570, -1.633150327867689988, 6.094999999999989981 ) ) ;
#100651=CARTESIAN_POINT ( 'NONE',  ( 21.79623647476855552, 7.934999999999990727, -1.457635852685135314E-15 ) ) ;
#100674=( NAMED_UNIT ( * ) SI_UNIT ( $, .STERADIAN. ) SOLID_ANGLE_UNIT ( ) );
#100689=CARTESIAN_POINT ( 'NONE',  ( 0.000000000000000000, -7.600000000000060041, 31.92499999999998295 ) ) ;
#100698=VERTEX_POINT ( 'NONE', #107797 ) ;
#100699=FACE_OUTER_BOUND ( 'NONE', #95275, .T. ) ;
#100718=CARTESIAN_POINT ( 'NONE',  ( 21.79623647476855552, 7.934999999999990727, -1.457635852685135314E-15 ) ) ;
#100744=SURFACE_STYLE_FILL_AREA ( #91320 ) ;
#100755=CARTESIAN_POINT ( 'NONE',  ( 24.47873647476856007, -5.808823158059033709, 5.808823158059035485 ) ) ;
#100779=( NAMED_UNIT ( * ) SI_UNIT ( $, .STERADIAN. ) SOLID_ANGLE_UNIT ( ) );
#100796=DIRECTION ( 'NONE',  ( 0.000000000000000000, 0.06845965770171351383, -0.9976538855070752332 ) ) ;
#100812=DIRECTION ( 'NONE',  ( 0.000000000000000000, -0.000000000000000000, 1.000000000000000000 ) ) ;
#100819=EDGE_CURVE ( 'NONE', #134245, #97576, #116497, .T. ) ;
#100823=ORIENTED_EDGE ( 'NONE', *, *, #33078, .T. ) ;
#100827=FILL_AREA_STYLE ('',( #101529 ) ) ;
#100837=CARTESIAN_POINT ( 'NONE',  ( 25.12913961620377279, 5.278424836066147208, 3.047499999999990550 ) ) ;
#100852=MECHANICAL_DESIGN_GEOMETRIC_PRESENTATION_REPRESENTATION('',(#107469),#110053);
#100870=CARTESIAN_POINT ( 'NONE',  ( 25.29623647476855908, 7.934999999999990727, -1.457635852685135314E-15 ) ) ;
#100883=ORIENTED_EDGE ( 'NONE', *, *, #137151, .F. ) ;
#100889=CARTESIAN_POINT ( 'NONE',  ( 61.46640106136307935, -43.14999999999999147, 34.92499999999998295 ) ) ;
#100890=DIRECTION ( 'NONE',  ( -1.000000000000000000, -0.000000000000000000, -0.000000000000000000 ) ) ;
#100912=CARTESIAN_POINT ( 'NONE',  ( 180.4193221990230143, -52.14999999999999147, 40.92499999999998295 ) ) ;
#100924=CARTESIAN_POINT ( 'NONE',  ( 1.666965064704732269, -1.287028696899377367E-11, -6.428034935295263708 ) ) ;
#100925=CARTESIAN_POINT ( 'NONE',  ( 176.2838169021916599, 7.919999999999943086, -18.97500000000001918 ) ) ;
#100935=SURFACE_STYLE_USAGE ( .BOTH. , #43708 ) ;
#100945=ORIENTED_EDGE ( 'NONE', *, *, #13984, .F. ) ;
#100963=CARTESIAN_POINT ( 'NONE',  ( 152.4000000000000057, 25.96999999999993847, -33.92499999999998295 ) ) ;
#100972=EDGE_CURVE ( 'NONE', #60071, #117911, #103343, .T. ) ;
#100974=PRESENTATION_STYLE_ASSIGNMENT (( #88699 ) ) ;
#101034=CARTESIAN_POINT ( 'NONE',  ( 0.7962364747685526378, 7.934999999999990727, -1.457635852685135314E-15 ) ) ;
#101045=( NAMED_UNIT ( * ) SI_UNIT ( $, .STERADIAN. ) SOLID_ANGLE_UNIT ( ) );
#101065=DIRECTION ( 'NONE',  ( 0.000000000000000000, 1.000000000000000000, -0.000000000000000000 ) ) ;
#101079=( NAMED_UNIT ( * ) PLANE_ANGLE_UNIT ( ) SI_UNIT ( $, .RADIAN. ) );
#101105=UNCERTAINTY_MEASURE_WITH_UNIT (LENGTH_MEASURE( 1.000000000000000082E-05 ), #21990, 'distance_accuracy_value', 'NONE');
#101126=STYLED_ITEM ( 'NONE', ( #125561 ), #11702 ) ;
#101131=FACE_OUTER_BOUND ( 'NONE', #34534, .T. ) ;
#101164=VECTOR ( 'NONE', #124537, 1000.000000000000000 ) ;
#101183=MECHANICAL_DESIGN_GEOMETRIC_PRESENTATION_REPRESENTATION('',(#115025),#94248);
#101192=CARTESIAN_POINT ( 'NONE',  ( 25.40000000000000213, 7.943993692193106249, -0.1521560028100145123 ) ) ;
#101209=CARTESIAN_POINT ( 'NONE',  ( 3.108306282870439752, 1.633150327867687324, -6.094999999999991758 ) ) ;
#101228=FILL_AREA_STYLE ('',( #123731 ) ) ;
#101231=FACE_OUTER_BOUND ( 'NONE', #103679, .T. ) ;
#101242=CARTESIAN_POINT ( 'NONE',  ( 22.14540314143522082, -2.126176841940958351, -7.934999999999989839 ) ) ;
#101291=CARTESIAN_POINT ( 'NONE',  ( 12.39583333333333570, 1.633150327867687324, -6.094999999999991758 ) ) ;
#101304=FACE_OUTER_BOUND ( 'NONE', #140612, .T. ) ;
#101306=CARTESIAN_POINT ( 'NONE',  ( 125.9828883629132434, -46.44928942427409169, -35.85226645762418940 ) ) ;
#101346=CARTESIAN_POINT ( 'NONE',  ( 21.06706980810188412, 2.126176841940952134, -7.934999999999992504 ) ) ;
#101347=CARTESIAN_POINT ( 'NONE',  ( 25.40000000000000924, -6.239863630333645439, -0.7640341322893426934 ) ) ;
#101348=( NAMED_UNIT ( * ) SI_UNIT ( $, .STERADIAN. ) SOLID_ANGLE_UNIT ( ) );
#101370=AXIS2_PLACEMENT_3D ( 'NONE', #25577, #11836, #56119 ) ;
#101398=ORIENTED_EDGE ( 'NONE', *, *, #95325, .T. ) ;
#101403=CARTESIAN_POINT ( 'NONE',  ( 14.04580628287044064, 5.278424836066143655, -3.047499999999997655 ) ) ;
#101412=CARTESIAN_POINT ( 'NONE',  ( 21.50456980810188412, 6.871911579029510442, -3.967499999999998916 ) ) ;
#101448=DIRECTION ( 'NONE',  ( 0.000000000000000000, -1.000000000000000000, 0.000000000000000000 ) ) ;
#101456=CARTESIAN_POINT ( 'NONE',  ( 17.62456980810188867, -6.871911579029512218, 3.967499999999996252 ) ) ;
#101496=LINE ( 'NONE', #113808, #1689 ) ;
#101524=CARTESIAN_POINT ( 'NONE',  ( 26.40000000000000568, -16.48000000000005016, 34.92499999999998295 ) ) ;
#101529=FILL_AREA_STYLE_COLOUR ( '', #4237 ) ;
#101543=ORIENTED_EDGE ( 'NONE', *, *, #116370, .F. ) ;
#101571=STYLED_ITEM ( 'NONE', ( #42603 ), #124980 ) ;
#101574=CARTESIAN_POINT ( 'NONE',  ( 25.15040314143521627, 7.934999999999989839, -2.126176841940961904 ) ) ;
#101584=LINE ( 'NONE', #2246, #31044 ) ;
#101598=( GEOMETRIC_REPRESENTATION_CONTEXT ( 3 ) GLOBAL_UNCERTAINTY_ASSIGNED_CONTEXT ( ( #79421 ) ) GLOBAL_UNIT_ASSIGNED_CONTEXT ( ( #126590, #27281, #139669 ) ) REPRESENTATION_CONTEXT ( 'NONE', 'WORKASPACE' ) );
#101602=COLOUR_RGB ( '', 0.40784314, 0.44705882, 0.49803922) ;
#101614=( GEOMETRIC_REPRESENTATION_CONTEXT ( 3 ) GLOBAL_UNCERTAINTY_ASSIGNED_CONTEXT ( ( #44818 ) ) GLOBAL_UNIT_ASSIGNED_CONTEXT ( ( #99293, #103583, #136224 ) ) REPRESENTATION_CONTEXT ( 'NONE', 'WORKASPACE' ) );
#101637=EDGE_CURVE ( 'NONE', #11327, #53362, #100466, .T. ) ;
#101638=CARTESIAN_POINT ( 'NONE',  ( 1.425881352870889796, -2.124795774637151080, -6.328817049275281548 ) ) ;
#101642=CARTESIAN_POINT ( 'NONE',  ( 127.2418942207595478, -46.18886352141520035, 34.92499999999998295 ) ) ;
#101650=EDGE_CURVE ( 'NONE', #92907, #34958, #74885, .T. ) ;
#101652=CARTESIAN_POINT ( 'NONE',  ( 0.6405549847417550957, 7.449887432306902646, -0.4886591319612960671 ) ) ;
#101672=STYLED_ITEM ( 'NONE', ( #86386 ), #939 ) ;
#101678=CARTESIAN_POINT ( 'NONE',  ( 153.4000000000000057, 26.96999999999993847, -34.92499999999998295 ) ) ;
#101705=( GEOMETRIC_REPRESENTATION_CONTEXT ( 3 ) GLOBAL_UNCERTAINTY_ASSIGNED_CONTEXT ( ( #21424 ) ) GLOBAL_UNIT_ASSIGNED_CONTEXT ( ( #3737, #92197, #81374 ) ) REPRESENTATION_CONTEXT ( 'NONE', 'WORKASPACE' ) );
#101706=DIRECTION ( 'NONE',  ( 0.000000000000000000, 0.000000000000000000, -1.000000000000000000 ) ) ;
#101757=CARTESIAN_POINT ( 'NONE',  ( -1.682930191898113881, -2.126176841940956130, 7.934999999999991616 ) ) ;
#101777=MECHANICAL_DESIGN_GEOMETRIC_PRESENTATION_REPRESENTATION('',(#39178),#104021);
#101780=LINE ( 'NONE', #80074, #76031 ) ;
#101790=COLOUR_RGB ( '', 0.09019608, 0.27058824, 0.51372549) ;
#101792=CARTESIAN_POINT ( 'NONE',  ( 0.1245698081018861286, -6.871911579029512218, 3.967499999999996252 ) ) ;
#101801=SURFACE_STYLE_FILL_AREA ( #3192 ) ;
#101831=CARTESIAN_POINT ( 'NONE',  ( 0.000000000000000000, -7.600000000000061817, 28.92499999999998650 ) ) ;
#101861=SURFACE_STYLE_USAGE ( .BOTH. , #91017 ) ;
#101892=DIRECTION ( 'NONE',  ( 0.000000000000000000, 0.000000000000000000, 1.000000000000000000 ) ) ;
#101926=ORIENTED_EDGE ( 'NONE', *, *, #118658, .F. ) ;
#101931=CARTESIAN_POINT ( 'NONE',  ( 7.774972949537104938, 4.461849672132300881, 4.461849672132299105 ) ) ;
#101963=CARTESIAN_POINT ( 'NONE',  ( 21.99956980810188867, -3.967499999999998028, -6.871911579029511330 ) ) ;
#102011=CARTESIAN_POINT ( 'NONE',  ( 14.29166666666666785, -3.047499999999994547, 5.278424836066145431 ) ) ;
#102012=CARTESIAN_POINT ( 'NONE',  ( 22.58290314143522082, 3.967499999999992699, -6.871911579029513994 ) ) ;
#102068=CARTESIAN_POINT ( 'NONE',  ( 24.56706980810188767, 2.126176841940952134, -7.934999999999992504 ) ) ;
#102081=EDGE_CURVE ( 'NONE', #98477, #25649, #56910, .T. ) ;
#102086=( BOUNDED_SURFACE ( )  B_SPLINE_SURFACE ( 3, 2, ( 
 ( #72594, #26885, #71131 ),
 ( #93580, #86980, #65980 ),
 ( #21728, #141356, #76110 ),
 ( #131202, #42070, #97095 ) ),
 .UNSPECIFIED., .F., .F., .F. ) 
 B_SPLINE_SURFACE_WITH_KNOTS ( ( 4, 4 ),
 ( 3, 3 ),
 ( -4.336808689942017736E-19, 0.001630001914283392113 ),
 ( 0.000000000000000000, 1.000000000000000000 ),
 .UNSPECIFIED. ) 
 GEOMETRIC_REPRESENTATION_ITEM ( )  RATIONAL_B_SPLINE_SURFACE ( (
 ( 1.000000000000000000, 0.7180326832784531543, 1.000000000000000000),
 ( 1.000000000000000000, 0.7157206429707758666, 1.000000000000000000),
 ( 1.000000000000000000, 0.7121002461815039153, 1.000000000000000000),
 ( 1.000000000000000000, 0.7071067811865475727, 1.000000000000000000) ) ) 
 REPRESENTATION_ITEM ( '' )  SURFACE ( )  );
#102099=( BOUNDED_CURVE ( )  B_SPLINE_CURVE ( 3, ( #68206, #134875, #110207, #36252 ),
 .UNSPECIFIED., .F., .T. ) 
 B_SPLINE_CURVE_WITH_KNOTS ( ( 4, 4 ),
 ( 4.712388980384689674, 6.283185307179586232 ),
 .UNSPECIFIED. ) 
 CURVE ( )  GEOMETRIC_REPRESENTATION_ITEM ( )  RATIONAL_B_SPLINE_CURVE ( ( 1.000000000000000000, 0.8047378541243649375, 0.8047378541243649375, 1.000000000000000000 ) ) 
 REPRESENTATION_ITEM ( '' )  );
#102104=EDGE_CURVE ( 'NONE', #16103, #113523, #139593, .T. ) ;
#102105=( LENGTH_UNIT ( ) NAMED_UNIT ( * ) SI_UNIT ( .MILLI., .METRE. ) );
#102135=EDGE_CURVE ( 'NONE', #75508, #58706, #79386, .T. ) ;
#102153=CARTESIAN_POINT ( 'NONE',  ( 29.08790314143522338, 6.871911579029515771, 3.967499999999989146 ) ) ;
#102154=ORIENTED_EDGE ( 'NONE', *, *, #119046, .F. ) ;
#102160=( GEOMETRIC_REPRESENTATION_CONTEXT ( 3 ) GLOBAL_UNCERTAINTY_ASSIGNED_CONTEXT ( ( #11554 ) ) GLOBAL_UNIT_ASSIGNED_CONTEXT ( ( #123803, #70165, #5542 ) ) REPRESENTATION_CONTEXT ( 'NONE', 'WORKASPACE' ) );
#102173=ORIENTED_EDGE ( 'NONE', *, *, #95325, .F. ) ;
#102195=CARTESIAN_POINT ( 'NONE',  ( 17.04123647476855652, 0.000000000000000000, 7.934999999999990727 ) ) ;
#102228=VECTOR ( 'NONE', #123476, 1000.000000000000000 ) ;
#102275=SURFACE_STYLE_FILL_AREA ( #110947 ) ;
#102311=DIRECTION ( 'NONE',  ( 0.000000000000000000, -1.000000000000000000, 0.000000000000000000 ) ) ;
#102330=CARTESIAN_POINT ( 'NONE',  ( 28.35873647476855197, 5.808823158059031044, -5.808823158059038150 ) ) ;
#102331=CARTESIAN_POINT ( 'NONE',  ( 4.442069808101886785, 7.934999999999993392, 2.126176841940951689 ) ) ;
#102335=CARTESIAN_POINT ( 'NONE',  ( 3.000000000000000000, 0.9892420537897055333, 14.41609864557725729 ) ) ;
#102337=FILL_AREA_STYLE ('',( #58139 ) ) ;
#102343=FILL_AREA_STYLE ('',( #5102 ) ) ;
#102413=ORIENTED_EDGE ( 'NONE', *, *, #54675, .T. ) ;
#102429=( GEOMETRIC_REPRESENTATION_CONTEXT ( 3 ) GLOBAL_UNCERTAINTY_ASSIGNED_CONTEXT ( ( #88281 ) ) GLOBAL_UNIT_ASSIGNED_CONTEXT ( ( #66192, #56049, #43010 ) ) REPRESENTATION_CONTEXT ( 'NONE', 'WORKASPACE' ) );
#102451=EDGE_CURVE ( 'NONE', #137006, #71833, #14868, .T. ) ;
#102455=AXIS2_PLACEMENT_3D ( 'NONE', #70782, #38143, #79546 ) ;
#102463=DIRECTION ( 'NONE',  ( 0.000000000000000000, 1.000000000000000000, 0.000000000000000000 ) ) ;
#102477=AXIS2_PLACEMENT_3D ( 'NONE', #28750, #117145, #17826 ) ;
#102500=CARTESIAN_POINT ( 'NONE',  ( 1.379569808101885897, 3.967499999999998916, 6.871911579029510442 ) ) ;
#102510=ORIENTED_EDGE ( 'NONE', *, *, #85776, .F. ) ;
#102511=DIRECTION ( 'NONE',  ( 0.000000000000000000, 1.000000000000000000, 0.000000000000000000 ) ) ;
#102512=CARTESIAN_POINT ( 'NONE',  ( 26.40000000000000568, -18.48000000000005372, 34.92499999999998295 ) ) ;
#102527=CARTESIAN_POINT ( 'NONE',  ( 6.462472949537106715, -7.464222240803106570E-16, -6.094999999999989981 ) ) ;
#102533=PLANE ( 'NONE',  #17792 ) ;
#102535=DIRECTION ( 'NONE',  ( 1.000000000000000000, 0.000000000000000000, 0.000000000000000000 ) ) ;
#102547=CARTESIAN_POINT ( 'NONE',  ( 184.1500000000000057, -49.85820393249935023, -34.92499999999998295 ) ) ;
#102599=DIRECTION ( 'NONE',  ( 0.000000000000000000, 0.6666666666666630769, -0.7453559924999331177 ) ) ;
#102640=ADVANCED_FACE ( 'NONE', ( #69757 ), #5136, .F. ) ;
#102648=SURFACE_STYLE_USAGE ( .BOTH. , #35266 ) ;
#102665=CARTESIAN_POINT ( 'NONE',  ( 4.274972949537106715, 4.461849672132300881, 4.461849672132299105 ) ) ;
#102674=EDGE_LOOP ( 'NONE', ( #40817, #29459, #87682, #43436 ) ) ;
#102686=SURFACE_STYLE_FILL_AREA ( #37422 ) ;
#102692=CARTESIAN_POINT ( 'NONE',  ( 25.93706980810189222, 2.126176841940952134, -7.934999999999993392 ) ) ;
#102710=PRODUCT_DEFINITION_FORMATION_WITH_SPECIFIED_SOURCE ( 'ANY', '', #72462, .NOT_KNOWN. ) ;
#102724=FILL_AREA_STYLE ('',( #38187 ) ) ;
#102736=CARTESIAN_POINT ( 'NONE',  ( 25.08333333333333570, -5.278424836066144543, 3.047499999999995879 ) ) ;
#102749=CARTESIAN_POINT ( 'NONE',  ( 125.0591050317621011, -46.71325913968131260, -35.40428284070993215 ) ) ;
#102797=FILL_AREA_STYLE_COLOUR ( '', #96355 ) ;
#102798=CARTESIAN_POINT ( 'NONE',  ( 22.67123647476855552, 0.000000000000000000, 7.934999999999990727 ) ) ;
#102864=CARTESIAN_POINT ( 'NONE',  ( 26.90040314143521627, -7.934999999999989839, 2.126176841940957907 ) ) ;
#102905=CARTESIAN_POINT ( 'NONE',  ( 30.02040314143521726, 7.934999999999989839, -2.126176841940961904 ) ) ;
#102917=DIRECTION ( 'NONE',  ( -0.000000000000000000, 1.000000000000000000, 2.921639538487157626E-15 ) ) ;
#102927=DIRECTION ( 'NONE',  ( -0.000000000000000000, -0.000000000000000000, 1.000000000000000000 ) ) ;
#102934=( NAMED_UNIT ( * ) SI_UNIT ( $, .STERADIAN. ) SOLID_ANGLE_UNIT ( ) );
#102978=PLANE ( 'NONE',  #93007 ) ;
#102998=( LENGTH_UNIT ( ) NAMED_UNIT ( * ) SI_UNIT ( .MILLI., .METRE. ) );
#103004=FILL_AREA_STYLE ('',( #108845 ) ) ;
#103010=PRESENTATION_STYLE_ASSIGNMENT (( #137068 ) ) ;
#103023=CARTESIAN_POINT ( 'NONE',  ( 4.587903141435219823, 6.871911579029515771, 3.967499999999989146 ) ) ;
#103036=CARTESIAN_POINT ( 'NONE',  ( 61.46640106136307935, -57.15000000000010516, 40.92499999999998295 ) ) ;
#103038=( NAMED_UNIT ( * ) PLANE_ANGLE_UNIT ( ) SI_UNIT ( $, .RADIAN. ) );
#103047=ORIENTED_EDGE ( 'NONE', *, *, #30098, .T. ) ;
#103054=EDGE_LOOP ( 'NONE', ( #76726, #110855, #117019, #10648, #94100 ) ) ;
#103055=STYLED_ITEM ( 'NONE', ( #110501 ), #120064 ) ;
#103094=CARTESIAN_POINT ( 'NONE',  ( 0.6891546199041412857, 7.409644225788786009, 0.3384941017316204226 ) ) ;
#103147=SURFACE_STYLE_USAGE ( .BOTH. , #49524 ) ;
#103182=CARTESIAN_POINT ( 'NONE',  ( 4.879569808101885897, 3.967499999999998916, 6.871911579029510442 ) ) ;
#103203=CARTESIAN_POINT ( 'NONE',  ( 7.337472949537107603, 6.094999999999989981, -1.119633336120465690E-15 ) ) ;
#103210=CARTESIAN_POINT ( 'NONE',  ( 5.520403141435220817, 7.934999999999989839, -2.126176841940961904 ) ) ;
#103275=DIRECTION ( 'NONE',  ( 0.000000000000000000, -1.000000000000000000, 0.000000000000000000 ) ) ;
#103316=CARTESIAN_POINT ( 'NONE',  ( 25.40000000000004121, 7.384918846911211254, -2.931050874386697203 ) ) ;
#103335=CARTESIAN_POINT ( 'NONE',  ( 5.587472949537105826, -6.094999999999989981, 3.732111120401553285E-16 ) ) ;
#103343=LINE ( 'NONE', #23663, #58707 ) ;
#103356=( NAMED_UNIT ( * ) SI_UNIT ( $, .STERADIAN. ) SOLID_ANGLE_UNIT ( ) );
#103362=CARTESIAN_POINT ( 'NONE',  ( 22.58290314143522082, 3.967499999999992699, -6.871911579029513994 ) ) ;
#103414=CARTESIAN_POINT ( 'NONE',  ( 20.27083333333333570, 6.094999999999991758, 1.633150327867687102 ) ) ;
#103426=DIRECTION ( 'NONE',  ( 1.000000000000000000, 0.000000000000000000, -0.000000000000000000 ) ) ;
#103450=DIRECTION ( 'NONE',  ( 0.000000000000000000, 0.000000000000000000, 1.000000000000000000 ) ) ;
#103455=DIRECTION ( 'NONE',  ( -1.000000000000000000, 0.000000000000000000, 0.000000000000000000 ) ) ;
#103467=SURFACE_STYLE_USAGE ( .BOTH. , #25939 ) ;
#103468=CARTESIAN_POINT ( 'NONE',  ( 22.08790314143522338, 6.871911579029515771, 3.967499999999989146 ) ) ;
#103535=CARTESIAN_POINT ( 'NONE',  ( 26.17123647476855908, 0.000000000000000000, 7.934999999999990727 ) ) ;
#103546=SURFACE_STYLE_USAGE ( .BOTH. , #125335 ) ;
#103548=CARTESIAN_POINT ( 'NONE',  ( 25.40000000000000568, -6.088644610809077484, -0.2782657062331916342 ) ) ;
#103583=( NAMED_UNIT ( * ) PLANE_ANGLE_UNIT ( ) SI_UNIT ( $, .RADIAN. ) );
#103584=CARTESIAN_POINT ( 'NONE',  ( 31.18706980810189222, -2.126176841940956130, 7.934999999999991616 ) ) ;
#103600=CARTESIAN_POINT ( 'NONE',  ( 151.4000000000000057, -16.48000000000005016, 12.69999999999954632 ) ) ;
#103601=DIRECTION ( 'NONE',  ( -1.000000000000000000, -0.000000000000000000, -0.000000000000000000 ) ) ;
#103635=CARTESIAN_POINT ( 'NONE',  ( 3.129569808101886341, -3.967499999999998028, -6.871911579029511330 ) ) ;
#103637=STYLED_ITEM ( 'NONE', ( #16864 ), #137549 ) ;
#103648=PRESENTATION_STYLE_ASSIGNMENT (( #25390 ) ) ;
#103656=FILL_AREA_STYLE ('',( #83378 ) ) ;
#103672=DIRECTION ( 'NONE',  ( 0.000000000000000000, -1.286409696682840916E-16, 1.000000000000000000 ) ) ;
#103679=EDGE_LOOP ( 'NONE', ( #44454, #42947, #36026, #81055, #121127, #113489, #6513, #99719, #115976, #40121 ) ) ;
#103696=DIRECTION ( 'NONE',  ( 0.000000000000000000, 0.000000000000000000, -1.000000000000000000 ) ) ;
#103698=CARTESIAN_POINT ( 'NONE',  ( -1.391263525231447584, -5.808823158059033709, 5.808823158059035485 ) ) ;
#103708=ORIENTED_EDGE ( 'NONE', *, *, #79207, .F. ) ;
#103714=CARTESIAN_POINT ( 'NONE',  ( 180.4193221990229574, -49.14999999999999147, -40.92499999999998295 ) ) ;
#103747=EDGE_CURVE ( 'NONE', #143089, #97576, #21948, .T. ) ;
#103757=( LENGTH_UNIT ( ) NAMED_UNIT ( * ) SI_UNIT ( .MILLI., .METRE. ) );
#103772=( NAMED_UNIT ( * ) SI_UNIT ( $, .STERADIAN. ) SOLID_ANGLE_UNIT ( ) );
#103822=STYLED_ITEM ( 'NONE', ( #99366 ), #113202 ) ;
#103828=CARTESIAN_POINT ( 'NONE',  ( 8.750000000000000000, -7.464222240803106570E-16, -6.094999999999989981 ) ) ;
#103843=DIRECTION ( 'NONE',  ( -0.5150380749100710309, 0.000000000000000000, 0.8571673007021021196 ) ) ;
#103872=CARTESIAN_POINT ( 'NONE',  ( 8.962903141435219823, -3.967499999999994476, 6.871911579029513106 ) ) ;
#103874=VERTEX_POINT ( 'NONE', #28395 ) ;
#103878=CARTESIAN_POINT ( 'NONE',  ( 25.22916666666666785, -6.094999999999989093, 1.633150327867691542 ) ) ;
#103898=CARTESIAN_POINT ( 'NONE',  ( 7.920806282870441528, 3.047499999999997655, 5.278424836066143655 ) ) ;
#103906=CARTESIAN_POINT ( 'NONE',  ( 1.582903141435219485, 3.967499999999992699, -6.871911579029513994 ) ) ;
#103911=ORIENTED_EDGE ( 'NONE', *, *, #112719, .F. ) ;
#103918=SURFACE_SIDE_STYLE ('',( #69948 ) ) ;
#103967=DIRECTION ( 'NONE',  ( -1.000000000000000000, 0.000000000000000000, 0.000000000000000000 ) ) ;
#103972=LINE ( 'NONE', #106844, #117826 ) ;
#103980=DIRECTION ( 'NONE',  ( 0.000000000000000000, -1.000000000000000000, 0.000000000000000000 ) ) ;
#104004=VERTEX_POINT ( 'NONE', #18178 ) ;
#104021=( GEOMETRIC_REPRESENTATION_CONTEXT ( 3 ) GLOBAL_UNCERTAINTY_ASSIGNED_CONTEXT ( ( #110168 ) ) GLOBAL_UNIT_ASSIGNED_CONTEXT ( ( #92059, #58795, #36278 ) ) REPRESENTATION_CONTEXT ( 'NONE', 'WORKASPACE' ) );
#104027=CARTESIAN_POINT ( 'NONE',  ( 0.000000000000000000, -14.29000000000013593, -12.70000000000045404 ) ) ;
#104040=CARTESIAN_POINT ( 'NONE',  ( 14.19163961620377101, 6.094999999999988205, -1.633150327867694651 ) ) ;
#104044=SURFACE_STYLE_FILL_AREA ( #80220 ) ;
#104049=ORIENTED_EDGE ( 'NONE', *, *, #99734, .F. ) ;
#104063=FILL_AREA_STYLE_COLOUR ( '', #83937 ) ;
#104071=ADVANCED_FACE ( 'NONE', ( #140696 ), #97928, .F. ) ;
#104072=CARTESIAN_POINT ( 'NONE',  ( 19.95790314143522437, 6.871911579029515771, 3.967499999999989146 ) ) ;
#104080=PRESENTATION_STYLE_ASSIGNMENT (( #125145 ) ) ;
#104081=UNCERTAINTY_MEASURE_WITH_UNIT (LENGTH_MEASURE( 1.000000000000000082E-05 ), #83564, 'distance_accuracy_value', 'NONE');
#104084=B_SPLINE_CURVE_WITH_KNOTS ( 'NONE', 3,
 ( #65500, #98098, #109678, #46627, #11768, #125574, #91512, #136419, #100240, #35003, #89356, #58932, #122686, #69054, #101652, #103094, #112535, #113964, #3729, #26252, #135724, #48020, #90807, #56052, #124838, #13193, #57470, #25513, #92191, #79245, #37113, #123451, #45880, #35736, #892, #36409 ),
 .UNSPECIFIED., .F., .F.,
 ( 4, 2, 2, 2, 2, 2, 2, 2, 2, 2, 2, 2, 2, 2, 2, 2, 2, 4 ),
 ( 0.000000000000000000, 0.002483296972363799576, 0.003724945458545699147, 0.004966593944727599151, 0.005587418187818549153, 0.006208242430909499156, 0.007449890917091394824, 0.008691539403273291359, 0.009933187889455186159, 0.01117483637563708443, 0.01241648486181898096, 0.01365813334800087923, 0.01489978183418277577, 0.01614143032036467404, 0.01738307880654656884, 0.01800390304963752144, 0.01862472729272847058, 0.01986637577891036885 ),
 .UNSPECIFIED. ) ;
#104115=CARTESIAN_POINT ( 'NONE',  ( 27.27083333333332860, 6.094999999999991758, 1.633150327867687102 ) ) ;
#104116=( LENGTH_UNIT ( ) NAMED_UNIT ( * ) SI_UNIT ( .MILLI., .METRE. ) );
#104144=VERTEX_POINT ( 'NONE', #78321 ) ;
#104148=CARTESIAN_POINT ( 'NONE',  ( 122.6835989386367771, -1.600000000000086020, -34.92499999999998295 ) ) ;
#104180=VERTEX_POINT ( 'NONE', #90633 ) ;
#104187=FILL_AREA_STYLE_COLOUR ( '', #83060 ) ;
#104219=( NAMED_UNIT ( * ) PLANE_ANGLE_UNIT ( ) SI_UNIT ( $, .RADIAN. ) );
#104223=EDGE_LOOP ( 'NONE', ( #118656, #52976, #136922, #100883 ) ) ;
#104228=AXIS2_PLACEMENT_3D ( 'NONE', #50896, #95090, #63234 ) ;
#104240=PRESENTATION_STYLE_ASSIGNMENT (( #68817 ) ) ;
#104245=CARTESIAN_POINT ( 'NONE',  ( 29.67123647476855552, 0.000000000000000000, 7.934999999999990727 ) ) ;
#104272=ORIENTED_EDGE ( 'NONE', *, *, #126834, .F. ) ;
#104291=CARTESIAN_POINT ( 'NONE',  ( 32.20790314143521726, -6.871911579029513106, -3.967499999999993587 ) ) ;
#104293=CARTESIAN_POINT ( 'NONE',  ( 10.62456980810188689, -6.871911579029512218, 3.967499999999996252 ) ) ;
#104302=EDGE_CURVE ( 'NONE', #67772, #65560, #124669, .T. ) ;
#104332=EDGE_CURVE ( 'NONE', #21837, #119012, #135331, .T. ) ;
#104335=MECHANICAL_DESIGN_GEOMETRIC_PRESENTATION_REPRESENTATION('',(#81205),#95025);
#104343=STYLED_ITEM ( 'NONE', ( #91988 ), #128132 ) ;
#104344=CARTESIAN_POINT ( 'NONE',  ( 25.39999999999999858, 0.000000000000000000, 0.000000000000000000 ) ) ;
#104354=CARTESIAN_POINT ( 'NONE',  ( 8.817069808101885897, -2.126176841940956130, 7.934999999999990727 ) ) ;
#104356=CARTESIAN_POINT ( 'NONE',  ( 21.14583333333333925, -1.633150327867709528, 6.094999999999979323 ) ) ;
#104358=( NAMED_UNIT ( * ) SI_UNIT ( $, .STERADIAN. ) SOLID_ANGLE_UNIT ( ) );
#104388=MECHANICAL_DESIGN_GEOMETRIC_PRESENTATION_REPRESENTATION('',(#32606),#58088);
#104425=VECTOR ( 'NONE', #103601, 1000.000000000000000 ) ;
#104430=CARTESIAN_POINT ( 'NONE',  ( 1.379569808101885897, 3.967499999999998916, 6.871911579029510442 ) ) ;
#104445=CARTESIAN_POINT ( 'NONE',  ( 183.3316408629057435, -52.14999999999999147, -41.64500000000001023 ) ) ;
#104466=DIRECTION ( 'NONE',  ( -1.000000000000000000, -0.000000000000000000, -0.000000000000000000 ) ) ;
#104476=DIRECTION ( 'NONE',  ( -1.000000000000000000, -0.000000000000000000, -0.000000000000000000 ) ) ;
#104493=LINE ( 'NONE', #5870, #71817 ) ;
#104494=COLOUR_RGB ( '', 0.72549020, 0.75294118, 0.79215686) ;
#104513=CARTESIAN_POINT ( 'NONE',  ( 184.1500000000000057, -14.29000000000013593, -12.70000000000045404 ) ) ;
#104550=ORIENTED_EDGE ( 'NONE', *, *, #55334, .F. ) ;
#104567=AXIS2_PLACEMENT_3D ( 'NONE', #132700, #25304, #134095 ) ;
#104608=ORIENTED_EDGE ( 'NONE', *, *, #33062, .T. ) ;
#104613=CARTESIAN_POINT ( 'NONE',  ( 10.42123647476855375, -9.717572351234235426E-16, -7.934999999999990727 ) ) ;
#104619=CARTESIAN_POINT ( 'NONE',  ( 25.37500000000000000, -6.094999999999989981, 3.732111120401553285E-16 ) ) ;
#104634=CARTESIAN_POINT ( 'NONE',  ( 61.46640106136302961, -57.15000000000008384, -34.92499999999998295 ) ) ;
#104636=CARTESIAN_POINT ( 'NONE',  ( 21.92080628287044064, 3.047499999999997655, 5.278424836066143655 ) ) ;
#104639=ORIENTED_EDGE ( 'NONE', *, *, #66597, .T. ) ;
#104643=CARTESIAN_POINT ( 'NONE',  ( 1.437069808101885782, 2.126176841940952134, -7.934999999999993392 ) ) ;
#104655=DIRECTION ( 'NONE',  ( 1.000000000000000000, 0.000000000000000000, -0.000000000000000000 ) ) ;
#104714=MECHANICAL_DESIGN_GEOMETRIC_PRESENTATION_REPRESENTATION('',(#5124),#116307);
#104738=AXIS2_PLACEMENT_3D ( 'NONE', #98824, #132207, #108243 ) ;
#104769=CARTESIAN_POINT ( 'NONE',  ( 180.8041599634935324, -49.02495722182847260, -39.69341335395904480 ) ) ;
#104783=CARTESIAN_POINT ( 'NONE',  ( 19.00413961620377279, -3.047499999999994547, 5.278424836066145431 ) ) ;
#104817=CARTESIAN_POINT ( 'NONE',  ( 0.000000000000000000, -57.15000000000009095, 34.92499999999998295 ) ) ;
#104844=DIRECTION ( 'NONE',  ( 0.000000000000000000, 0.000000000000000000, 1.000000000000000000 ) ) ;
#104860=CARTESIAN_POINT ( 'NONE',  ( 25.66666666666666785, -5.278424836066145431, -3.047499999999993658 ) ) ;
#104885=SURFACE_STYLE_USAGE ( .BOTH. , #26616 ) ;
#104909=ORIENTED_EDGE ( 'NONE', *, *, #41190, .T. ) ;
#104933=CIRCLE ( 'NONE', #65675, 1.000000000000000000 ) ;
#104958=FACE_OUTER_BOUND ( 'NONE', #23217, .T. ) ;
#104961=DIRECTION ( 'NONE',  ( 0.000000000000000000, 0.000000000000000000, 1.000000000000000000 ) ) ;
#104975=CARTESIAN_POINT ( 'NONE',  ( 0.03269009325358174928, -47.89015928896881036, 37.22465919495169118 ) ) ;
#104979=CARTESIAN_POINT ( 'NONE',  ( 31.71290314143522693, 3.967499999999992699, -6.871911579029513994 ) ) ;
#105024=CARTESIAN_POINT ( 'NONE',  ( 28.99956980810188867, -3.967499999999998028, -6.871911579029511330 ) ) ;
#105025=CARTESIAN_POINT ( 'NONE',  ( 4.645403141435220817, -2.126176841940958351, -7.934999999999988951 ) ) ;
#105052=MECHANICAL_DESIGN_GEOMETRIC_PRESENTATION_REPRESENTATION('',(#100414),#30983);
#105053=( LENGTH_UNIT ( ) NAMED_UNIT ( * ) SI_UNIT ( .MILLI., .METRE. ) );
#105059=PRESENTATION_STYLE_ASSIGNMENT (( #38386 ) ) ;
#105066=CARTESIAN_POINT ( 'NONE',  ( 7.583333333333333925, -5.278424836066144543, 3.047499999999995879 ) ) ;
#105084=CARTESIAN_POINT ( 'NONE',  ( 8.233736474768550195, 5.808823158059035485, 5.808823158059032821 ) ) ;
#105103=LINE ( 'NONE', #7182, #96447 ) ;
#105117=EDGE_CURVE ( 'NONE', #79775, #94854, #54510, .T. ) ;
#105124=COLOUR_RGB ( '', 0.40784314, 0.44705882, 0.49803922) ;
#105127=DIRECTION ( 'NONE',  ( 0.000000000000000000, 0.000000000000000000, -1.000000000000000000 ) ) ;
#105140=VERTEX_POINT ( 'NONE', #24993 ) ;
#105155=SURFACE_STYLE_FILL_AREA ( #45809 ) ;
#105159=SURFACE_STYLE_USAGE ( .BOTH. , #37788 ) ;
#105160=( NAMED_UNIT ( * ) PLANE_ANGLE_UNIT ( ) SI_UNIT ( $, .RADIAN. ) );
#105167=CARTESIAN_POINT ( 'NONE',  ( 183.8247562798467527, -48.93522302958525216, -39.28544916627431149 ) ) ;
#105175=DIRECTION ( 'NONE',  ( 0.000000000000000000, 0.000000000000000000, 1.000000000000000000 ) ) ;
#105211=FILL_AREA_STYLE ('',( #50842 ) ) ;
#105213=ORIENTED_EDGE ( 'NONE', *, *, #42385, .T. ) ;
#105259=ORIENTED_EDGE ( 'NONE', *, *, #768, .T. ) ;
#105265=LINE ( 'NONE', #128461, #4645 ) ;
#105285=PLANE ( 'NONE',  #20341 ) ;
#105320=CYLINDRICAL_SURFACE ( 'NONE', #30587, 3.000000000000002665 ) ;
#105322=CARTESIAN_POINT ( 'NONE',  ( 6.483736474768551972, -5.808823158059035485, -5.808823158059033709 ) ) ;
#105352=CARTESIAN_POINT ( 'NONE',  ( 6.249569808101886892, 3.967499999999998916, 6.871911579029510442 ) ) ;
#105372=EDGE_CURVE ( 'NONE', #8723, #43368, #77977, .T. ) ;
#105383=UNCERTAINTY_MEASURE_WITH_UNIT (LENGTH_MEASURE( 1.000000000000000082E-05 ), #89244, 'distance_accuracy_value', 'NONE');
#105422=STYLED_ITEM ( 'NONE', ( #13075 ), #6157 ) ;
#105460=( NAMED_UNIT ( * ) SI_UNIT ( $, .STERADIAN. ) SOLID_ANGLE_UNIT ( ) );
#105463=VERTEX_POINT ( 'NONE', #69632 ) ;
#105477=VECTOR ( 'NONE', #84078, 1000.000000000000000 ) ;
#105478=CARTESIAN_POINT ( 'NONE',  ( 12.73330628287043886, -6.094999999999989981, -1.633150327867689100 ) ) ;
#105504=ORIENTED_EDGE ( 'NONE', *, *, #135373, .T. ) ;
#105510=CARTESIAN_POINT ( 'NONE',  ( 27.97873647476855297, -5.808823158059033709, 5.808823158059035485 ) ) ;
#105526=( LENGTH_UNIT ( ) NAMED_UNIT ( * ) SI_UNIT ( .MILLI., .METRE. ) );
#105545=FACE_OUTER_BOUND ( 'NONE', #143127, .T. ) ;
#105555=CARTESIAN_POINT ( 'NONE',  ( 26.10416666666666430, -1.633150327867691987, -6.094999999999989093 ) ) ;
#105576=CARTESIAN_POINT ( 'NONE',  ( 1.862596602551424896, -5.584750846682028147, 2.792454972228691989 ) ) ;
#105585=FILL_AREA_STYLE_COLOUR ( '', #86793 ) ;
#105586=DIRECTION ( 'NONE',  ( -1.000000000000000000, -0.000000000000000000, -0.000000000000000000 ) ) ;
#105595=CARTESIAN_POINT ( 'NONE',  ( 52.60764783923754351, -49.05583548141699168, -39.86617647058817937 ) ) ;
#105599=VECTOR ( 'NONE', #123103, 1000.000000000000000 ) ;
#105615=FILL_AREA_STYLE_COLOUR ( '', #40843 ) ;
#105616=FILL_AREA_STYLE_COLOUR ( '', #72899 ) ;
#105631=EDGE_CURVE ( 'NONE', #672, #5240, #26843, .T. ) ;
#105652=FILL_AREA_STYLE ('',( #15760 ) ) ;
#105654=EDGE_CURVE ( 'NONE', #93928, #46809, #74614, .T. ) ;
#105656=( LENGTH_UNIT ( ) NAMED_UNIT ( * ) SI_UNIT ( .MILLI., .METRE. ) );
#105657=ORIENTED_EDGE ( 'NONE', *, *, #89884, .T. ) ;
#105671=CARTESIAN_POINT ( 'NONE',  ( 0.7079031414352193741, -6.871911579029513106, -3.967499999999993587 ) ) ;
#105681=CARTESIAN_POINT ( 'NONE',  ( 159.7320121765528711, 26.96999999999993847, 34.92499999999998295 ) ) ;
#105694=DIRECTION ( 'NONE',  ( 0.000000000000000000, 0.000000000000000000, -1.000000000000000000 ) ) ;
#105714=CARTESIAN_POINT ( 'NONE',  ( 26.22873647476855652, 5.808823158059031044, -5.808823158059038150 ) ) ;
#105715=CARTESIAN_POINT ( 'NONE',  ( 6.395403141435219929, 2.126176841940962348, 7.934999999999988951 ) ) ;
#105731=CARTESIAN_POINT ( 'NONE',  ( 24.39999999999999858, -2.600000000000012079, -20.40202195861969159 ) ) ;
#105750=CIRCLE ( 'NONE', #91800, 1.000000000000000888 ) ;
#105773=CARTESIAN_POINT ( 'NONE',  ( 12.60873647476855197, -5.808823158059033709, 5.808823158059035485 ) ) ;
#105776=ORIENTED_EDGE ( 'NONE', *, *, #111786, .T. ) ;
#105786=CARTESIAN_POINT ( 'NONE',  ( 6.270833333333333925, 6.094999999999991758, 1.633150327867686880 ) ) ;
#105806=CIRCLE ( 'NONE', #43347, 0.9999999999999997780 ) ;
#105821=LINE ( 'NONE', #117410, #133985 ) ;
#105843=MECHANICAL_DESIGN_GEOMETRIC_PRESENTATION_REPRESENTATION('',(#66572),#41094);
#105844=CARTESIAN_POINT ( 'NONE',  ( 11.29623647476855375, 7.934999999999990727, -1.457635852685135314E-15 ) ) ;
#105847=DIRECTION ( 'NONE',  ( 0.000000000000000000, -1.000000000000000000, 0.000000000000000000 ) ) ;
#105848=DIRECTION ( 'NONE',  ( 0.000000000000000000, 0.000000000000000000, -1.000000000000000000 ) ) ;
#105857=CARTESIAN_POINT ( 'NONE',  ( 183.5369301914234086, -49.19053253528003466, -40.77637019028070853 ) ) ;
#105864=MECHANICAL_DESIGN_GEOMETRIC_PRESENTATION_REPRESENTATION('',(#20183),#43400);
#105869=CARTESIAN_POINT ( 'NONE',  ( 0.3872656504351221218, -51.96230815476842224, -39.57541490114649463 ) ) ;
#105874=ORIENTED_EDGE ( 'NONE', *, *, #134827, .T. ) ;
#105898=CARTESIAN_POINT ( 'NONE',  ( 156.1499999999997783, -49.14999999999999147, -34.92499999999975557 ) ) ;
#105922=PRESENTATION_STYLE_ASSIGNMENT (( #44093 ) ) ;
#105963=VERTEX_POINT ( 'NONE', #55573 ) ;
#105966=FACE_OUTER_BOUND ( 'NONE', #86306, .T. ) ;
#105989=CIRCLE ( 'NONE', #38870, 31.93000000000001393 ) ;
#106012=CARTESIAN_POINT ( 'NONE',  ( 8.233736474768550195, 5.808823158059036373, 5.808823158059032821 ) ) ;
#106021=CARTESIAN_POINT ( 'NONE',  ( 11.27497294953710671, 4.461849672132300881, 4.461849672132299105 ) ) ;
#106046=CARTESIAN_POINT ( 'NONE',  ( 2.020403141435219485, 7.934999999999989839, -2.126176841940961904 ) ) ;
#106063=DIRECTION ( 'NONE',  ( -1.000000000000000000, 0.000000000000000000, -0.000000000000000000 ) ) ;
#106079=ORIENTED_EDGE ( 'NONE', *, *, #107947, .F. ) ;
#106094=ORIENTED_EDGE ( 'NONE', *, *, #91700, .F. ) ;
#106111=AXIS2_PLACEMENT_3D ( 'NONE', #92104, #24018, #14561 ) ;
#106174=ORIENTED_EDGE ( 'NONE', *, *, #58835, .F. ) ;
#106178=CARTESIAN_POINT ( 'NONE',  ( 11.85830628287044064, -1.633150327867689988, 6.094999999999989981 ) ) ;
#106181=ORIENTED_EDGE ( 'NONE', *, *, #26776, .T. ) ;
#106226=EDGE_CURVE ( 'NONE', #23170, #84791, #36179, .T. ) ;
#106250=CARTESIAN_POINT ( 'NONE',  ( 25.39999999999999503, 3.246059068589359775, 5.158694168414005077 ) ) ;
#106253=FILL_AREA_STYLE_COLOUR ( '', #99191 ) ;
#106257=CARTESIAN_POINT ( 'NONE',  ( 33.68750000000000711, 4.461849672132297329, -4.461849672132302658 ) ) ;
#106275=CARTESIAN_POINT ( 'NONE',  ( 12.39583333333333570, 1.633150327867697316, -6.094999999999986429 ) ) ;
#106277=CARTESIAN_POINT ( 'NONE',  ( 1.944300147912140453, -5.919729343870397287, 1.711352533870144521 ) ) ;
#106285=PRESENTATION_STYLE_ASSIGNMENT (( #138247 ) ) ;
#106290=CARTESIAN_POINT ( 'NONE',  ( 166.8575281714868481, 26.96999999999994202, -31.92499999999998295 ) ) ;
#106307=CARTESIAN_POINT ( 'NONE',  ( 24.39999999999999858, 1.399999999999986366, 20.40202195861970580 ) ) ;
#106313=ORIENTED_EDGE ( 'NONE', *, *, #99334, .T. ) ;
#106319=PRESENTATION_STYLE_ASSIGNMENT (( #4849 ) ) ;
#106320=EDGE_CURVE ( 'NONE', #105140, #68985, #68683, .T. ) ;
#106368=CARTESIAN_POINT ( 'NONE',  ( 2.999999998679837354, -47.86718710719786429, 37.19897551713999917 ) ) ;
#106371=CARTESIAN_POINT ( 'NONE',  ( 5.082903141435219041, 3.967499999999992699, -6.871911579029513994 ) ) ;
#106376=ORIENTED_EDGE ( 'NONE', *, *, #82858, .T. ) ;
#106379=( NAMED_UNIT ( * ) SI_UNIT ( $, .STERADIAN. ) SOLID_ANGLE_UNIT ( ) );
#106381=CARTESIAN_POINT ( 'NONE',  ( 181.1500000000000057, 0.000000000000000000, -31.92499999999998295 ) ) ;
#106392=AXIS2_PLACEMENT_3D ( 'NONE', #120556, #111116, #74981 ) ;
#106404=SURFACE_SIDE_STYLE ('',( #117996 ) ) ;
#106412=CARTESIAN_POINT ( 'NONE',  ( 2.041666666666666963, 3.047499999999993214, -5.278424836066146320 ) ) ;
#106413=CARTESIAN_POINT ( 'NONE',  ( 6.832903141435220817, -3.967499999999994476, 6.871911579029513106 ) ) ;
#106434=DIRECTION ( 'NONE',  ( -0.9707728879609256456, 0.000000000000000000, -0.2400000000000085398 ) ) ;
#106455=( NAMED_UNIT ( * ) SI_UNIT ( $, .STERADIAN. ) SOLID_ANGLE_UNIT ( ) );
#106465=EDGE_LOOP ( 'NONE', ( #14488, #122574, #102510, #28678 ) ) ;
#106466=DIRECTION ( 'NONE',  ( 0.000000000000000000, -1.000000000000000000, 0.000000000000000000 ) ) ;
#106475=CARTESIAN_POINT ( 'NONE',  ( 13.19206980810188412, -7.934999999999990727, -2.126176841940955242 ) ) ;
#106483=DIRECTION ( 'NONE',  ( -1.000000000000000000, -0.000000000000000000, 0.000000000000000000 ) ) ;
#106485=EDGE_LOOP ( 'NONE', ( #12754, #31446, #62619, #79599, #15481 ) ) ;
#106534=VECTOR ( 'NONE', #85959, 1000.000000000000000 ) ;
#106553=CARTESIAN_POINT ( 'NONE',  ( 13.33790314143522160, -6.871911579029513106, -3.967499999999993587 ) ) ;
#106598=VERTEX_POINT ( 'NONE', #38632 ) ;
#106636=EDGE_CURVE ( 'NONE', #81966, #66916, #1556, .T. ) ;
#106645=FILL_AREA_STYLE ('',( #28414 ) ) ;
#106678=DIRECTION ( 'NONE',  ( 0.000000000000000000, 0.000000000000000000, 1.000000000000000000 ) ) ;
#106686=CARTESIAN_POINT ( 'NONE',  ( 3.191216777807879712, -48.83231052142029682, 38.98973348322100207 ) ) ;
#106718=CARTESIAN_POINT ( 'NONE',  ( 19.29580628287044064, -5.278424836066144543, 3.047499999999995879 ) ) ;
#106732=SURFACE_SIDE_STYLE ('',( #127818 ) ) ;
#106733=CARTESIAN_POINT ( 'NONE',  ( 15.23373647476855375, 5.808823158059036373, 5.808823158059032821 ) ) ;
#106747=LINE ( 'NONE', #75585, #72525 ) ;
#106773=CARTESIAN_POINT ( 'NONE',  ( 15.87456980810188867, 6.871911579029510442, -3.967499999999998916 ) ) ;
#106782=CARTESIAN_POINT ( 'NONE',  ( 5.879139616203772789, -5.278424836066145431, -3.047499999999993658 ) ) ;
#106793=CARTESIAN_POINT ( 'NONE',  ( 24.39999999999999858, 1.194621026894847171, -17.40906030209848510 ) ) ;
#106844=CARTESIAN_POINT ( 'NONE',  ( 25.39999999999999858, 0.000000000000000000, 6.094999999999989093 ) ) ;
#106849=ORIENTED_EDGE ( 'NONE', *, *, #32387, .T. ) ;
#106868=STYLED_ITEM ( 'NONE', ( #98442 ), #61305 ) ;
#106911=VERTEX_POINT ( 'NONE', #69689 ) ;
#106914=CARTESIAN_POINT ( 'NONE',  ( 16.37913961620377279, -5.278424836066145431, -3.047499999999993658 ) ) ;
#106950=CARTESIAN_POINT ( 'NONE',  ( 33.95790314143522437, 6.871911579029515771, 3.967499999999989146 ) ) ;
#106995=DIRECTION ( 'NONE',  ( 0.000000000000000000, 0.000000000000000000, -1.000000000000000000 ) ) ;
#107025=ORIENTED_EDGE ( 'NONE', *, *, #137151, .T. ) ;
#107036=CARTESIAN_POINT ( 'NONE',  ( 184.1499999999998067, -57.14999999999999147, -34.92499999999972715 ) ) ;
#107065=AXIS2_PLACEMENT_3D ( 'NONE', #64853, #63449, #88021 ) ;
#107114=CARTESIAN_POINT ( 'NONE',  ( 8.145403141435220817, -2.126176841940958351, -7.934999999999989839 ) ) ;
#107144=CARTESIAN_POINT ( 'NONE',  ( 52.60764783923752930, -49.05583548141699879, -39.86617647058820069 ) ) ;
#107151=UNCERTAINTY_MEASURE_WITH_UNIT (LENGTH_MEASURE( 1.000000000000000082E-05 ), #51634, 'distance_accuracy_value', 'NONE');
#107161=CARTESIAN_POINT ( 'NONE',  ( 2.770833333333333925, 6.094999999999991758, 1.633150327867687102 ) ) ;
#107162=CARTESIAN_POINT ( 'NONE',  ( 6.687069808101886004, -2.126176841940956130, 7.934999999999990727 ) ) ;
#107178=EDGE_CURVE ( 'NONE', #57246, #85199, #1909, .T. ) ;
#107184=FILL_AREA_STYLE ('',( #52787 ) ) ;
#107192=CARTESIAN_POINT ( 'NONE',  ( 58.17012237851905354, -48.09441802426618295, 35.89947574910241457 ) ) ;
#107201=CARTESIAN_POINT ( 'NONE',  ( 128.4365526510869699, -51.77943056867388805, 39.18578444878806266 ) ) ;
#107220=CARTESIAN_POINT ( 'NONE',  ( 11.73373647476855197, 5.808823158059035485, 5.808823158059032821 ) ) ;
#107233=CARTESIAN_POINT ( 'NONE',  ( 18.22916666666666785, -6.094999999999989093, 1.633150327867691542 ) ) ;
#107235=EDGE_LOOP ( 'NONE', ( #86083, #48809, #113737, #74412 ) ) ;
#107291=CARTESIAN_POINT ( 'NONE',  ( 8.817069808101885897, -2.126176841940956130, 7.934999999999991616 ) ) ;
#107319=EDGE_LOOP ( 'NONE', ( #126875, #41997, #58412, #53926 ) ) ;
#107327=UNCERTAINTY_MEASURE_WITH_UNIT (LENGTH_MEASURE( 1.000000000000000082E-05 ), #65044, 'distance_accuracy_value', 'NONE');
#107333=CARTESIAN_POINT ( 'NONE',  ( 3.062499999999999556, 4.461849672132300881, 4.461849672132299105 ) ) ;
#107361=ORIENTED_EDGE ( 'NONE', *, *, #108905, .F. ) ;
#107382=( NAMED_UNIT ( * ) SI_UNIT ( $, .STERADIAN. ) SOLID_ANGLE_UNIT ( ) );
#107409=AXIS2_PLACEMENT_3D ( 'NONE', #96099, #142494, #54772 ) ;
#107412=EDGE_CURVE ( 'NONE', #34779, #42914, #130313, .T. ) ;
#107418=VECTOR ( 'NONE', #39768, 1000.000000000000000 ) ;
#107464=CARTESIAN_POINT ( 'NONE',  ( 22.23373647476855197, 5.808823158059036373, 5.808823158059032821 ) ) ;
#107469=STYLED_ITEM ( 'NONE', ( #52764 ), #89171 ) ;
#107490=CARTESIAN_POINT ( 'NONE',  ( 3.937500000000000000, -4.461849672132299105, 4.461849672132299993 ) ) ;
#107499=CARTESIAN_POINT ( 'NONE',  ( 11.49956980810188689, -3.967499999999998028, -6.871911579029511330 ) ) ;
#107505=EDGE_LOOP ( 'NONE', ( #130524, #127230, #6062, #63709 ) ) ;
#107514=CYLINDRICAL_SURFACE ( 'NONE', #88286, 1.000000000000000888 ) ;
#107543=DIRECTION ( 'NONE',  ( 0.000000000000000000, 0.000000000000000000, 1.000000000000000000 ) ) ;
#107553=( LENGTH_UNIT ( ) NAMED_UNIT ( * ) SI_UNIT ( .MILLI., .METRE. ) );
#107555=FILL_AREA_STYLE ('',( #64068 ) ) ;
#107558=CARTESIAN_POINT ( 'NONE',  ( 24.39999999999999858, -1.600000000000012301, -20.40202195861969514 ) ) ;
#107562=CARTESIAN_POINT ( 'NONE',  ( 14.43749999999999822, -4.461849672132299105, 4.461849672132299993 ) ) ;
#107567=STYLED_ITEM ( 'NONE', ( #31953 ), #104071 ) ;
#107573=SURFACE_SIDE_STYLE ('',( #71400 ) ) ;
#107580=EDGE_CURVE ( 'NONE', #67772, #55981, #76651, .T. ) ;
#107628=CARTESIAN_POINT ( 'NONE',  ( 22.06663961620377634, 1.633150327867695095, 6.094999999999988205 ) ) ;
#107632=B_SPLINE_CURVE_WITH_KNOTS ( 'NONE', 3,
 ( #73692, #139698, #17172, #128093, #28773, #71562, #95433, #4804, #61435, #6952, #5553, #40378, #51953, #117863, #38923, #127349, #84581, #38218, #115010, #105576, #81748, #106277, #93300, #128778 ),
 .UNSPECIFIED., .F., .F.,
 ( 4, 2, 2, 2, 2, 2, 2, 2, 2, 2, 2, 4 ),
 ( 0.01986637577891036885, 0.02043143082653421302, 0.02099648587415805720, 0.02212659596940574208, 0.02269165101702958626, 0.02325670606465343043, 0.02438681615990111531, 0.02495187120752495602, 0.02551692625514880020, 0.02664703635039648508, 0.02777714644564416996, 0.02890725654089185484 ),
 .UNSPECIFIED. ) ;
#107657=B_SPLINE_CURVE_WITH_KNOTS ( 'NONE', 3,
 ( #132189, #77800, #121283, #56075, #88685, #182 ),
 .UNSPECIFIED., .F., .F.,
 ( 4, 2, 4 ),
 ( 0.01602987264650632127, 0.01771478214218283678, 0.01939969163785935230 ),
 .UNSPECIFIED. ) ;
#107664=CARTESIAN_POINT ( 'NONE',  ( 30.74956980810188867, 3.967499999999998916, 6.871911579029510442 ) ) ;
#107697=( NAMED_UNIT ( * ) SI_UNIT ( $, .STERADIAN. ) SOLID_ANGLE_UNIT ( ) );
#107710=CARTESIAN_POINT ( 'NONE',  ( 29.02083333333333215, -6.094999999999989981, -1.633150327867689100 ) ) ;
#107714=EDGE_CURVE ( 'NONE', #6561, #109345, #49799, .T. ) ;
#107726=FACE_OUTER_BOUND ( 'NONE', #60236, .T. ) ;
#107729=DIRECTION ( 'NONE',  ( 1.000000000000000000, -0.000000000000000000, 0.000000000000000000 ) ) ;
#107743=EDGE_CURVE ( 'NONE', #33206, #47238, #102099, .T. ) ;
#107755=PRESENTATION_STYLE_ASSIGNMENT (( #17200 ) ) ;
#107762=COLOUR_RGB ( '', 0.08235294, 0.09019608, 0.10196078) ;
#107797=CARTESIAN_POINT ( 'NONE',  ( 152.4000000000000057, -14.29000000000013593, 12.69999999999954632 ) ) ;
#107815=EDGE_CURVE ( 'NONE', #110351, #34779, #23190, .T. ) ;
#107816=CARTESIAN_POINT ( 'NONE',  ( 5.374569808101886892, 6.871911579029510442, -3.967499999999998916 ) ) ;
#107819=DIRECTION ( 'NONE',  ( 0.000000000000000000, -1.000000000000000000, 0.000000000000000000 ) ) ;
#107839=CARTESIAN_POINT ( 'NONE',  ( 52.69985579144460530, -48.99436351328190398, -39.52330221398148069 ) ) ;
#107857=CARTESIAN_POINT ( 'NONE',  ( 8.895833333333333925, 1.633150327867687324, -6.094999999999991758 ) ) ;
#107858=CARTESIAN_POINT ( 'NONE',  ( 20.54123647476855652, 0.000000000000000000, 7.934999999999990727 ) ) ;
#107868=CARTESIAN_POINT ( 'NONE',  ( 128.5894344200537773, -52.00875322212549179, -39.86617647058817226 ) ) ;
#107873=CARTESIAN_POINT ( 'NONE',  ( 0.01254890717039356708, -50.57777258831014677, 35.91905586107260007 ) ) ;
#107877=SURFACE_STYLE_FILL_AREA ( #52102 ) ;
#107881=CARTESIAN_POINT ( 'NONE',  ( 58.16711163708901466, -46.44928942427405616, 35.85226645763361120 ) ) ;
#107889=CARTESIAN_POINT ( 'NONE',  ( 128.1966263608613588, -51.41954113333839160, 38.53170190052058075 ) ) ;
#107908=CARTESIAN_POINT ( 'NONE',  ( 20.33790314143522338, -6.871911579029513106, -3.967499999999993587 ) ) ;
#107930=SURFACE_SIDE_STYLE ('',( #8598 ) ) ;
#107932=CARTESIAN_POINT ( 'NONE',  ( 25.39999999999999147, 4.671400280653048576, -6.417465358227912198 ) ) ;
#107938=VERTEX_POINT ( 'NONE', #61588 ) ;
#107943=CARTESIAN_POINT ( 'NONE',  ( 174.7500000000000000, 7.919999999999947526, 19.12499999999998224 ) ) ;
#107947=EDGE_CURVE ( 'NONE', #65885, #62041, #17331, .T. ) ;
#107964=FACE_OUTER_BOUND ( 'NONE', #136441, .T. ) ;
#107977=CARTESIAN_POINT ( 'NONE',  ( 5.317069808101885897, -2.126176841940956130, 7.934999999999991616 ) ) ;
#107995=CARTESIAN_POINT ( 'NONE',  ( 184.1499999999998067, -50.22575108203221816, -35.38524182945423746 ) ) ;
#108018=CARTESIAN_POINT ( 'NONE',  ( 0.1600000000000025846, -3.262421210207534283, -7.241152424009429822 ) ) ;
#108021=FACE_OUTER_BOUND ( 'NONE', #138386, .T. ) ;
#108106=CARTESIAN_POINT ( 'NONE',  ( 153.4000000000000057, -16.48000000000005016, 33.92499999999998295 ) ) ;
#108123=( NAMED_UNIT ( * ) PLANE_ANGLE_UNIT ( ) SI_UNIT ( $, .RADIAN. ) );
#108147=CARTESIAN_POINT ( 'NONE',  ( 14.79623647476855375, 7.934999999999990727, -1.457635852685135314E-15 ) ) ;
#108170=CARTESIAN_POINT ( 'NONE',  ( 4.375000000000000000, -6.094999999999989981, 3.732111120401553285E-16 ) ) ;
#108179=CARTESIAN_POINT ( 'NONE',  ( 13.68706980810188334, -2.126176841940956130, 7.934999999999991616 ) ) ;
#108243=DIRECTION ( 'NONE',  ( 0.000000000000000000, 0.000000000000000000, 1.000000000000000000 ) ) ;
#108257=( NAMED_UNIT ( * ) PLANE_ANGLE_UNIT ( ) SI_UNIT ( $, .RADIAN. ) );
#108263=DIRECTION ( 'NONE',  ( 0.000000000000000000, 0.000000000000000000, 1.000000000000000000 ) ) ;
#108311=CARTESIAN_POINT ( 'NONE',  ( 23.37913961620377279, -5.278424836066145431, -3.047499999999993658 ) ) ;
#108314=ADVANCED_FACE ( 'NONE', ( #83709 ), #117685, .F. ) ;
#108317=CARTESIAN_POINT ( 'NONE',  ( 152.4000000000000057, 7.919999999999947526, -21.52770000000001005 ) ) ;
#108349=( NAMED_UNIT ( * ) PLANE_ANGLE_UNIT ( ) SI_UNIT ( $, .RADIAN. ) );
#108458=VECTOR ( 'NONE', #28344, 1000.000000000000000 ) ;
#108472=VERTEX_POINT ( 'NONE', #98124 ) ;
#108482=CARTESIAN_POINT ( 'NONE',  ( -1.850027050462894174, -4.461849672132299105, 4.461849672132299993 ) ) ;
#108485=CARTESIAN_POINT ( 'NONE',  ( 25.39999999999999858, 0.000000000000000000, 0.000000000000000000 ) ) ;
#108488=COLOUR_RGB ( '', 0.72549020, 0.75294118, 0.79215686) ;
#108513=CARTESIAN_POINT ( 'NONE',  ( 0.2704031414352193186, -7.934999999999989839, 2.126176841940957907 ) ) ;
#108544=ORIENTED_EDGE ( 'NONE', *, *, #96479, .F. ) ;
#108546=UNCERTAINTY_MEASURE_WITH_UNIT (LENGTH_MEASURE( 1.000000000000000082E-05 ), #60894, 'distance_accuracy_value', 'NONE');
#108555=CARTESIAN_POINT ( 'NONE',  ( 0.4375000000000001665, -4.461849672132299105, 4.461849672132299993 ) ) ;
#108556=CARTESIAN_POINT ( 'NONE',  ( 14.56206980810188512, -7.934999999999990727, -2.126176841940955242 ) ) ;
#108567=CARTESIAN_POINT ( 'NONE',  ( 128.6786164994711612, -49.14501756083436135, -40.36361034346619903 ) ) ;
#108571=MECHANICAL_DESIGN_GEOMETRIC_PRESENTATION_REPRESENTATION('',(#113259),#78513);
#108574=AXIS2_PLACEMENT_3D ( 'NONE', #15213, #48589, #94221 ) ;
#108576=SURFACE_STYLE_USAGE ( .BOTH. , #139854 ) ;
#108592=CARTESIAN_POINT ( 'NONE',  ( 128.6577301979972390, -49.12413125935271552, 39.93743342457242562 ) ) ;
#108616=EDGE_CURVE ( 'NONE', #97401, #96891, #77149, .T. ) ;
#108618=CARTESIAN_POINT ( 'NONE',  ( 15.81706980810188767, -2.126176841940956130, 7.934999999999990727 ) ) ;
#108641=( NAMED_UNIT ( * ) PLANE_ANGLE_UNIT ( ) SI_UNIT ( $, .RADIAN. ) );
#108685=CARTESIAN_POINT ( 'NONE',  ( 7.212903141435218934, 3.967499999999992699, -6.871911579029513994 ) ) ;
#108729=CARTESIAN_POINT ( 'NONE',  ( 0.1600000000000028066, -2.637033663574361420, -7.491577539992840151 ) ) ;
#108739=ORIENTED_EDGE ( 'NONE', *, *, #6994, .F. ) ;
#108752=( LENGTH_UNIT ( ) NAMED_UNIT ( * ) SI_UNIT ( .MILLI., .METRE. ) );
#108784=STYLED_ITEM ( 'NONE', ( #39208 ), #63723 ) ;
#108814=AXIS2_PLACEMENT_3D ( 'NONE', #19971, #64936, #110536 ) ;
#108824=ORIENTED_EDGE ( 'NONE', *, *, #58835, .T. ) ;
#108837=ORIENTED_EDGE ( 'NONE', *, *, #78263, .F. ) ;
#108838=( LENGTH_UNIT ( ) NAMED_UNIT ( * ) SI_UNIT ( .MILLI., .METRE. ) );
#108845=FILL_AREA_STYLE_COLOUR ( '', #46052 ) ;
#108852=CARTESIAN_POINT ( 'NONE',  ( 19.44163961620376924, -6.094999999999989093, 1.633150327867691542 ) ) ;
#108861=CARTESIAN_POINT ( 'NONE',  ( 24.39999999999999858, -7.600000000000055600, -33.92499999999998295 ) ) ;
#108862=CARTESIAN_POINT ( 'NONE',  ( 14.35873647476855197, 5.808823158059031044, -5.808823158059038150 ) ) ;
#108905=EDGE_CURVE ( 'NONE', #94854, #3140, #126523, .T. ) ;
#108912=DIRECTION ( 'NONE',  ( 0.000000000000000000, 0.7453559924999308972, -0.6666666666666655194 ) ) ;
#108934=DIRECTION ( 'NONE',  ( -0.000000000000000000, -5.075120898959323014E-15, -1.000000000000000000 ) ) ;
#108985=( NAMED_UNIT ( * ) PLANE_ANGLE_UNIT ( ) SI_UNIT ( $, .RADIAN. ) );
#108989=( LENGTH_UNIT ( ) NAMED_UNIT ( * ) SI_UNIT ( .MILLI., .METRE. ) );
#109002=CONICAL_SURFACE ( 'NONE', #46577, 2.552699999999928693, 1.029744258676634772 ) ;
#109040=CARTESIAN_POINT ( 'NONE',  ( 2.999999999999999112, -43.14999999999997726, 34.92499999999998295 ) ) ;
#109050=CARTESIAN_POINT ( 'NONE',  ( 22.50413961620377634, -3.047499999999994547, 5.278424836066145431 ) ) ;
#109099=PRESENTATION_STYLE_ASSIGNMENT (( #3016 ) ) ;
#109143=CARTESIAN_POINT ( 'NONE',  ( 28.29166666666667140, -3.047499999999994547, 5.278424836066145431 ) ) ;
#109164=ORIENTED_EDGE ( 'NONE', *, *, #103747, .F. ) ;
#109165=FILL_AREA_STYLE ('',( #98990 ) ) ;
#109171=ORIENTED_EDGE ( 'NONE', *, *, #60269, .F. ) ;
#109197=FILL_AREA_STYLE ('',( #30952 ) ) ;
#109206=CARTESIAN_POINT ( 'NONE',  ( 180.8090197240729537, -49.02095135882289156, 39.67421197282972400 ) ) ;
#109244=CIRCLE ( 'NONE', #123140, 3.000000000000001332 ) ;
#109266=CARTESIAN_POINT ( 'NONE',  ( 16.16623647476855652, 7.934999999999990727, -1.457635852685135314E-15 ) ) ;
#109311=CARTESIAN_POINT ( 'NONE',  ( 2.187499999999999556, 4.461849672132297329, -4.461849672132302658 ) ) ;
#109312=CARTESIAN_POINT ( 'NONE',  ( 19.66623647476855297, 7.934999999999990727, -1.457635852685135314E-15 ) ) ;
#109316=FACE_OUTER_BOUND ( 'NONE', #82310, .T. ) ;
#109335=DIRECTION ( 'NONE',  ( 0.000000000000000000, 0.000000000000000000, 1.000000000000000000 ) ) ;
#109336=CARTESIAN_POINT ( 'NONE',  ( 0.000000000000000000, -49.85820393249939286, 34.92500000000001847 ) ) ;
#109345=VERTEX_POINT ( 'NONE', #40521 ) ;
#109354=CARTESIAN_POINT ( 'NONE',  ( 183.9346320274810012, -51.67626207039724306, 38.40320453011148771 ) ) ;
#109368=CARTESIAN_POINT ( 'NONE',  ( 18.29623647476855197, 7.934999999999990727, -1.457635852685135314E-15 ) ) ;
#109370=CARTESIAN_POINT ( 'NONE',  ( 166.8575281714868765, 26.96999999999993847, 32.10205088422555519 ) ) ;
#109380=CIRCLE ( 'NONE', #102477, 6.000000000000001776 ) ;
#109390=AXIS2_PLACEMENT_3D ( 'NONE', #104344, #122729, #121298 ) ;
#109437=CARTESIAN_POINT ( 'NONE',  ( 23.10873647476855552, -5.808823158059033709, 5.808823158059035485 ) ) ;
#109445=EDGE_LOOP ( 'NONE', ( #43331, #98244, #6288, #85709 ) ) ;
#109463=AXIS2_PLACEMENT_3D ( 'NONE', #1265, #33938, #78154 ) ;
#109467=ADVANCED_FACE ( 'NONE', ( #129639 ), #48309, .T. ) ;
#109482=CARTESIAN_POINT ( 'NONE',  ( 0.1600000000000006972, -7.413834132789976827, 2.908321245901498209 ) ) ;
#109490=DIRECTION ( 'NONE',  ( 0.000000000000000000, -1.000000000000000000, 0.000000000000000000 ) ) ;
#109519=ORIENTED_EDGE ( 'NONE', *, *, #52687, .F. ) ;
#109527=CARTESIAN_POINT ( 'NONE',  ( 156.1500000000000057, -49.14999999999999147, 49.92499999999997584 ) ) ;
#109532=ORIENTED_EDGE ( 'NONE', *, *, #105117, .F. ) ;
#109559=CARTESIAN_POINT ( 'NONE',  ( 25.39999999999999858, 1.399999999999986366, 20.40202195861970580 ) ) ;
#109566=CARTESIAN_POINT ( 'NONE',  ( 3.000000000000000888, -47.87246431468552998, 37.20487561447691149 ) ) ;
#109569=CARTESIAN_POINT ( 'NONE',  ( 25.39999999999999503, 3.246059068589359775, 5.158694168414005077 ) ) ;
#109578=PRESENTATION_STYLE_ASSIGNMENT (( #22538 ) ) ;
#109604=CARTESIAN_POINT ( 'NONE',  ( 21.50456980810188412, 6.871911579029510442, -3.967499999999998916 ) ) ;
#109659=STYLED_ITEM ( 'NONE', ( #27598 ), #87420 ) ;
#109665=ORIENTED_EDGE ( 'NONE', *, *, #8540, .F. ) ;
#109678=CARTESIAN_POINT ( 'NONE',  ( 0.2519841907209453002, 4.694990751126481676, -6.337663282209763160 ) ) ;
#109684=EDGE_CURVE ( 'NONE', #143089, #121198, #20136, .T. ) ;
#109723=PRESENTATION_STYLE_ASSIGNMENT (( #140909 ) ) ;
#109767=FACE_OUTER_BOUND ( 'NONE', #121842, .T. ) ;
#109770=SURFACE_SIDE_STYLE ('',( #78581 ) ) ;
#109778=MECHANICAL_DESIGN_GEOMETRIC_PRESENTATION_REPRESENTATION('',(#135371),#139921);
#109781=CARTESIAN_POINT ( 'NONE',  ( 26.00413961620377279, -3.047499999999994547, 5.278424836066145431 ) ) ;
#109849=UNCERTAINTY_MEASURE_WITH_UNIT (LENGTH_MEASURE( 1.000000000000000082E-05 ), #121620, 'distance_accuracy_value', 'NONE');
#109851=CARTESIAN_POINT ( 'NONE',  ( 56.90810577924028024, -46.18886352141520035, 34.92499999999998295 ) ) ;
#109900=DIRECTION ( 'NONE',  ( 0.000000000000000000, 0.000000000000000000, 1.000000000000000000 ) ) ;
#109912=( NAMED_UNIT ( * ) SI_UNIT ( $, .STERADIAN. ) SOLID_ANGLE_UNIT ( ) );
#109922=CARTESIAN_POINT ( 'NONE',  ( 183.5369301914312530, -49.19053253528764458, 40.77637019028212251 ) ) ;
#109946=CARTESIAN_POINT ( 'NONE',  ( 1.066639616203771901, 1.633150327867695095, 6.094999999999988205 ) ) ;
#109958=( NAMED_UNIT ( * ) SI_UNIT ( $, .STERADIAN. ) SOLID_ANGLE_UNIT ( ) );
#109969=ORIENTED_EDGE ( 'NONE', *, *, #131364, .T. ) ;
#109973=CARTESIAN_POINT ( 'NONE',  ( 13.68706980810188334, -2.126176841940956130, 7.934999999999991616 ) ) ;
#109983=SURFACE_STYLE_USAGE ( .BOTH. , #33875 ) ;
#110012=FILL_AREA_STYLE ('',( #79600 ) ) ;
#110015=CARTESIAN_POINT ( 'NONE',  ( 17.64583333333333215, -1.633150327867689988, 6.094999999999989981 ) ) ;
#110016=CARTESIAN_POINT ( 'NONE',  ( 16.02040314143522082, 7.934999999999988951, -2.126176841940961904 ) ) ;
#110037=FACE_OUTER_BOUND ( 'NONE', #104223, .T. ) ;
#110048=CARTESIAN_POINT ( 'NONE',  ( 125.0591050317584632, -46.71325913968133392, 35.40428284070863896 ) ) ;
#110053=( GEOMETRIC_REPRESENTATION_CONTEXT ( 3 ) GLOBAL_UNCERTAINTY_ASSIGNED_CONTEXT ( ( #69219 ) ) GLOBAL_UNIT_ASSIGNED_CONTEXT ( ( #31054, #20854, #31751 ) ) REPRESENTATION_CONTEXT ( 'NONE', 'WORKASPACE' ) );
#110065=CARTESIAN_POINT ( 'NONE',  ( 14.50456980810188767, 6.871911579029510442, -3.967499999999998916 ) ) ;
#110087=CARTESIAN_POINT ( 'NONE',  ( 25.39999999999999858, -5.520864266206504263E-14, 0.000000000000000000 ) ) ;
#110125=CARTESIAN_POINT ( 'NONE',  ( 13.89997294953710494, 4.461849672132297329, -4.461849672132302658 ) ) ;
#110133=CARTESIAN_POINT ( 'NONE',  ( 16.83790314143521982, -6.871911579029513106, -3.967499999999993587 ) ) ;
#110168=UNCERTAINTY_MEASURE_WITH_UNIT (LENGTH_MEASURE( 1.000000000000000082E-05 ), #92059, 'distance_accuracy_value', 'NONE');
#110175=MECHANICAL_DESIGN_GEOMETRIC_PRESENTATION_REPRESENTATION('',(#142600),#24508);
#110186=EDGE_CURVE ( 'NONE', #45858, #111873, #98888, .T. ) ;
#110207=CARTESIAN_POINT ( 'NONE',  ( 152.8142135623730837, 26.96999999999993847, 34.92499999999998295 ) ) ;
#110228=EDGE_CURVE ( 'NONE', #11327, #77069, #105806, .T. ) ;
#110248=DIRECTION ( 'NONE',  ( 0.000000000000000000, 0.000000000000000000, 1.000000000000000000 ) ) ;
#110255=DIRECTION ( 'NONE',  ( -1.000000000000000000, -0.000000000000000000, -0.000000000000000000 ) ) ;
#110297=CARTESIAN_POINT ( 'NONE',  ( 24.42123647476855552, -9.717572351234235426E-16, -7.934999999999990727 ) ) ;
#110303=EDGE_CURVE ( 'NONE', #48102, #98765, #101496, .T. ) ;
#110351=VERTEX_POINT ( 'NONE', #59461 ) ;
#110364=CARTESIAN_POINT ( 'NONE',  ( 0.000000000000000000, -1.600000000000013634, 20.40202195861969159 ) ) ;
#110389=SURFACE_SIDE_STYLE ('',( #32887 ) ) ;
#110470=CARTESIAN_POINT ( 'NONE',  ( 21.33747294953710849, 6.094999999999989981, -1.119633336120465690E-15 ) ) ;
#110487=EDGE_CURVE ( 'NONE', #121754, #112625, #22452, .T. ) ;
#110501=PRESENTATION_STYLE_ASSIGNMENT (( #66336 ) ) ;
#110504=EDGE_LOOP ( 'NONE', ( #110686, #124564, #15193, #17880 ) ) ;
#110526=CARTESIAN_POINT ( 'NONE',  ( 128.0531643868628464, -51.20434817233914515, 36.87500513592859619 ) ) ;
#110536=DIRECTION ( 'NONE',  ( 0.000000000000000000, 0.000000000000000000, -1.000000000000000000 ) ) ;
#110559=CIRCLE ( 'NONE', #24893, 6.000000000000000000 ) ;
#110561=FILL_AREA_STYLE_COLOUR ( '', #37428 ) ;
#110562=AXIS2_PLACEMENT_3D ( 'NONE', #114192, #89583, #101892 ) ;
#110602=SURFACE_STYLE_FILL_AREA ( #66433 ) ;
#110634=CARTESIAN_POINT ( 'NONE',  ( -1.412527050462894396, -6.094999999999989981, 3.732111120401553285E-16 ) ) ;
#110660=CARTESIAN_POINT ( 'NONE',  ( 15.87456980810188867, 6.871911579029510442, -3.967499999999998916 ) ) ;
#110669=CYLINDRICAL_SURFACE ( 'NONE', #129752, 3.999999999999996447 ) ;
#110686=ORIENTED_EDGE ( 'NONE', *, *, #62327, .F. ) ;
#110687=EDGE_CURVE ( 'NONE', #131877, #17685, #136098, .T. ) ;
#110700=FILL_AREA_STYLE ('',( #98436 ) ) ;
#110705=CARTESIAN_POINT ( 'NONE',  ( 18.08333333333333215, -5.278424836066144543, 3.047499999999995879 ) ) ;
#110706=CARTESIAN_POINT ( 'NONE',  ( 17.47873647476855652, -5.808823158059033709, 5.808823158059035485 ) ) ;
#110729=( NAMED_UNIT ( * ) SI_UNIT ( $, .STERADIAN. ) SOLID_ANGLE_UNIT ( ) );
#110730=EDGE_CURVE ( 'NONE', #65560, #85199, #12172, .T. ) ;
#110755=VECTOR ( 'NONE', #47107, 1000.000000000000000 ) ;
#110770=DIRECTION ( 'NONE',  ( 1.000000000000000000, -0.000000000000000000, 0.000000000000000000 ) ) ;
#110775=DIRECTION ( 'NONE',  ( -0.000000000000000000, -5.075120898959323014E-15, -1.000000000000000000 ) ) ;
#110793=LINE ( 'NONE', #23066, #64248 ) ;
#110818=DIRECTION ( 'NONE',  ( -0.5150380749100710309, 1.049727191138606123E-16, -0.8571673007021021196 ) ) ;
#110829=CARTESIAN_POINT ( 'NONE',  ( 17.42123647476855908, -9.717572351234235426E-16, -7.934999999999990727 ) ) ;
#110840=CARTESIAN_POINT ( 'NONE',  ( 156.1499999999997783, -57.14999999999999147, -34.92499999999975557 ) ) ;
#110849=LINE ( 'NONE', #55822, #44335 ) ;
#110853=MECHANICAL_DESIGN_GEOMETRIC_PRESENTATION_REPRESENTATION('',(#92345),#85414);
#110855=ORIENTED_EDGE ( 'NONE', *, *, #34650, .T. ) ;
#110878=CARTESIAN_POINT ( 'NONE',  ( 18.20790314143522082, -6.871911579029513106, -3.967499999999993587 ) ) ;
#110882=CIRCLE ( 'NONE', #48406, 1.000000000000000000 ) ;
#110905=( NAMED_UNIT ( * ) PLANE_ANGLE_UNIT ( ) SI_UNIT ( $, .RADIAN. ) );
#110919=COLOUR_RGB ( '', 0.09019608, 0.27058824, 0.51372549) ;
#110947=FILL_AREA_STYLE ('',( #34874 ) ) ;
#110953=FACE_OUTER_BOUND ( 'NONE', #137000, .T. ) ;
#110954=MECHANICAL_DESIGN_GEOMETRIC_PRESENTATION_REPRESENTATION('',(#32250),#94719);
#110959=AXIS2_PLACEMENT_3D ( 'NONE', #17890, #86046, #41827 ) ;
#110997=CARTESIAN_POINT ( 'NONE',  ( 131.8806778009765708, -52.14999999999999147, 40.92499999999998295 ) ) ;
#111011=CARTESIAN_POINT ( 'NONE',  ( 31.85873647476855552, 5.808823158059031044, -5.808823158059038150 ) ) ;
#111116=DIRECTION ( 'NONE',  ( 0.000000000000000000, -1.000000000000000000, 0.000000000000000000 ) ) ;
#111136=CIRCLE ( 'NONE', #74121, 31.92999999999999972 ) ;
#111187=CARTESIAN_POINT ( 'NONE',  ( 4.150403141435219823, 7.934999999999989839, -2.126176841940961904 ) ) ;
#111200=AXIS2_PLACEMENT_3D ( 'NONE', #65910, #11455, #52828 ) ;
#111207=SURFACE_STYLE_USAGE ( .BOTH. , #12620 ) ;
#111210=AXIS2_PLACEMENT_3D ( 'NONE', #64728, #74183, #108912 ) ;
#111230=CARTESIAN_POINT ( 'NONE',  ( 55.32830738432641482, -52.14999999996970814, 41.05175048930647819 ) ) ;
#111233=AXIS2_PLACEMENT_3D ( 'NONE', #68195, #25338, #112369 ) ;
#111240=FILL_AREA_STYLE ('',( #11930 ) ) ;
#111249=DIRECTION ( 'NONE',  ( -0.000000000000000000, 0.000000000000000000, 1.000000000000000000 ) ) ;
#111257=UNCERTAINTY_MEASURE_WITH_UNIT (LENGTH_MEASURE( 1.000000000000000082E-05 ), #93309, 'distance_accuracy_value', 'NONE');
#111274=AXIS2_PLACEMENT_3D ( 'NONE', #82489, #48420, #81801 ) ;
#111276=AXIS2_PLACEMENT_3D ( 'NONE', #98834, #53189, #64805 ) ;
#111296=FACE_OUTER_BOUND ( 'NONE', #92670, .T. ) ;
#111305=ADVANCED_FACE ( 'NONE', ( #94546 ), #114856, .T. ) ;
#111313=CIRCLE ( 'NONE', #111200, 1.000000000000000888 ) ;
#111318=VECTOR ( 'NONE', #44455, 1000.000000000000000 ) ;
#111335=B_SPLINE_CURVE_WITH_KNOTS ( 'NONE', 3,
 ( #38107, #28662, #126506, #27198, #16301, #30047, #17730, #51836, #104769, #39539, #74301, #83769 ),
 .UNSPECIFIED., .F., .F.,
 ( 4, 2, 2, 2, 2, 4 ),
 ( 0.000000000000000000, 0.001125297245559203976, 0.002250594491118407953, 0.002813243113898006905, 0.003375891736677605857, 0.004501188982236803762 ),
 .UNSPECIFIED. ) ;
#111340=CARTESIAN_POINT ( 'NONE',  ( 4.129139616203772789, 5.278424836066147208, 3.047499999999990550 ) ) ;
#111349=VECTOR ( 'NONE', #49914, 1000.000000000000000 ) ;
#111363=CARTESIAN_POINT ( 'NONE',  ( 10.69163961620377279, 6.094999999999988205, -1.633150327867694651 ) ) ;
#111395=CARTESIAN_POINT ( 'NONE',  ( 11.64540314143521904, -2.126176841940958351, -7.934999999999989839 ) ) ;
#111437=UNCERTAINTY_MEASURE_WITH_UNIT (LENGTH_MEASURE( 1.000000000000000082E-05 ), #91839, 'distance_accuracy_value', 'NONE');
#111442=MECHANICAL_DESIGN_GEOMETRIC_PRESENTATION_REPRESENTATION('',(#11873),#74429);
#111447=CARTESIAN_POINT ( 'NONE',  ( 11.37500000000000178, -6.094999999999989981, 3.732111120401553285E-16 ) ) ;
#111467=DIRECTION ( 'NONE',  ( -0.000000000000000000, 1.000000000000000000, 0.000000000000000000 ) ) ;
#111468=CYLINDRICAL_SURFACE ( 'NONE', #132292, 2.999999999999999112 ) ;
#111503=COLOUR_RGB ( '', 0.08235294, 0.09019608, 0.10196078) ;
#111556=EDGE_CURVE ( 'NONE', #34663, #140587, #52119, .T. ) ;
#111576=MECHANICAL_DESIGN_GEOMETRIC_PRESENTATION_REPRESENTATION('',(#97709),#49106);
#111581=CARTESIAN_POINT ( 'NONE',  ( 19.17123647476855197, 0.000000000000000000, 7.934999999999990727 ) ) ;
#111601=( GEOMETRIC_REPRESENTATION_CONTEXT ( 3 ) GLOBAL_UNCERTAINTY_ASSIGNED_CONTEXT ( ( #91125 ) ) GLOBAL_UNIT_ASSIGNED_CONTEXT ( ( #138315, #104219, #139032 ) ) REPRESENTATION_CONTEXT ( 'NONE', 'WORKASPACE' ) );
#111614=ORIENTED_EDGE ( 'NONE', *, *, #27897, .F. ) ;
#111624=UNCERTAINTY_MEASURE_WITH_UNIT (LENGTH_MEASURE( 1.000000000000000082E-05 ), #118874, 'distance_accuracy_value', 'NONE');
#111634=CARTESIAN_POINT ( 'NONE',  ( 24.33290314143522437, -3.967499999999994476, 6.871911579029513106 ) ) ;
#111670=ORIENTED_EDGE ( 'NONE', *, *, #45968, .T. ) ;
#111671=ORIENTED_EDGE ( 'NONE', *, *, #5030, .F. ) ;
#111690=ORIENTED_EDGE ( 'NONE', *, *, #137756, .F. ) ;
#111692=SURFACE_SIDE_STYLE ('',( #23970 ) ) ;
#111710=AXIS2_PLACEMENT_3D ( 'NONE', #130006, #29959, #63361 ) ;
#111723=CARTESIAN_POINT ( 'NONE',  ( 24.83747294953710849, 6.094999999999989981, -1.119633336120465690E-15 ) ) ;
#111749=( GEOMETRIC_REPRESENTATION_CONTEXT ( 3 ) GLOBAL_UNCERTAINTY_ASSIGNED_CONTEXT ( ( #7090 ) ) GLOBAL_UNIT_ASSIGNED_CONTEXT ( ( #95434, #29457, #387 ) ) REPRESENTATION_CONTEXT ( 'NONE', 'WORKASPACE' ) );
#111761=CARTESIAN_POINT ( 'NONE',  ( 23.25456980810188767, -6.871911579029512218, 3.967499999999996252 ) ) ;
#111780=EDGE_CURVE ( 'NONE', #119924, #66688, #27409, .T. ) ;
#111786=EDGE_CURVE ( 'NONE', #69422, #71281, #66977, .T. ) ;
#111787=EDGE_LOOP ( 'NONE', ( #113511, #50500 ) ) ;
#111814=DIRECTION ( 'NONE',  ( -0.000000000000000000, 0.000000000000000000, 1.000000000000000000 ) ) ;
#111820=CARTESIAN_POINT ( 'NONE',  ( 1.598550070791607602, -0.6056895305754137482, -6.475271963048705892 ) ) ;
#111867=DIRECTION ( 'NONE',  ( -1.000000000000000000, -0.000000000000000000, 0.000000000000000000 ) ) ;
#111873=VERTEX_POINT ( 'NONE', #81780 ) ;
#111888=EDGE_CURVE ( 'NONE', #81966, #14111, #112936, .T. ) ;
#111891=ADVANCED_FACE ( 'NONE', ( #125249 ), #70208, .F. ) ;
#111895=ADVANCED_FACE ( 'NONE', ( #114368 ), #15039, .T. ) ;
#111908=VERTEX_POINT ( 'NONE', #40402 ) ;
#111916=EDGE_CURVE ( 'NONE', #62052, #21546, #48103, .T. ) ;
#111943=CARTESIAN_POINT ( 'NONE',  ( 29.94163961620377279, -6.094999999999989093, 1.633150327867691765 ) ) ;
#111951=ORIENTED_EDGE ( 'NONE', *, *, #27028, .F. ) ;
#111952=SURFACE_STYLE_FILL_AREA ( #57583 ) ;
#111991=SURFACE_STYLE_USAGE ( .BOTH. , #67800 ) ;
#111994=SURFACE_STYLE_USAGE ( .BOTH. , #67804 ) ;
#112004=( NAMED_UNIT ( * ) PLANE_ANGLE_UNIT ( ) SI_UNIT ( $, .RADIAN. ) );
#112012=CARTESIAN_POINT ( 'NONE',  ( 2.999999999999999112, -43.14999999999999147, 34.92499999999998295 ) ) ;
#112055=VERTEX_POINT ( 'NONE', #131681 ) ;
#112081=ADVANCED_FACE ( 'NONE', ( #96856 ), #66620, .T. ) ;
#112085=CONICAL_SURFACE ( 'NONE', #49605, 8.094999999999991758, 0.7853981633974466137 ) ;
#112091=ORIENTED_EDGE ( 'NONE', *, *, #78375, .T. ) ;
#112096=( NAMED_UNIT ( * ) PLANE_ANGLE_UNIT ( ) SI_UNIT ( $, .RADIAN. ) );
#112114=CARTESIAN_POINT ( 'NONE',  ( 10.98330628287044064, 6.094999999999991758, 1.633150327867687102 ) ) ;
#112120=DIRECTION ( 'NONE',  ( 0.000000000000000000, 2.921639538487157626E-15, -1.000000000000000000 ) ) ;
#112142=AXIS2_PLACEMENT_3D ( 'NONE', #133422, #87761, #725 ) ;
#112143=CARTESIAN_POINT ( 'NONE',  ( 20.39540314143521726, 2.126176841940962348, 7.934999999999989839 ) ) ;
#112144=LINE ( 'NONE', #22935, #16162 ) ;
#112159=CARTESIAN_POINT ( 'NONE',  ( 128.5894344200537489, -49.14999999999999147, 39.86617647058822911 ) ) ;
#112167=VERTEX_POINT ( 'NONE', #56996 ) ;
#112168=CARTESIAN_POINT ( 'NONE',  ( 16.96247294953710849, -7.464222240803106570E-16, -6.094999999999989981 ) ) ;
#112173=PRESENTATION_STYLE_ASSIGNMENT (( #1913 ) ) ;
#112183=( NAMED_UNIT ( * ) PLANE_ANGLE_UNIT ( ) SI_UNIT ( $, .RADIAN. ) );
#112185=DIRECTION ( 'NONE',  ( 0.000000000000000000, -1.000000000000000000, 0.000000000000000000 ) ) ;
#112190=CARTESIAN_POINT ( 'NONE',  ( 10.20833333333333570, 3.047499999999997655, 5.278424836066143655 ) ) ;
#112202=CARTESIAN_POINT ( 'NONE',  ( 128.0580420323230157, -46.73296206246060791, -36.09967824800569502 ) ) ;
#112203=ORIENTED_EDGE ( 'NONE', *, *, #2753, .F. ) ;
#112239=PRESENTATION_STYLE_ASSIGNMENT (( #103467 ) ) ;
#112240=CARTESIAN_POINT ( 'NONE',  ( 22.52540314143522338, 2.126176841940962348, 7.934999999999988951 ) ) ;
#112312=CARTESIAN_POINT ( 'NONE',  ( 17.12956980810188767, -3.967499999999998028, -6.871911579029511330 ) ) ;
#112325=SURFACE_STYLE_FILL_AREA ( #679 ) ;
#112329=FACE_OUTER_BOUND ( 'NONE', #42015, .T. ) ;
#112332=CARTESIAN_POINT ( 'NONE',  ( 60.59549430335705011, -44.02090675800599939, -34.92500000000512728 ) ) ;
#112339=FACE_OUTER_BOUND ( 'NONE', #61528, .T. ) ;
#112352=CARTESIAN_POINT ( 'NONE',  ( 18.93706980810188867, 2.126176841940952134, -7.934999999999993392 ) ) ;
#112369=DIRECTION ( 'NONE',  ( 0.000000000000000000, 0.000000000000000000, 1.000000000000000000 ) ) ;
#112388=ORIENTED_EDGE ( 'NONE', *, *, #86910, .T. ) ;
#112406=APPLICATION_CONTEXT ( 'automotive_design' ) ;
#112407=CARTESIAN_POINT ( 'NONE',  ( 2.692069808101885897, -7.934999999999990727, -2.126176841940955242 ) ) ;
#112414=ORIENTED_EDGE ( 'NONE', *, *, #68907, .T. ) ;
#112415=ORIENTED_EDGE ( 'NONE', *, *, #15645, .F. ) ;
#112419=FACE_OUTER_BOUND ( 'NONE', #60261, .T. ) ;
#112421=ORIENTED_EDGE ( 'NONE', *, *, #34197, .F. ) ;
#112423=SURFACE_SIDE_STYLE ('',( #22520 ) ) ;
#112442=EDGE_LOOP ( 'NONE', ( #49548, #73176, #142588, #85052 ) ) ;
#112443=EDGE_CURVE ( 'NONE', #67143, #89687, #71380, .T. ) ;
#112471=CARTESIAN_POINT ( 'NONE',  ( 28.94206980810188767, 7.934999999999993392, 2.126176841940951689 ) ) ;
#112477=DIRECTION ( 'NONE',  ( 0.000000000000000000, 0.9976538855070752332, -0.06845965770171351383 ) ) ;
#112492=ORIENTED_EDGE ( 'NONE', *, *, #91940, .F. ) ;
#112535=CARTESIAN_POINT ( 'NONE',  ( 0.7137474236366083691, 7.354941029308180056, 0.7481386797838406322 ) ) ;
#112551=DIRECTION ( 'NONE',  ( 0.000000000000000000, 0.000000000000000000, 1.000000000000000000 ) ) ;
#112563=CARTESIAN_POINT ( 'NONE',  ( 152.8142135623730837, 26.96999999999993847, -34.92499999999998295 ) ) ;
#112591=EDGE_CURVE ( 'NONE', #131877, #37393, #45835, .T. ) ;
#112625=VERTEX_POINT ( 'NONE', #103828 ) ;
#112629=SURFACE_STYLE_USAGE ( .BOTH. , #109770 ) ;
#112639=CARTESIAN_POINT ( 'NONE',  ( 32.71247294953710849, 0.000000000000000000, 6.094999999999989981 ) ) ;
#112655=( GEOMETRIC_REPRESENTATION_CONTEXT ( 3 ) GLOBAL_UNCERTAINTY_ASSIGNED_CONTEXT ( ( #46407 ) ) GLOBAL_UNIT_ASSIGNED_CONTEXT ( ( #4278, #48575, #104358 ) ) REPRESENTATION_CONTEXT ( 'NONE', 'WORKASPACE' ) );
#112657=FACE_OUTER_BOUND ( 'NONE', #20224, .T. ) ;
#112694=SURFACE_SIDE_STYLE ('',( #133057 ) ) ;
#112697=EDGE_CURVE ( 'NONE', #70428, #96891, #114716, .T. ) ;
#112719=EDGE_CURVE ( 'NONE', #48370, #42602, #87615, .T. ) ;
#112763=CARTESIAN_POINT ( 'NONE',  ( 2.999999999999999112, -1.600000000000060929, 28.92500000000001847 ) ) ;
#112800=CARTESIAN_POINT ( 'NONE',  ( 6.024972949537104938, -4.461849672132299993, -4.461849672132299105 ) ) ;
#112830=CARTESIAN_POINT ( 'NONE',  ( 19.37456980810188867, 6.871911579029510442, -3.967499999999998916 ) ) ;
#112838=( LENGTH_UNIT ( ) NAMED_UNIT ( * ) SI_UNIT ( .MILLI., .METRE. ) );
#112844=LINE ( 'NONE', #25111, #94660 ) ;
#112846=DIRECTION ( 'NONE',  ( -1.000000000000000000, -0.000000000000000000, -0.000000000000000000 ) ) ;
#112868=( BOUNDED_SURFACE ( )  B_SPLINE_SURFACE ( 3, 2, ( 
 ( #93950, #128040, #5493 ),
 ( #75093, #6188, #96080 ),
 ( #7639, #129428, #138907 ),
 ( #96762, #119259, #83086 ),
 ( #39599, #60662, #62778 ),
 ( #49771, #41720, #117120 ),
 ( #17113, #29403, #138183 ),
 ( #117814, #17794, #38866 ),
 ( #30116, #62068, #127288 ),
 ( #27987, #72257, #51900 ),
 ( #74364, #118552, #51177 ),
 ( #116427, #61381, #28720 ) ),
 .UNSPECIFIED., .F., .F., .F. ) 
 B_SPLINE_SURFACE_WITH_KNOTS ( ( 4, 2, 2, 2, 2, 4 ),
 ( 3, 3 ),
 ( 4.336808689942017736E-19, 0.001647923167088038423, 0.002471884750632057526, 0.003295846334176076413, 0.004943769501264114186, 0.006591692668352152826 ),
 ( 0.000000000000000000, 1.000000000000000000 ),
 .UNSPECIFIED. ) 
 GEOMETRIC_REPRESENTATION_ITEM ( )  RATIONAL_B_SPLINE_SURFACE ( (
 ( 1.000000000000000000, 0.7071067811865475727, 1.000000000000000000),
 ( 1.000000000000000000, 0.7122033721489962055, 1.000000000000000000),
 ( 1.000000000000000000, 0.7158366153114927855, 1.000000000000000000),
 ( 1.000000000000000000, 0.7192720032935935315, 1.000000000000000000),
 ( 1.000000000000000000, 0.7200809050417179558, 1.000000000000000000),
 ( 1.000000000000000000, 0.7210491446665049375, 1.000000000000000000),
 ( 1.000000000000000000, 0.7212054070303647313, 1.000000000000000000),
 ( 1.000000000000000000, 0.7207522793907679137, 1.000000000000000000),
 ( 1.000000000000000000, 0.7192424821649830990, 1.000000000000000000),
 ( 1.000000000000000000, 0.7143802006614198286, 1.000000000000000000),
 ( 1.000000000000000000, 0.7109884861397212097, 1.000000000000000000),
 ( 1.000000000000000000, 0.7071067811865492381, 1.000000000000000000) ) ) 
 REPRESENTATION_ITEM ( '' )  SURFACE ( )  );
#112873=FILL_AREA_STYLE ('',( #89695 ) ) ;
#112880=CARTESIAN_POINT ( 'NONE',  ( 16.47916666666667140, 6.094999999999988205, -1.633150327867694651 ) ) ;
#112934=CARTESIAN_POINT ( 'NONE',  ( 22.96290314143522338, -3.967499999999994476, 6.871911579029513106 ) ) ;
#112936=LINE ( 'NONE', #3440, #101164 ) ;
#112952=EDGE_CURVE ( 'NONE', #119924, #47238, #113466, .T. ) ;
#112955=DIRECTION ( 'NONE',  ( 1.000000000000000000, 0.000000000000000000, 0.000000000000000000 ) ) ;
#112957=FILL_AREA_STYLE ('',( #23064 ) ) ;
#112966=VERTEX_POINT ( 'NONE', #142219 ) ;
#112970=( GEOMETRIC_REPRESENTATION_CONTEXT ( 3 ) GLOBAL_UNCERTAINTY_ASSIGNED_CONTEXT ( ( #49040 ) ) GLOBAL_UNIT_ASSIGNED_CONTEXT ( ( #95115, #73396, #29154 ) ) REPRESENTATION_CONTEXT ( 'NONE', 'WORKASPACE' ) );
#112992=ORIENTED_EDGE ( 'NONE', *, *, #110730, .F. ) ;
#112993=COLOUR_RGB ( '', 0.72549020, 0.75294118, 0.79215686) ;
#112997=CARTESIAN_POINT ( 'NONE',  ( 32.87956980810189123, 3.967499999999998916, 6.871911579029510442 ) ) ;
#113011=( NAMED_UNIT ( * ) PLANE_ANGLE_UNIT ( ) SI_UNIT ( $, .RADIAN. ) );
#113024=UNCERTAINTY_MEASURE_WITH_UNIT (LENGTH_MEASURE( 1.000000000000000082E-05 ), #133699, 'distance_accuracy_value', 'NONE');
#113037=CARTESIAN_POINT ( 'NONE',  ( 18.06206980810188867, -7.934999999999991616, -2.126176841940955242 ) ) ;
#113057=VECTOR ( 'NONE', #37361, 1000.000000000000000 ) ;
#113065=CARTESIAN_POINT ( 'NONE',  ( 151.4000000000000057, -17.48000000000005016, -34.92499999999998295 ) ) ;
#113074=CARTESIAN_POINT ( 'NONE',  ( 52.69985579143948939, -48.99436351328167660, 39.52330221398018750 ) ) ;
#113091=CIRCLE ( 'NONE', #131638, 1.000000000000000888 ) ;
#113100=CARTESIAN_POINT ( 'NONE',  ( 0.6504031414352192675, 7.934999999999988951, -2.126176841940961904 ) ) ;
#113118=( NAMED_UNIT ( * ) PLANE_ANGLE_UNIT ( ) SI_UNIT ( $, .RADIAN. ) );
#113154=EDGE_CURVE ( 'NONE', #96033, #11916, #143185, .T. ) ;
#113162=CARTESIAN_POINT ( 'NONE',  ( 28.65040314143521982, 7.934999999999989839, -2.126176841940961904 ) ) ;
#113163=CARTESIAN_POINT ( 'NONE',  ( 2.254569808101886341, -6.871911579029512218, 3.967499999999996252 ) ) ;
#113202=ADVANCED_FACE ( 'NONE', ( #54495 ), #29848, .T. ) ;
#113213=ADVANCED_FACE ( 'NONE', ( #110953 ), #123325, .F. ) ;
#113220=CARTESIAN_POINT ( 'NONE',  ( 0.7210889554053107053, -7.059391798541635232, -2.151955493142619247 ) ) ;
#113259=STYLED_ITEM ( 'NONE', ( #59122 ), #62770 ) ;
#113310=TOROIDAL_SURFACE ( 'NONE', #78672, 31.92999999999999972, 3.000000000000000000 ) ;
#113332=CARTESIAN_POINT ( 'NONE',  ( -0.07876352523144723727, -9.717572351234235426E-16, -7.934999999999990727 ) ) ;
#113349=FILL_AREA_STYLE_COLOUR ( '', #129702 ) ;
#113366=DIRECTION ( 'NONE',  ( 0.000000000000000000, -1.000000000000000000, -5.559056632600921604E-15 ) ) ;
#113380=CARTESIAN_POINT ( 'NONE',  ( 183.4786297241425927, -52.14999999999998437, -41.05044666116291552 ) ) ;
#113383=VECTOR ( 'NONE', #51234, 1000.000000000000000 ) ;
#113405=CIRCLE ( 'NONE', #131959, 5.999999999999998224 ) ;
#113428=( NAMED_UNIT ( * ) SI_UNIT ( $, .STERADIAN. ) SOLID_ANGLE_UNIT ( ) );
#113435=COLOUR_RGB ( '', 0.09019608, 0.27058824, 0.51372549) ;
#113437=CLOSED_SHELL ( 'NONE', ( #66228, #46689, #82437, #64958, #81930, #112081, #16114, #63034, #115316, #11702, #130635, #70028, #22614, #122273, #100016, #21254, #116793, #36322, #62770, #118359, #91558, #79080, #97639, #102640, #79637, #120916, #116870, #32375, #98966, #71398, #33147, #118172, #7398, #13691, #104071, #12196, #5117, #108314, #99140, #975, #4147, #43643, #23446, #86018, #65144, #61305, #47657, #139780, #20929, #134888, #23037, #33681, #137549, #80703, #15304, #34948, #111895, #47140, #90366, #73585, #41038, #70138, #81831, #31273, #124337, #96794, #83137, #44864, #89171, #117596, #939, #95871, #90943, #22381, #40939, #93057, #111891, #62206, #82181, #18383, #27925, #75511, #44362, #79516, #88505, #141443, #16334, #124980, #38134, #82293, #95688, #68458, #37829, #88424, #116311, #128132, #109467, #51969, #124881, #87420, #137587, #87823, #21720, #13350, #33428, #2933, #28818, #64289, #131194, #65185, #98714, #41693, #248, #27794, #8773, #120064, #57143, #6157, #41826, #34639, #113213, #65678, #33707, #113202, #111305, #49850, #41202, #116432, #77853, #25975, #12766, #63723, #90553, #39731, #131026, #96714, #120045, #62638, #69272 ) ) ;
#113445=CARTESIAN_POINT ( 'NONE',  ( 3.000000000000000000, -43.14999999999999147, -31.92499999999998295 ) ) ;
#113466=LINE ( 'NONE', #58448, #113057 ) ;
#113469=DIRECTION ( 'NONE',  ( 0.000000000000000000, 0.000000000000000000, 1.000000000000000000 ) ) ;
#113475=CARTESIAN_POINT ( 'NONE',  ( 19.10416666666666785, -1.633150327867672447, -6.094999999999999751 ) ) ;
#113489=ORIENTED_EDGE ( 'NONE', *, *, #64635, .T. ) ;
#113505=CARTESIAN_POINT ( 'NONE',  ( 2.233306282870438864, -6.094999999999989981, -1.633150327867689100 ) ) ;
#113511=ORIENTED_EDGE ( 'NONE', *, *, #20578, .T. ) ;
#113515=CYLINDRICAL_SURFACE ( 'NONE', #53773, 6.094999999999989093 ) ;
#113523=VERTEX_POINT ( 'NONE', #134008 ) ;
#113534=CARTESIAN_POINT ( 'NONE',  ( 22.43706980810188867, 2.126176841940952134, -7.934999999999993392 ) ) ;
#113584=CARTESIAN_POINT ( 'NONE',  ( 24.64583333333333570, -1.633150327867689988, 6.094999999999989981 ) ) ;
#113624=( GEOMETRIC_REPRESENTATION_CONTEXT ( 3 ) GLOBAL_UNCERTAINTY_ASSIGNED_CONTEXT ( ( #37647 ) ) GLOBAL_UNIT_ASSIGNED_CONTEXT ( ( #108752, #11584, #131989 ) ) REPRESENTATION_CONTEXT ( 'NONE', 'WORKASPACE' ) );
#113627=ORIENTED_EDGE ( 'NONE', *, *, #33420, .F. ) ;
#113638=MECHANICAL_DESIGN_GEOMETRIC_PRESENTATION_REPRESENTATION('',(#95107),#139118);
#113652=ORIENTED_EDGE ( 'NONE', *, *, #143348, .T. ) ;
#113667=VECTOR ( 'NONE', #104466, 1000.000000000000000 ) ;
#113691=VECTOR ( 'NONE', #68589, 1000.000000000000000 ) ;
#113724=CARTESIAN_POINT ( 'NONE',  ( 30.54623647476855552, -7.934999999999990727, 4.858786175617117713E-16 ) ) ;
#113737=ORIENTED_EDGE ( 'NONE', *, *, #33671, .F. ) ;
#113755=PRESENTATION_STYLE_ASSIGNMENT (( #47137 ) ) ;
#113759=LINE ( 'NONE', #46409, #16117 ) ;
#113767=CARTESIAN_POINT ( 'NONE',  ( 21.99956980810188867, -3.967499999999998028, -6.871911579029511330 ) ) ;
#113780=FACE_BOUND ( 'NONE', #76772, .T. ) ;
#113808=CARTESIAN_POINT ( 'NONE',  ( 174.7500000000000000, 7.919999999999947526, -21.52769999999994965 ) ) ;
#113841=( NAMED_UNIT ( * ) SI_UNIT ( $, .STERADIAN. ) SOLID_ANGLE_UNIT ( ) );
#113859=CYLINDRICAL_SURFACE ( 'NONE', #87803, 3.999999999999989786 ) ;
#113865=EDGE_CURVE ( 'NONE', #64706, #67772, #13690, .T. ) ;
#113880=CARTESIAN_POINT ( 'NONE',  ( 25.39999999999999858, -30.18000000000009564, -12.70000000000045404 ) ) ;
#113893=CARTESIAN_POINT ( 'NONE',  ( 2.400403141435218934, -7.934999999999989839, 2.126176841940957907 ) ) ;
#113906=CARTESIAN_POINT ( 'NONE',  ( 183.7880820442461811, -48.99280962439294029, -39.49606053969851160 ) ) ;
#113929=CARTESIAN_POINT ( 'NONE',  ( 2.999999999999999112, -43.14999999999999147, -34.92499999999998295 ) ) ;
#113938=DIRECTION ( 'NONE',  ( -0.000000000000000000, 1.000000000000000000, -0.000000000000000000 ) ) ;
#113949=CARTESIAN_POINT ( 'NONE',  ( 0.4515083163331480853, -7.650011319436560875, 0.5189475094714633974 ) ) ;
#113964=CARTESIAN_POINT ( 'NONE',  ( 0.7643236001482540676, 7.174902596057846083, 1.559348790086458436 ) ) ;
#113965=FILL_AREA_STYLE_COLOUR ( '', #56818 ) ;
#113985=STYLED_ITEM ( 'NONE', ( #32570 ), #16334 ) ;
#114009=ORIENTED_EDGE ( 'NONE', *, *, #52372, .F. ) ;
#114017=CIRCLE ( 'NONE', #88578, 3.000000000000002665 ) ;
#114038=EDGE_CURVE ( 'NONE', #15743, #79053, #123291, .T. ) ;
#114062=CARTESIAN_POINT ( 'NONE',  ( 2.254569808101886341, -6.871911579029512218, 3.967499999999996252 ) ) ;
#114092=CARTESIAN_POINT ( 'NONE',  ( 7.045806282870439752, 5.278424836066143655, -3.047499999999997655 ) ) ;
#114102=CARTESIAN_POINT ( 'NONE',  ( 8.582903141435219041, 3.967499999999992699, -6.871911579029513994 ) ) ;
#114136=ORIENTED_EDGE ( 'NONE', *, *, #124687, .T. ) ;
#114158=ORIENTED_EDGE ( 'NONE', *, *, #129278, .T. ) ;
#114168=( LENGTH_UNIT ( ) NAMED_UNIT ( * ) SI_UNIT ( .MILLI., .METRE. ) );
#114192=CARTESIAN_POINT ( 'NONE',  ( 28.00000000000002487, -52.14999999999999147, 34.92500000000003268 ) ) ;
#114212=CARTESIAN_POINT ( 'NONE',  ( 25.40000000000001279, 7.747411163680002488, -1.763262371054023170 ) ) ;
#114231=CARTESIAN_POINT ( 'NONE',  ( 9.962472949537104938, -7.464222240803106570E-16, -6.094999999999989981 ) ) ;
#114263=CARTESIAN_POINT ( 'NONE',  ( 20.10373647476854941, 5.808823158059036373, 5.808823158059032821 ) ) ;
#114291=DIRECTION ( 'NONE',  ( 0.000000000000000000, 0.9976538855070753442, -0.06845965770171351383 ) ) ;
#114308=CARTESIAN_POINT ( 'NONE',  ( 26.54166666666666785, 3.047499999999993214, -5.278424836066146320 ) ) ;
#114309=DIRECTION ( 'NONE',  ( 0.000000000000000000, 1.000000000000000000, -0.000000000000000000 ) ) ;
#114313=AXIS2_PLACEMENT_3D ( 'NONE', #66141, #129953, #30654 ) ;
#114318=SURFACE_SIDE_STYLE ('',( #95236 ) ) ;
#114337=EDGE_CURVE ( 'NONE', #111908, #65308, #111335, .T. ) ;
#114346=DIRECTION ( 'NONE',  ( -1.000000000000000000, -0.000000000000000000, 0.000000000000000000 ) ) ;
#114348=AXIS2_PLACEMENT_3D ( 'NONE', #4764, #16381, #104844 ) ;
#114368=FACE_OUTER_BOUND ( 'NONE', #20203, .T. ) ;
#114411=SURFACE_STYLE_USAGE ( .BOTH. , #70937 ) ;
#114414=DIRECTION ( 'NONE',  ( 0.000000000000000000, 0.000000000000000000, 1.000000000000000000 ) ) ;
#114432=CARTESIAN_POINT ( 'NONE',  ( 27.33790314143521982, -6.871911579029513106, -3.967499999999993587 ) ) ;
#114435=ORIENTED_EDGE ( 'NONE', *, *, #107412, .T. ) ;
#114441=CYLINDRICAL_SURFACE ( 'NONE', #7908, 3.000000000000002665 ) ;
#114451=( LENGTH_UNIT ( ) NAMED_UNIT ( * ) SI_UNIT ( .MILLI., .METRE. ) );
#114457=CARTESIAN_POINT ( 'NONE',  ( 128.1499999999997499, -49.14999999999999147, 40.92499999999998295 ) ) ;
#114466=CARTESIAN_POINT ( 'NONE',  ( 29.43706980810189222, 2.126176841940952134, -7.934999999999993392 ) ) ;
#114493=DIRECTION ( 'NONE',  ( -1.000000000000000000, -0.000000000000000000, 0.000000000000000000 ) ) ;
#114495=CARTESIAN_POINT ( 'NONE',  ( 55.49226980201036952, -49.12413125935466240, 39.93743342457241141 ) ) ;
#114526=CARTESIAN_POINT ( 'NONE',  ( 0.2129031414352194063, 3.967499999999992699, -6.871911579029513994 ) ) ;
#114528=COLOUR_RGB ( '', 0.40784314, 0.44705882, 0.49803922) ;
#114578=SURFACE_STYLE_FILL_AREA ( #26865 ) ;
#114590=SURFACE_SIDE_STYLE ('',( #105155 ) ) ;
#114606=LINE ( 'NONE', #62406, #108458 ) ;
#114665=CYLINDRICAL_SURFACE ( 'NONE', #27710, 1.000000000000000000 ) ;
#114681=ORIENTED_EDGE ( 'NONE', *, *, #112697, .T. ) ;
#114716=LINE ( 'NONE', #137935, #36587 ) ;
#114750=CARTESIAN_POINT ( 'NONE',  ( 9.400403141435219823, -7.934999999999989839, 2.126176841940957907 ) ) ;
#114783=CARTESIAN_POINT ( 'NONE',  ( 9.020403141435219041, 7.934999999999989839, -2.126176841940961904 ) ) ;
#114807=CARTESIAN_POINT ( 'NONE',  ( 10.93750000000000178, -4.461849672132299105, 4.461849672132299993 ) ) ;
#114841=LINE ( 'NONE', #15519, #81132 ) ;
#114856=CYLINDRICAL_SURFACE ( 'NONE', #50182, 1.000000000000000888 ) ;
#114860=CIRCLE ( 'NONE', #17593, 9.000000000000001776 ) ;
#114889=MECHANICAL_DESIGN_GEOMETRIC_PRESENTATION_REPRESENTATION('',(#29240),#112655);
#114896=ORIENTED_EDGE ( 'NONE', *, *, #39040, .T. ) ;
#114907=CARTESIAN_POINT ( 'NONE',  ( 13.89997294953710494, 4.461849672132297329, -4.461849672132302658 ) ) ;
#114930=CARTESIAN_POINT ( 'NONE',  ( 27.99999999999999645, -49.14999999999999147, -53.92499999999967741 ) ) ;
#114935=CARTESIAN_POINT ( 'NONE',  ( 24.62456980810188867, -6.871911579029512218, 3.967499999999996252 ) ) ;
#114986=CARTESIAN_POINT ( 'NONE',  ( 26.83333333333333570, 5.278424836066143655, -3.047499999999997655 ) ) ;
#114987=FACE_OUTER_BOUND ( 'NONE', #106465, .T. ) ;
#115010=CARTESIAN_POINT ( 'NONE',  ( 1.809685201411095568, -5.249926533735820300, 3.476758287636498412 ) ) ;
#115025=STYLED_ITEM ( 'NONE', ( #45200 ), #134888 ) ;
#115028=EDGE_CURVE ( 'NONE', #103874, #84791, #8456, .T. ) ;
#115044=SURFACE_STYLE_FILL_AREA ( #48395 ) ;
#115104=VECTOR ( 'NONE', #46105, 1000.000000000000000 ) ;
#115109=CARTESIAN_POINT ( 'NONE',  ( 25.15040314143521627, 7.934999999999989839, -2.126176841940961904 ) ) ;
#115134=CARTESIAN_POINT ( 'NONE',  ( 59.09089496824513787, -46.71325913967877597, -35.40428284070723208 ) ) ;
#115152=EDGE_CURVE ( 'NONE', #51562, #15743, #78827, .T. ) ;
#115154=CARTESIAN_POINT ( 'NONE',  ( 29.58290314143522082, 3.967499999999992699, -6.871911579029513994 ) ) ;
#115155=CARTESIAN_POINT ( 'NONE',  ( 5.812069808101886892, 7.934999999999992504, 2.126176841940951689 ) ) ;
#115167=CARTESIAN_POINT ( 'NONE',  ( 23.81663961620377279, -1.633150327867672447, -6.094999999999999751 ) ) ;
#115182=CARTESIAN_POINT ( 'NONE',  ( 55.95337363913753848, -51.41954113333839871, 38.53170190052308186 ) ) ;
#115207=CARTESIAN_POINT ( 'NONE',  ( 7.358736474768553748, 5.808823158059031044, -5.808823158059037262 ) ) ;
#115212=DIRECTION ( 'NONE',  ( 0.000000000000000000, 1.000000000000000000, 0.000000000000000000 ) ) ;
#115246=MECHANICAL_DESIGN_GEOMETRIC_PRESENTATION_REPRESENTATION('',(#75983),#66774);
#115251=ORIENTED_EDGE ( 'NONE', *, *, #124687, .F. ) ;
#115256=CARTESIAN_POINT ( 'NONE',  ( 151.4000000000000057, -16.48000000000005016, 34.92499999999998295 ) ) ;
#115272=( NAMED_UNIT ( * ) PLANE_ANGLE_UNIT ( ) SI_UNIT ( $, .RADIAN. ) );
#115302=FILL_AREA_STYLE ('',( #5842 ) ) ;
#115316=ADVANCED_FACE ( 'NONE', ( #27216 ), #38125, .F. ) ;
#115321=DIRECTION ( 'NONE',  ( 0.000000000000000000, 1.000000000000000000, 6.938893903907228378E-15 ) ) ;
#115410=DIRECTION ( 'NONE',  ( -0.000000000000000000, 1.000000000000000000, 2.921639538487157626E-15 ) ) ;
#115446=SURFACE_STYLE_USAGE ( .BOTH. , #47437 ) ;
#115449=CARTESIAN_POINT ( 'NONE',  ( 7.212903141435218934, 3.967499999999992699, -6.871911579029513994 ) ) ;
#115457=VECTOR ( 'NONE', #46009, 1000.000000000000000 ) ;
#115482=CARTESIAN_POINT ( 'NONE',  ( 0.8537364747685528554, -5.808823158059035485, -5.808823158059033709 ) ) ;
#115483=LINE ( 'NONE', #142298, #52845 ) ;
#115497=MECHANICAL_DESIGN_GEOMETRIC_PRESENTATION_REPRESENTATION('',(#101672),#124861);
#115508=FACE_OUTER_BOUND ( 'NONE', #20321, .T. ) ;
#115512=UNCERTAINTY_MEASURE_WITH_UNIT (LENGTH_MEASURE( 1.000000000000000082E-05 ), #87579, 'distance_accuracy_value', 'NONE');
#115543=DIRECTION ( 'NONE',  ( 0.000000000000000000, 5.075120898959323014E-15, 1.000000000000000000 ) ) ;
#115565=VERTEX_POINT ( 'NONE', #108317 ) ;
#115577=CARTESIAN_POINT ( 'NONE',  ( 152.4000000000000057, 7.919999999999947526, 19.12499999999998224 ) ) ;
#115592=( LENGTH_UNIT ( ) NAMED_UNIT ( * ) SI_UNIT ( .MILLI., .METRE. ) );
#115595=STYLED_ITEM ( 'NONE', ( #54357 ), #70138 ) ;
#115596=CIRCLE ( 'NONE', #99475, 9.000000000000001776 ) ;
#115613=CARTESIAN_POINT ( 'NONE',  ( 18.56663961620376924, 1.633150327867695095, 6.094999999999988205 ) ) ;
#115621=( NAMED_UNIT ( * ) SI_UNIT ( $, .STERADIAN. ) SOLID_ANGLE_UNIT ( ) );
#115644=CARTESIAN_POINT ( 'NONE',  ( 181.1500000000000057, -43.14999999999999147, 34.92499999999998295 ) ) ;
#115653=CARTESIAN_POINT ( 'NONE',  ( 30.45790314143522437, 6.871911579029515771, 3.967499999999989146 ) ) ;
#115695=CARTESIAN_POINT ( 'NONE',  ( 19.68750000000000000, 4.461849672132297329, -4.461849672132302658 ) ) ;
#115710=CARTESIAN_POINT ( 'NONE',  ( 25.39999999999999858, 1.399999999999987699, -20.40202195861970580 ) ) ;
#115810=TOROIDAL_SURFACE ( 'NONE', #78822, 9.000000000000001776, 3.000000000000000000 ) ;
#115824=CARTESIAN_POINT ( 'NONE',  ( 26.46290314143521982, -3.967499999999994476, 6.871911579029513106 ) ) ;
#115835=CARTESIAN_POINT ( 'NONE',  ( 28.00000000000002487, -49.14999999999999147, 59.92500000000006111 ) ) ;
#115836=FACE_OUTER_BOUND ( 'NONE', #72356, .T. ) ;
#115855=TOROIDAL_SURFACE ( 'NONE', #78876, 25.00000000000002487, 3.000000000000000000 ) ;
#115861=LINE ( 'NONE', #114457, #122999 ) ;
#115862=UNCERTAINTY_MEASURE_WITH_UNIT (LENGTH_MEASURE( 1.000000000000000082E-05 ), #13359, 'distance_accuracy_value', 'NONE');
#115874=CARTESIAN_POINT ( 'NONE',  ( 34.54123647476855297, 0.000000000000000000, 7.934999999999990727 ) ) ;
#115876=CARTESIAN_POINT ( 'NONE',  ( 8.582903141435219041, 3.967499999999992699, -6.871911579029513994 ) ) ;
#115879=CARTESIAN_POINT ( 'NONE',  ( 0.000000000000000000, -4.600000000000013856, 20.40202195861967382 ) ) ;
#115883=CARTESIAN_POINT ( 'NONE',  ( 25.40000000000000213, 4.219727177090330628, 4.866784818621353814 ) ) ;
#115897=FILL_AREA_STYLE_COLOUR ( '', #94312 ) ;
#115904=CARTESIAN_POINT ( 'NONE',  ( 25.39999999999999858, -14.29000000000013593, -12.70000000000045404 ) ) ;
#115934=DIRECTION ( 'NONE',  ( 0.000000000000000000, -1.000000000000000000, 0.000000000000000000 ) ) ;
#115937=CARTESIAN_POINT ( 'NONE',  ( 10.42123647476855375, -9.717572351234235426E-16, -7.934999999999990727 ) ) ;
#115940=SURFACE_STYLE_FILL_AREA ( #59480 ) ;
#115976=ORIENTED_EDGE ( 'NONE', *, *, #72932, .F. ) ;
#116013=CARTESIAN_POINT ( 'NONE',  ( -1.099596858564781066, -7.934999999999989839, 2.126176841940957907 ) ) ;
#116023=EDGE_LOOP ( 'NONE', ( #104608, #78476, #5175, #21431 ) ) ;
#116026=PLANE ( 'NONE',  #142299 ) ;
#116030=CARTESIAN_POINT ( 'NONE',  ( 183.3316408629057150, -49.14999999999996305, -41.64500000000001734 ) ) ;
#116047=CARTESIAN_POINT ( 'NONE',  ( 0.000000000000000000, -49.85820393249936444, -34.92499999999998295 ) ) ;
#116055=UNCERTAINTY_MEASURE_WITH_UNIT (LENGTH_MEASURE( 1.000000000000000082E-05 ), #44317, 'distance_accuracy_value', 'NONE');
#116065=CARTESIAN_POINT ( 'NONE',  ( 2.333333333333333481, 5.278424836066143655, -3.047499999999997655 ) ) ;
#116066=( LENGTH_UNIT ( ) NAMED_UNIT ( * ) SI_UNIT ( .MILLI., .METRE. ) );
#116111=SURFACE_SIDE_STYLE ('',( #61767 ) ) ;
#116113=CARTESIAN_POINT ( 'NONE',  ( 184.1500000000000057, -57.15000000000008384, -34.92499999999998295 ) ) ;
#116119=CIRCLE ( 'NONE', #90689, 2.552699999999928693 ) ;
#116148=STYLED_ITEM ( 'NONE', ( #32964 ), #117596 ) ;
#116153=DIRECTION ( 'NONE',  ( -1.000000000000000000, -0.000000000000000000, 0.000000000000000000 ) ) ;
#116168=DIRECTION ( 'NONE',  ( 0.000000000000000000, 0.000000000000000000, -1.000000000000000000 ) ) ;
#116171=EDGE_CURVE ( 'NONE', #61213, #3140, #141286, .T. ) ;
#116191=CARTESIAN_POINT ( 'NONE',  ( 15.89583333333333393, 1.633150327867687324, -6.094999999999991758 ) ) ;
#116194=ORIENTED_EDGE ( 'NONE', *, *, #60106, .F. ) ;
#116199=EDGE_CURVE ( 'NONE', #34958, #110351, #17431, .T. ) ;
#116209=CARTESIAN_POINT ( 'NONE',  ( 12.17123647476855375, 0.000000000000000000, 7.934999999999990727 ) ) ;
#116212=EDGE_CURVE ( 'NONE', #62156, #136091, #60259, .T. ) ;
#116225=ORIENTED_EDGE ( 'NONE', *, *, #71235, .F. ) ;
#116230=ORIENTED_EDGE ( 'NONE', *, *, #8288, .F. ) ;
#116238=AXIS2_PLACEMENT_3D ( 'NONE', #31418, #114309, #93273 ) ;
#116241=CARTESIAN_POINT ( 'NONE',  ( 3.478736474768552078, -5.808823158059033709, 5.808823158059035485 ) ) ;
#116255=CARTESIAN_POINT ( 'NONE',  ( 183.3316408629057435, -52.14999999999999147, -41.64500000000001023 ) ) ;
#116296=SURFACE_STYLE_USAGE ( .BOTH. , #73523 ) ;
#116307=( GEOMETRIC_REPRESENTATION_CONTEXT ( 3 ) GLOBAL_UNCERTAINTY_ASSIGNED_CONTEXT ( ( #68168 ) ) GLOBAL_UNIT_ASSIGNED_CONTEXT ( ( #118302, #108123, #31324 ) ) REPRESENTATION_CONTEXT ( 'NONE', 'WORKASPACE' ) );
#116311=ADVANCED_FACE ( 'NONE', ( #29034 ), #102086, .T. ) ;
#116314=FILL_AREA_STYLE ('',( #72143 ) ) ;
#116370=EDGE_CURVE ( 'NONE', #141239, #132990, #95252, .T. ) ;
#116378=CARTESIAN_POINT ( 'NONE',  ( 17.39997294953710849, 4.461849672132297329, -4.461849672132302658 ) ) ;
#116413=CARTESIAN_POINT ( 'NONE',  ( 33.66623647476855297, 7.934999999999990727, -1.457635852685135314E-15 ) ) ;
#116427=CARTESIAN_POINT ( 'NONE',  ( -8.673617379884035472E-16, -49.85820393249935023, -34.92499999999999005 ) ) ;
#116432=ADVANCED_FACE ( 'NONE', ( #128805 ), #11940, .T. ) ;
#116439=ORIENTED_EDGE ( 'NONE', *, *, #48244, .F. ) ;
#116445=CARTESIAN_POINT ( 'NONE',  ( 24.39999999999999858, 1.126161369193132478, 16.41140641659140798 ) ) ;
#116456=CARTESIAN_POINT ( 'NONE',  ( 21.72916666666667140, -6.094999999999989093, 1.633150327867691765 ) ) ;
#116480=FILL_AREA_STYLE_COLOUR ( '', #54083 ) ;
#116489=FACE_OUTER_BOUND ( 'NONE', #25952, .T. ) ;
#116497=CIRCLE ( 'NONE', #54021, 3.000000000000000000 ) ;
#116500=EDGE_CURVE ( 'NONE', #126231, #104004, #62145, .T. ) ;
#116504=( BOUNDED_CURVE ( )  B_SPLINE_CURVE ( 2, ( #10188, #65332, #98626, #142858, #12332, #20339, #42143, #87764, #9449, #45022, #53729, #142168, #32690 ),
 .UNSPECIFIED., .F., .F. ) 
 B_SPLINE_CURVE_WITH_KNOTS ( ( 3, 2, 2, 2, 2, 2, 3 ),
 ( 0.6500000000000001332, 0.6583333333333334370, 0.6666666666666667407, 0.6750000000000001554, 0.6833333333333334592, 0.6916666666666667629, 0.7000000000000000666 ),
 .UNSPECIFIED. ) 
 CURVE ( )  GEOMETRIC_REPRESENTATION_ITEM ( )  RATIONAL_B_SPLINE_CURVE ( ( 0.9999999999999995559, 0.9659258262890687563, 1.000000000000000000, 0.9659258262890683122, 1.000000000000000000, 0.9659258262890683122, 1.000000000000000000, 0.9659258262890683122, 1.000000000000000000, 0.9659258262890683122, 1.000000000000000000, 0.9659258262890678681, 1.000000000000000444 ) ) 
 REPRESENTATION_ITEM ( '' )  );
#116512=CARTESIAN_POINT ( 'NONE',  ( 25.40000000000000213, -6.224491245752634683, -3.516874333047554479 ) ) ;
#116523=FILL_AREA_STYLE ('',( #105615 ) ) ;
#116524=CYLINDRICAL_SURFACE ( 'NONE', #89109, 17.45000000000002061 ) ;
#116573=CARTESIAN_POINT ( 'NONE',  ( 0.2099742459736120836, -51.66308182546811167, 38.35990878063377352 ) ) ;
#116577=CARTESIAN_POINT ( 'NONE',  ( 6.103736474768551190, 5.808823158059036373, 5.808823158059032821 ) ) ;
#116620=CARTESIAN_POINT ( 'NONE',  ( 34.24956980810188156, 3.967499999999998916, 6.871911579029510442 ) ) ;
#116621=CARTESIAN_POINT ( 'NONE',  ( 11.79123647476855297, -9.717572351234235426E-16, -7.934999999999990727 ) ) ;
#116626=ORIENTED_EDGE ( 'NONE', *, *, #9908, .F. ) ;
#116633=CARTESIAN_POINT ( 'NONE',  ( 23.67080628287044064, -3.047499999999997211, -5.278424836066143655 ) ) ;
#116645=DIRECTION ( 'NONE',  ( 1.000000000000000000, 0.000000000000000000, 0.000000000000000000 ) ) ;
#116646=CARTESIAN_POINT ( 'NONE',  ( 57.17148983091625780, -47.44491123045354897, 36.62621018406385787 ) ) ;
#116676=CARTESIAN_POINT ( 'NONE',  ( 9.400403141435219823, -7.934999999999988951, 2.126176841940957907 ) ) ;
#116707=CYLINDRICAL_SURFACE ( 'NONE', #28304, 3.999999999999989786 ) ;
#116709=EDGE_CURVE ( 'NONE', #104180, #34779, #118837, .T. ) ;
#116745=CARTESIAN_POINT ( 'NONE',  ( 8.525403141435219823, 2.126176841940962348, 7.934999999999989839 ) ) ;
#116754=FILL_AREA_STYLE_COLOUR ( '', #27789 ) ;
#116757=CARTESIAN_POINT ( 'NONE',  ( 180.6665599231034207, -49.11775834062181190, -40.20665288735654030 ) ) ;
#116769=CARTESIAN_POINT ( 'NONE',  ( 0.01254890717040265530, -50.57777258831010414, -35.91905586107258586 ) ) ;
#116770=ORIENTED_EDGE ( 'NONE', *, *, #112719, .T. ) ;
#116793=ADVANCED_FACE ( 'NONE', ( #129707 ), #19526, .F. ) ;
#116815=( LENGTH_UNIT ( ) NAMED_UNIT ( * ) SI_UNIT ( .MILLI., .METRE. ) );
#116870=ADVANCED_FACE ( 'NONE', ( #77513 ), #121676, .F. ) ;
#116882=VERTEX_POINT ( 'NONE', #39716 ) ;
#116913=SURFACE_STYLE_USAGE ( .BOTH. , #106732 ) ;
#116915=CARTESIAN_POINT ( 'NONE',  ( 13.04623647476855375, -7.934999999999990727, 4.858786175617117713E-16 ) ) ;
#116917=CARTESIAN_POINT ( 'NONE',  ( 184.1500000000000057, -43.14999999999999147, -31.92499999999998295 ) ) ;
#116920=COLOUR_RGB ( '', 0.40784314, 0.44705882, 0.49803922) ;
#116949=CARTESIAN_POINT ( 'NONE',  ( 7.853736474768552966, -5.808823158059035485, -5.808823158059033709 ) ) ;
#116988=MECHANICAL_DESIGN_GEOMETRIC_PRESENTATION_REPRESENTATION('',(#119346),#24374);
#117003=DIRECTION ( 'NONE',  ( 0.000000000000000000, 0.000000000000000000, 1.000000000000000000 ) ) ;
#117019=ORIENTED_EDGE ( 'NONE', *, *, #118953, .F. ) ;
#117044=ORIENTED_EDGE ( 'NONE', *, *, #105631, .F. ) ;
#117070=CARTESIAN_POINT ( 'NONE',  ( 15.35830628287044242, -1.633150327867689988, 6.094999999999989981 ) ) ;
#117104=CARTESIAN_POINT ( 'NONE',  ( 28.27040314143521726, -7.934999999999989839, 2.126176841940957907 ) ) ;
#117120=CARTESIAN_POINT ( 'NONE',  ( 3.221442824812127625, -48.88296141031989350, -39.14553452061910832 ) ) ;
#117145=DIRECTION ( 'NONE',  ( 1.000000000000000000, 0.000000000000000000, -0.000000000000000000 ) ) ;
#117148=CARTESIAN_POINT ( 'NONE',  ( 28.72916666666666785, -6.094999999999989093, 1.633150327867691765 ) ) ;
#117169=SURFACE_STYLE_USAGE ( .BOTH. , #94701 ) ;
#117184=CIRCLE ( 'NONE', #10596, 3.000000000000002665 ) ;
#117237=DIRECTION ( 'NONE',  ( -1.000000000000000000, -0.000000000000000000, 0.000000000000000000 ) ) ;
#117238=DIRECTION ( 'NONE',  ( 0.000000000000000000, 0.000000000000000000, -1.000000000000000000 ) ) ;
#117246=ORIENTED_EDGE ( 'NONE', *, *, #100384, .F. ) ;
#117250=CARTESIAN_POINT ( 'NONE',  ( 128.5894344200537773, -52.00875322212549179, -39.86617647058817226 ) ) ;
#117253=CARTESIAN_POINT ( 'NONE',  ( 3.187477005606119906, -48.82538788374325378, 38.96958855984426151 ) ) ;
#117258=CARTESIAN_POINT ( 'NONE',  ( 7.999569808101885116, -3.967499999999998028, -6.871911579029511330 ) ) ;
#117296=UNCERTAINTY_MEASURE_WITH_UNIT (LENGTH_MEASURE( 1.000000000000000082E-05 ), #65087, 'distance_accuracy_value', 'NONE');
#117309=CARTESIAN_POINT ( 'NONE',  ( 27.24956980810188867, 3.967499999999998916, 6.871911579029510442 ) ) ;
#117310=CARTESIAN_POINT ( 'NONE',  ( 9.457903141435219041, 6.871911579029515771, 3.967499999999989146 ) ) ;
#117343=( NAMED_UNIT ( * ) PLANE_ANGLE_UNIT ( ) SI_UNIT ( $, .RADIAN. ) );
#117365=CARTESIAN_POINT ( 'NONE',  ( 9.108736474768551972, -5.808823158059033709, 5.808823158059035485 ) ) ;
#117366=CARTESIAN_POINT ( 'NONE',  ( 22.02083333333333570, -6.094999999999989981, -1.633150327867689322 ) ) ;
#117384=MECHANICAL_DESIGN_GEOMETRIC_PRESENTATION_REPRESENTATION('',(#31740),#142883);
#117387=CARTESIAN_POINT ( 'NONE',  ( 25.39999999999999503, -2.292782931496808008, -7.607334647038449305 ) ) ;
#117399=AXIS2_PLACEMENT_3D ( 'NONE', #77639, #31270, #2 ) ;
#117410=CARTESIAN_POINT ( 'NONE',  ( 25.39999999999999858, -30.18000000000009564, 12.69999999999954454 ) ) ;
#117431=CARTESIAN_POINT ( 'NONE',  ( 5.900403141435219823, -7.934999999999989839, 2.126176841940957907 ) ) ;
#117437=FILL_AREA_STYLE_COLOUR ( '', #60306 ) ;
#117442=CARTESIAN_POINT ( 'NONE',  ( 131.6379680400227983, -49.11957940092398900, -40.22172306649559914 ) ) ;
#117451=ORIENTED_EDGE ( 'NONE', *, *, #101637, .T. ) ;
#117493=STYLED_ITEM ( 'NONE', ( #61507 ), #124881 ) ;
#117504=( LENGTH_UNIT ( ) NAMED_UNIT ( * ) SI_UNIT ( .MILLI., .METRE. ) );
#117507=CARTESIAN_POINT ( 'NONE',  ( 3.000000000000000000, -7.600000000000061817, 31.92499999999998295 ) ) ;
#117508=SURFACE_STYLE_USAGE ( .BOTH. , #17499 ) ;
#117523=DIRECTION ( 'NONE',  ( -1.000000000000000000, 0.000000000000000000, 0.000000000000000000 ) ) ;
#117540=MECHANICAL_DESIGN_GEOMETRIC_PRESENTATION_REPRESENTATION('',(#89815),#131535);
#117555=EDGE_CURVE ( 'NONE', #84791, #65885, #130842, .T. ) ;
#117557=CARTESIAN_POINT ( 'NONE',  ( 3.302882771356424829, -48.98543874033773449, 39.51758185027073722 ) ) ;
#117581=CARTESIAN_POINT ( 'NONE',  ( 19.58747294953710849, -6.094999999999989981, 3.732111120401553285E-16 ) ) ;
#117595=CARTESIAN_POINT ( 'NONE',  ( 8.087903141435219823, 6.871911579029515771, 3.967499999999989146 ) ) ;
#117596=ADVANCED_FACE ( 'NONE', ( #52528 ), #96712, .F. ) ;
#117598=ORIENTED_EDGE ( 'NONE', *, *, #86051, .F. ) ;
#117629=DIRECTION ( 'NONE',  ( 0.000000000000000000, 0.000000000000000000, 1.000000000000000000 ) ) ;
#117630=CARTESIAN_POINT ( 'NONE',  ( 15.29123647476855297, -9.717572351234235426E-16, -7.934999999999990727 ) ) ;
#117656=ORIENTED_EDGE ( 'NONE', *, *, #100819, .F. ) ;
#117685=PLANE ( 'NONE',  #73178 ) ;
#117695=CARTESIAN_POINT ( 'NONE',  ( 25.39999999999999858, -5.520864266206504263E-14, 33.92499999999998295 ) ) ;
#117735=ORIENTED_EDGE ( 'NONE', *, *, #97459, .F. ) ;
#117762=CARTESIAN_POINT ( 'NONE',  ( 17.98330628287043353, 6.094999999999991758, 1.633150327867687102 ) ) ;
#117767=VERTEX_POINT ( 'NONE', #59696 ) ;
#117811=( GEOMETRIC_REPRESENTATION_CONTEXT ( 3 ) GLOBAL_UNCERTAINTY_ASSIGNED_CONTEXT ( ( #14449 ) ) GLOBAL_UNIT_ASSIGNED_CONTEXT ( ( #74958, #51764, #85792 ) ) REPRESENTATION_CONTEXT ( 'NONE', 'WORKASPACE' ) );
#117814=CARTESIAN_POINT ( 'NONE',  ( 0.1121846519734732428, -51.37040454773406850, -37.49526731630729159 ) ) ;
#117826=VECTOR ( 'NONE', #93131, 1000.000000000000000 ) ;
#117836=LINE ( 'NONE', #92004, #106534 ) ;
#117848=CARTESIAN_POINT ( 'NONE',  ( 30.18750000000000355, 4.461849672132297329, -4.461849672132302658 ) ) ;
#117863=CARTESIAN_POINT ( 'NONE',  ( 1.689646240811447875, -4.218299268060232698, 4.823946320418484923 ) ) ;
#117881=CIRCLE ( 'NONE', #57724, 3.999999999999996447 ) ;
#117892=CARTESIAN_POINT ( 'NONE',  ( 0.000000000000000000, -1.600000000000086020, -34.92499999999998295 ) ) ;
#117894=DIRECTION ( 'NONE',  ( 0.000000000000000000, 0.000000000000000000, -1.000000000000000000 ) ) ;
#117909=CIRCLE ( 'NONE', #136370, 14.45000000000002238 ) ;
#117911=VERTEX_POINT ( 'NONE', #138680 ) ;
#117946=ORIENTED_EDGE ( 'NONE', *, *, #106636, .T. ) ;
#117948=VERTEX_POINT ( 'NONE', #19724 ) ;
#117954=DIRECTION ( 'NONE',  ( -0.000000000000000000, -1.000000000000000000, -0.000000000000000000 ) ) ;
#117957=EDGE_LOOP ( 'NONE', ( #129280, #62246, #133240, #15068 ) ) ;
#117960=CARTESIAN_POINT ( 'NONE',  ( 3.478736474768552078, -5.808823158059033709, 5.808823158059035485 ) ) ;
#117988=CARTESIAN_POINT ( 'NONE',  ( 56.39204447046056146, -48.22435659090880478, -37.54366622512048224 ) ) ;
#117996=SURFACE_STYLE_FILL_AREA ( #73825 ) ;
#118005=CARTESIAN_POINT ( 'NONE',  ( 3.354166666666666963, 1.633150327867695095, 6.094999999999988205 ) ) ;
#118006=CARTESIAN_POINT ( 'NONE',  ( 4.353736474768552966, -5.808823158059035485, -5.808823158059033709 ) ) ;
#118038=CARTESIAN_POINT ( 'NONE',  ( 54.91896556007530705, -47.51495700086010743, 36.79359617903246260 ) ) ;
#118042=AXIS2_PLACEMENT_3D ( 'NONE', #30031, #74279, #42376 ) ;
#118064=CARTESIAN_POINT ( 'NONE',  ( 11.58790314143521982, 6.871911579029515771, 3.967499999999989146 ) ) ;
#118066=CARTESIAN_POINT ( 'NONE',  ( 22.45833333333333215, -3.047499999999997211, -5.278424836066143655 ) ) ;
#118089=FILL_AREA_STYLE ('',( #27529 ) ) ;
#118142=CARTESIAN_POINT ( 'NONE',  ( 8.379569808101887674, 3.967499999999998916, 6.871911579029510442 ) ) ;
#118151=CARTESIAN_POINT ( 'NONE',  ( 174.7500000000000000, 7.919999999999947526, 21.67769999999990915 ) ) ;
#118172=ADVANCED_FACE ( 'NONE', ( #7031, #104958 ), #93378, .T. ) ;
#118183=CARTESIAN_POINT ( 'NONE',  ( 0.1600000000000010858, -7.884487147571573651, 0.9551861632841017746 ) ) ;
#118234=DIRECTION ( 'NONE',  ( 1.000000000000000000, 0.000000000000000000, 0.000000000000000000 ) ) ;
#118237=DIRECTION ( 'NONE',  ( -1.000000000000000000, 0.000000000000000000, 0.000000000000000000 ) ) ;
#118238=DIRECTION ( 'NONE',  ( 0.000000000000000000, 1.000000000000000000, 0.000000000000000000 ) ) ;
#118252=ORIENTED_EDGE ( 'NONE', *, *, #126192, .T. ) ;
#118276=DIRECTION ( 'NONE',  ( 0.000000000000000000, 0.000000000000000000, 1.000000000000000000 ) ) ;
#118290=ORIENTED_EDGE ( 'NONE', *, *, #141850, .F. ) ;
#118298=( BOUNDED_SURFACE ( )  B_SPLINE_SURFACE ( 3, 2, ( 
 ( #49993, #127533, #28230 ),
 ( #6409, #142698, #96295 ),
 ( #63731, #74604, #52114 ),
 ( #110048, #131113, #64416 ),
 ( #18749, #41229, #98475 ),
 ( #85434, #52802, #119483 ),
 ( #76753, #142007, #128958 ),
 ( #141253, #97000, #43390 ),
 ( #129662, #41964, #86179 ),
 ( #87602, #95612, #53552 ),
 ( #40543, #20173, #84746 ),
 ( #10032, #31096, #42697 ),
 ( #107889, #31796, #8556 ),
 ( #107201, #108592, #97759 ),
 ( #140539, #30359, #10722 ),
 ( #9275, #131827, #21637 ) ),
 .UNSPECIFIED., .F., .F., .F. ) 
 B_SPLINE_SURFACE_WITH_KNOTS ( ( 4, 2, 2, 2, 2, 2, 2, 4 ),
 ( 3, 3 ),
 ( 4.712388980384689674, 5.060738160973321520, 5.234912751267637887, 5.409087341561953366, 5.583261931856269733, 5.757436522150586100, 5.931611112444901579, 6.105785702739217946 ),
 ( 0.000000000000000000, 1.000000000000000000 ),
 .UNSPECIFIED. ) 
 GEOMETRIC_REPRESENTATION_ITEM ( )  RATIONAL_B_SPLINE_SURFACE ( (
 ( 1.000000000000000000, 1.000000000000000000, 1.000000000000000000),
 ( 1.000000000000000000, 1.000097732991246824, 1.000000000000000000),
 ( 1.000000000000000000, 0.9896287210064191875, 1.000000000000000000),
 ( 1.000000000000000000, 0.9608359430472837026, 1.000000000000000000),
 ( 1.000000000000000000, 0.9490805577171954610, 1.000000000000000000),
 ( 1.000000000000000000, 0.9222453908327026273, 1.000000000000000000),
 ( 1.000000000000000000, 0.9071649184813318501, 1.000000000000000000),
 ( 1.000000000000000000, 0.8751006588766834238, 1.000000000000000000),
 ( 1.000000000000000000, 0.8581174656084207264, 1.000000000000000000),
 ( 1.000000000000000000, 0.8241077986063138905, 1.000000000000000000),
 ( 1.000000000000000000, 0.8070860741946217498, 1.000000000000000000),
 ( 1.000000000000000000, 0.7752313834061490549, 1.000000000000000000),
 ( 1.000000000000000000, 0.7604116155351092754, 1.000000000000000000),
 ( 1.000000000000000000, 0.7353122387368599133, 1.000000000000000000),
 ( 1.000000000000000000, 0.7250426641248335358, 1.000000000000000000),
 ( 1.000000000000000000, 0.7180326832784525992, 1.000000000000000000) ) ) 
 REPRESENTATION_ITEM ( '' )  SURFACE ( )  );
#118302=( LENGTH_UNIT ( ) NAMED_UNIT ( * ) SI_UNIT ( .MILLI., .METRE. ) );
#118330=CARTESIAN_POINT ( 'NONE',  ( 21.65040314143522338, 7.934999999999989839, -2.126176841940961904 ) ) ;
#118351=CARTESIAN_POINT ( 'NONE',  ( 3.000000000000000000, -4.600000000000061817, 28.92500000000000426 ) ) ;
#118354=MECHANICAL_DESIGN_GEOMETRIC_PRESENTATION_REPRESENTATION('',(#106868),#11860);
#118359=ADVANCED_FACE ( 'NONE', ( #68629 ), #113515, .F. ) ;
#118361=ORIENTED_EDGE ( 'NONE', *, *, #74130, .F. ) ;
#118364=CARTESIAN_POINT ( 'NONE',  ( 12.66623647476855297, 7.934999999999990727, -1.457635852685135314E-15 ) ) ;
#118421=ORIENTED_EDGE ( 'NONE', *, *, #112443, .T. ) ;
#118487=CARTESIAN_POINT ( 'NONE',  ( 184.1500000000000057, -57.15000000000003411, 15.92499999999935589 ) ) ;
#118507=CARTESIAN_POINT ( 'NONE',  ( 23.08747294953710494, -6.094999999999989981, 3.732111120401553285E-16 ) ) ;
#118527=EDGE_LOOP ( 'NONE', ( #38934, #64564, #17923, #55431 ) ) ;
#118540=CARTESIAN_POINT ( 'NONE',  ( 32.49956980810188867, -3.967499999999998028, -6.871911579029511330 ) ) ;
#118552=CARTESIAN_POINT ( 'NONE',  ( 0.03269009326452938097, -47.89015928896886720, -37.22465919494650421 ) ) ;
#118575=EDGE_CURVE ( 'NONE', #93434, #65885, #46879, .T. ) ;
#118579=UNCERTAINTY_MEASURE_WITH_UNIT (LENGTH_MEASURE( 1.000000000000000082E-05 ), #90180, 'distance_accuracy_value', 'NONE');
#118614=ORIENTED_EDGE ( 'NONE', *, *, #113865, .F. ) ;
#118631=ORIENTED_EDGE ( 'NONE', *, *, #69687, .F. ) ;
#118646=DIRECTION ( 'NONE',  ( -1.000000000000000000, -0.000000000000000000, 0.000000000000000000 ) ) ;
#118656=ORIENTED_EDGE ( 'NONE', *, *, #46347, .F. ) ;
#118657=CARTESIAN_POINT ( 'NONE',  ( 183.9400257540257826, -51.66308182546811878, 38.35990878063730491 ) ) ;
#118658=EDGE_CURVE ( 'NONE', #91232, #68141, #54020, .T. ) ;
#118695=DIRECTION ( 'NONE',  ( -1.000000000000000000, -0.000000000000000000, 0.000000000000000000 ) ) ;
#118705=CARTESIAN_POINT ( 'NONE',  ( 0.000000000000000000, -49.85820393249939286, 34.92500000000001847 ) ) ;
#118708=CARTESIAN_POINT ( 'NONE',  ( 7.270403141435218153, -7.934999999999989839, 2.126176841940957907 ) ) ;
#118713=ORIENTED_EDGE ( 'NONE', *, *, #64815, .T. ) ;
#118735=CARTESIAN_POINT ( 'NONE',  ( 54.24578869845078799, -47.96374157527412052, -37.32649486623387247 ) ) ;
#118753=CARTESIAN_POINT ( 'NONE',  ( 7.875000000000000000, -6.094999999999989981, 3.732111120401553285E-16 ) ) ;
#118754=CARTESIAN_POINT ( 'NONE',  ( 19.81206980810188512, 7.934999999999992504, 2.126176841940951689 ) ) ;
#118760=EDGE_CURVE ( 'NONE', #137006, #26733, #77888, .T. ) ;
#118789=VECTOR ( 'NONE', #103843, 1000.000000000000227 ) ;
#118812=CARTESIAN_POINT ( 'NONE',  ( 18.44206980810188767, 7.934999999999992504, 2.126176841940951689 ) ) ;
#118830=SURFACE_STYLE_FILL_AREA ( #30406 ) ;
#118837=LINE ( 'NONE', #120974, #97399 ) ;
#118840=CARTESIAN_POINT ( 'NONE',  ( 25.40000000000000568, -1.106537714668802241, -7.868010767219997703 ) ) ;
#118841=DIRECTION ( 'NONE',  ( -0.000000000000000000, 1.000000000000000000, -0.000000000000000000 ) ) ;
#118852=( GEOMETRIC_REPRESENTATION_CONTEXT ( 3 ) GLOBAL_UNCERTAINTY_ASSIGNED_CONTEXT ( ( #88109 ) ) GLOBAL_UNIT_ASSIGNED_CONTEXT ( ( #116066, #79930, #58179 ) ) REPRESENTATION_CONTEXT ( 'NONE', 'WORKASPACE' ) );
#118872=EDGE_LOOP ( 'NONE', ( #101926, #120834, #36330, #136565, #2070, #65777 ) ) ;
#118874=( LENGTH_UNIT ( ) NAMED_UNIT ( * ) SI_UNIT ( .MILLI., .METRE. ) );
#118883=CARTESIAN_POINT ( 'NONE',  ( 9.546236474768553748, -7.934999999999990727, 4.858786175617117713E-16 ) ) ;
#118921=CARTESIAN_POINT ( 'NONE',  ( 0.1599999999999981992, -7.755134012341974525, -1.713328601965980580 ) ) ;
#118953=EDGE_CURVE ( 'NONE', #126231, #65837, #137178, .T. ) ;
#118969=PLANE ( 'NONE',  #81383 ) ;
#118992=VECTOR ( 'NONE', #134769, 1000.000000000000000 ) ;
#119012=VERTEX_POINT ( 'NONE', #102512 ) ;
#119016=PRESENTATION_STYLE_ASSIGNMENT (( #50925 ) ) ;
#119046=EDGE_CURVE ( 'NONE', #17549, #64706, #53083, .T. ) ;
#119053=CARTESIAN_POINT ( 'NONE',  ( 21.35873647476855552, 5.808823158059031044, -5.808823158059038150 ) ) ;
#119083=CARTESIAN_POINT ( 'NONE',  ( 13.24956980810188689, 3.967499999999998916, 6.871911579029510442 ) ) ;
#119088=STYLED_ITEM ( 'NONE', ( #1028 ), #120045 ) ;
#119093=PRESENTATION_STYLE_ASSIGNMENT (( #74917 ) ) ;
#119112=EDGE_CURVE ( 'NONE', #85199, #55981, #106747, .T. ) ;
#119134=DIRECTION ( 'NONE',  ( 0.000000000000000000, -1.000000000000000000, 0.000000000000000000 ) ) ;
#119143=CARTESIAN_POINT ( 'NONE',  ( 156.1500000000000057, -57.14999999999999147, 53.92499999999997584 ) ) ;
#119145=ORIENTED_EDGE ( 'NONE', *, *, #122379, .F. ) ;
#119154=EDGE_CURVE ( 'NONE', #95030, #125982, #29908, .T. ) ;
#119170=( GEOMETRIC_REPRESENTATION_CONTEXT ( 3 ) GLOBAL_UNCERTAINTY_ASSIGNED_CONTEXT ( ( #38718 ) ) GLOBAL_UNIT_ASSIGNED_CONTEXT ( ( #75788, #93614, #38516 ) ) REPRESENTATION_CONTEXT ( 'NONE', 'WORKASPACE' ) );
#119186=ORIENTED_EDGE ( 'NONE', *, *, #69978, .F. ) ;
#119198=EDGE_CURVE ( 'NONE', #68141, #33799, #77968, .T. ) ;
#119205=SURFACE_SIDE_STYLE ('',( #40948 ) ) ;
#119216=( BOUNDED_CURVE ( )  B_SPLINE_CURVE ( 2, ( #23861, #65966, #1354, #110125, #101403, #21711, #2799, #57949, #66653, #89126, #44946, #12950, #133343 ),
 .UNSPECIFIED., .F., .T. ) 
 B_SPLINE_CURVE_WITH_KNOTS ( ( 3, 2, 2, 2, 2, 2, 3 ),
 ( 0.4500000000000000111, 0.4583333333333333148, 0.4666666666666666741, 0.4749999999999999778, 0.4833333333333333370, 0.4916666666666666408, 0.5000000000000000000 ),
 .UNSPECIFIED. ) 
 CURVE ( )  GEOMETRIC_REPRESENTATION_ITEM ( )  RATIONAL_B_SPLINE_CURVE ( ( 1.000000000000000000, 0.9659258262890683122, 1.000000000000000000, 0.9659258262890683122, 1.000000000000000000, 0.9659258262890683122, 1.000000000000000000, 0.9659258262890683122, 1.000000000000000000, 0.9659258262890683122, 1.000000000000000000, 0.9659258262890683122, 1.000000000000000000 ) ) 
 REPRESENTATION_ITEM ( '' )  );
#119217=CARTESIAN_POINT ( 'NONE',  ( 22.35830628287044064, -1.633150327867689988, 6.094999999999989981 ) ) ;
#119259=CARTESIAN_POINT ( 'NONE',  ( 0.4812208760386733064, -49.11951764990739377, -40.13200514437903621 ) ) ;
#119282=ORIENTED_EDGE ( 'NONE', *, *, #7969, .F. ) ;
#119302=DIRECTION ( 'NONE',  ( 0.000000000000000000, 1.541976423090494844E-15, 1.000000000000000000 ) ) ;
#119311=VERTEX_POINT ( 'NONE', #121904 ) ;
#119338=CARTESIAN_POINT ( 'NONE',  ( 25.39999999999999858, -57.15000000000009095, 34.92499999999998295 ) ) ;
#119346=STYLED_ITEM ( 'NONE', ( #17689 ), #90943 ) ;
#119348=CARTESIAN_POINT ( 'NONE',  ( 183.3316408629058003, -52.14999999999999147, 41.64499999999997470 ) ) ;
#119374=( GEOMETRIC_REPRESENTATION_CONTEXT ( 3 ) GLOBAL_UNCERTAINTY_ASSIGNED_CONTEXT ( ( #1061 ) ) GLOBAL_UNIT_ASSIGNED_CONTEXT ( ( #107553, #137354, #129299 ) ) REPRESENTATION_CONTEXT ( 'NONE', 'WORKASPACE' ) );
#119375=( NAMED_UNIT ( * ) SI_UNIT ( $, .STERADIAN. ) SOLID_ANGLE_UNIT ( ) );
#119379=DIRECTION ( 'NONE',  ( 0.000000000000000000, 0.000000000000000000, -1.000000000000000000 ) ) ;
#119399=CARTESIAN_POINT ( 'NONE',  ( 0.2242312616537213421, -48.73293412427595683, 38.67339632249958470 ) ) ;
#119400=ORIENTED_EDGE ( 'NONE', *, *, #49610, .F. ) ;
#119401=CARTESIAN_POINT ( 'NONE',  ( -0.4587635252314473666, 0.000000000000000000, 7.934999999999990727 ) ) ;
#119409=ORIENTED_EDGE ( 'NONE', *, *, #79028, .F. ) ;
#119410=DIRECTION ( 'NONE',  ( 0.000000000000000000, 0.000000000000000000, -1.000000000000000000 ) ) ;
#119447=CARTESIAN_POINT ( 'NONE',  ( 4.666666666666666963, -5.278424836066145431, -3.047499999999993658 ) ) ;
#119448=CARTESIAN_POINT ( 'NONE',  ( 14.41623647476855297, -7.934999999999990727, 4.858786175617117713E-16 ) ) ;
#119461=CARTESIAN_POINT ( 'NONE',  ( 128.1415536296147479, -48.60795469097355692, -38.18754904899805780 ) ) ;
#119466=CYLINDRICAL_SURFACE ( 'NONE', #37904, 6.094999999999989093 ) ;
#119476=EDGE_CURVE ( 'NONE', #31146, #60580, #73280, .T. ) ;
#119483=CARTESIAN_POINT ( 'NONE',  ( 127.6280169629028762, -46.44627868284323569, 35.89947574910195272 ) ) ;
#119487=CARTESIAN_POINT ( 'NONE',  ( 183.8105469881215868, -51.90335959434331414, 39.28179725402794276 ) ) ;
#119500=CARTESIAN_POINT ( 'NONE',  ( 18.58790314143521982, 6.871911579029515771, 3.967499999999989146 ) ) ;
#119510=CARTESIAN_POINT ( 'NONE',  ( 18.52083333333333215, -6.094999999999989981, -1.633150327867689322 ) ) ;
#119521=CARTESIAN_POINT ( 'NONE',  ( 25.40000000000001634, 6.851870715257561528, -4.022987505400126729 ) ) ;
#119534=AXIS2_PLACEMENT_3D ( 'NONE', #32211, #66277, #9719 ) ;
#119550=COLOUR_RGB ( '', 0.72549020, 0.75294118, 0.79215686) ;
#119573=CARTESIAN_POINT ( 'NONE',  ( 8.962903141435219823, -3.967499999999994476, 6.871911579029513106 ) ) ;
#119581=CARTESIAN_POINT ( 'NONE',  ( 152.4000000000000057, -14.29000000000013593, 12.69999999999954632 ) ) ;
#119600=VERTEX_POINT ( 'NONE', #22416 ) ;
#119628=AXIS2_PLACEMENT_3D ( 'NONE', #105898, #92177, #38540 ) ;
#119634=CIRCLE ( 'NONE', #138197, 16.45000000000002061 ) ;
#119660=ORIENTED_EDGE ( 'NONE', *, *, #30482, .T. ) ;
#119681=COLOUR_RGB ( '', 0.31764706, 0.68627451, 0.89019608) ;
#119692=DIRECTION ( 'NONE',  ( 0.000000000000000000, 0.000000000000000000, -1.000000000000000000 ) ) ;
#119728=CARTESIAN_POINT ( 'NONE',  ( 18.85830628287044419, -1.633150327867709528, 6.094999999999979323 ) ) ;
#119740=CARTESIAN_POINT ( 'NONE',  ( 20.19206980810188767, -7.934999999999991616, -2.126176841940955242 ) ) ;
#119745=AXIS2_PLACEMENT_3D ( 'NONE', #81185, #49981, #71028 ) ;
#119754=DIRECTION ( 'NONE',  ( -0.000000000000000000, 0.000000000000000000, 1.000000000000000000 ) ) ;
#119767=ORIENTED_EDGE ( 'NONE', *, *, #44136, .T. ) ;
#119768=CARTESIAN_POINT ( 'NONE',  ( 4.083333333333333925, -5.278424836066144543, 3.047499999999995879 ) ) ;
#119770=DIRECTION ( 'NONE',  ( 0.000000000000000000, 0.000000000000000000, 1.000000000000000000 ) ) ;
#119783=SURFACE_STYLE_FILL_AREA ( #53109 ) ;
#119823=ORIENTED_EDGE ( 'NONE', *, *, #80568, .T. ) ;
#119835=CYLINDRICAL_SURFACE ( 'NONE', #23123, 6.094999999999989093 ) ;
#119843=DIRECTION ( 'NONE',  ( 0.000000000000000000, -1.000000000000000000, 0.000000000000000000 ) ) ;
#119854=CARTESIAN_POINT ( 'NONE',  ( 25.39999999999999858, -30.18000000000009564, -12.70000000000045404 ) ) ;
#119861=CARTESIAN_POINT ( 'NONE',  ( 0.000000000000000000, -7.600000000000061817, 31.92499999999998295 ) ) ;
#119880=EDGE_LOOP ( 'NONE', ( #22173, #60551, #59679, #10103, #105776, #97700 ) ) ;
#119885=ORIENTED_EDGE ( 'NONE', *, *, #40496, .F. ) ;
#119897=VERTEX_POINT ( 'NONE', #115835 ) ;
#119910=CARTESIAN_POINT ( 'NONE',  ( 20.89997294953711204, 4.461849672132297329, -4.461849672132302658 ) ) ;
#119924=VERTEX_POINT ( 'NONE', #105681 ) ;
#119986=CARTESIAN_POINT ( 'NONE',  ( 33.97916666666667851, 6.094999999999988205, -1.633150327867694651 ) ) ;
#119995=PRESENTATION_STYLE_ASSIGNMENT (( #31607 ) ) ;
#120045=ADVANCED_FACE ( 'NONE', ( #90946 ), #68233, .T. ) ;
#120046=( LENGTH_UNIT ( ) NAMED_UNIT ( * ) SI_UNIT ( .MILLI., .METRE. ) );
#120055=CARTESIAN_POINT ( 'NONE',  ( 2.044376628204111146, -6.094999999999989981, 0.4826247175876904327 ) ) ;
#120057=CIRCLE ( 'NONE', #15844, 25.00000000000002842 ) ;
#120063=COLOUR_RGB ( '', 0.40784314, 0.44705882, 0.49803922) ;
#120064=ADVANCED_FACE ( 'NONE', ( #88802 ), #38168, .T. ) ;
#120075=CARTESIAN_POINT ( 'NONE',  ( -1.266693717129561136, -6.094999999999989981, -1.633150327867689100 ) ) ;
#120086=ORIENTED_EDGE ( 'NONE', *, *, #80816, .F. ) ;
#120088=DIRECTION ( 'NONE',  ( 0.000000000000000000, 0.000000000000000000, 1.000000000000000000 ) ) ;
#120107=CARTESIAN_POINT ( 'NONE',  ( 14.56206980810188334, -7.934999999999991616, -2.126176841940955242 ) ) ;
#120148=CARTESIAN_POINT ( 'NONE',  ( 5.104166666666667851, -1.633150327867691987, -6.094999999999989093 ) ) ;
#120149=CARTESIAN_POINT ( 'NONE',  ( 19.37456980810188867, 6.871911579029510442, -3.967499999999998916 ) ) ;
#120150=SURFACE_SIDE_STYLE ('',( #97725 ) ) ;
#120156=B_SPLINE_CURVE_WITH_KNOTS ( 'NONE', 3,
 ( #140082, #109566, #97228, #65389, #62521, #106686, #10241, #117557, #86412, #63258, #30607, #7380 ),
 .UNSPECIFIED., .F., .F.,
 ( 4, 2, 2, 2, 2, 4 ),
 ( 0.000000000000000000, 0.001125297245559171450, 0.002250594491118342901, 0.002813243113897941853, 0.003375891736677540372, 0.004501188982236737843 ),
 .UNSPECIFIED. ) ;
#120160=CARTESIAN_POINT ( 'NONE',  ( 126.8009042512117333, -49.32595796886457862, -36.54674188582465888 ) ) ;
#120168=EDGE_CURVE ( 'NONE', #20276, #93784, #1101, .T. ) ;
#120175=DIRECTION ( 'NONE',  ( 0.000000000000000000, 0.000000000000000000, -1.000000000000000000 ) ) ;
#120183=EDGE_LOOP ( 'NONE', ( #83071, #55908, #84540, #24088, #80859 ) ) ;
#120201=VERTEX_POINT ( 'NONE', #121446 ) ;
#120208=CARTESIAN_POINT ( 'NONE',  ( 166.8575281714868481, 26.96999999999994202, 31.92499999999998295 ) ) ;
#120225=ORIENTED_EDGE ( 'NONE', *, *, #11689, .T. ) ;
#120256=MECHANICAL_DESIGN_GEOMETRIC_PRESENTATION_REPRESENTATION('',(#115595),#6731);
#120258=ORIENTED_EDGE ( 'NONE', *, *, #102104, .T. ) ;
#120274=CARTESIAN_POINT ( 'NONE',  ( 21.65040314143522338, 7.934999999999989839, -2.126176841940961904 ) ) ;
#120316=SURFACE_SIDE_STYLE ('',( #131238 ) ) ;
#120332=CIRCLE ( 'NONE', #60278, 6.094999999999989093 ) ;
#120352=ORIENTED_EDGE ( 'NONE', *, *, #102104, .F. ) ;
#120374=CARTESIAN_POINT ( 'NONE',  ( 156.1500000000000057, -49.14999999999999147, -45.92499999999969162 ) ) ;
#120444=CARTESIAN_POINT ( 'NONE',  ( 15.81706980810188767, -2.126176841940956130, 7.934999999999991616 ) ) ;
#120471=( NAMED_UNIT ( * ) SI_UNIT ( $, .STERADIAN. ) SOLID_ANGLE_UNIT ( ) );
#120513=FILL_AREA_STYLE_COLOUR ( '', #26032 ) ;
#120534=CARTESIAN_POINT ( 'NONE',  ( 156.1500000000000057, -49.14999999999999147, 45.92499999999998295 ) ) ;
#120556=CARTESIAN_POINT ( 'NONE',  ( 28.00000000000002487, -49.14999999999999147, -34.92499999999976978 ) ) ;
#120603=VECTOR ( 'NONE', #45335, 1000.000000000000000 ) ;
#120633=CARTESIAN_POINT ( 'NONE',  ( 25.85830628287044064, -1.633150327867689988, 6.094999999999989981 ) ) ;
#120675=ORIENTED_EDGE ( 'NONE', *, *, #5143, .T. ) ;
#120676=( NAMED_UNIT ( * ) SI_UNIT ( $, .STERADIAN. ) SOLID_ANGLE_UNIT ( ) );
#120685=VECTOR ( 'NONE', #87992, 1000.000000000000000 ) ;
#120687=PRESENTATION_STYLE_ASSIGNMENT (( #111994 ) ) ;
#120695=( GEOMETRIC_REPRESENTATION_CONTEXT ( 3 ) GLOBAL_UNCERTAINTY_ASSIGNED_CONTEXT ( ( #53504 ) ) GLOBAL_UNIT_ASSIGNED_CONTEXT ( ( #69572, #3529, #89849 ) ) REPRESENTATION_CONTEXT ( 'NONE', 'WORKASPACE' ) );
#120745=CARTESIAN_POINT ( 'NONE',  ( 55.32809448528701779, -52.14999999999999147, 41.05261164187027845 ) ) ;
#120786=ORIENTED_EDGE ( 'NONE', *, *, #103747, .T. ) ;
#120789=CARTESIAN_POINT ( 'NONE',  ( 183.7880820442500749, -48.99280962439389953, 39.49606053969937847 ) ) ;
#120817=CARTESIAN_POINT ( 'NONE',  ( -1.120860383796227655, -5.278424836066145431, -3.047499999999993658 ) ) ;
#120822=DIRECTION ( 'NONE',  ( 0.000000000000000000, 5.782411586589356455E-15, -1.000000000000000000 ) ) ;
#120825=CIRCLE ( 'NONE', #19009, 2.000000000000001776 ) ;
#120834=ORIENTED_EDGE ( 'NONE', *, *, #33224, .T. ) ;
#120845=CARTESIAN_POINT ( 'NONE',  ( 15.14540314143522082, -2.126176841940958351, -7.934999999999989839 ) ) ;
#120848=( BOUNDED_CURVE ( )  B_SPLINE_CURVE ( 2, ( #136282, #47206, #114526, #92775, #37716, #113100, #59478, #24665, #23221, #2909, #91385, #12361, #57335, #35597, #3600, #124703, #90671, #79823, #70372, #112407, #13062, #15201, #103635, #4277, #48571, #56645, #45750, #89921, #134162, #34861, #126824, #28963, #7164, #71060, #38414, #96313, #140562, #6432, #51440, #60925, #95632, #84768, #39867, #41247, #94199, #94904, #128978, #139171, #40563, #137740, #138442, #115207, #82633, #18038, #60180, #7893, #39130, #105084, #27509, #15891, #71772, #104354, #5019, #117365, #49317, #116676, #93504, #52135, #61621, #26811, #126140, #62321, #115937, #16639, #50016, #5747, #73895, #83348, #84089, #17360, #118064, #107220, #73200, #127560, #128283, #28254, #18775, #105773, #72513, #139888, #50717, #106475, #29650, #63048, #53576, #22324, #9293, #20194, #54312, #74623, #110065, #44129, #20916, #76778, #55723, #11451, #64436, #21657, #33286, #108618, #8575, #97022, #97779, #76034, #41992, #86202, #42714, #19501, #141274, #86917, #66595, #31814, #99927, #131129, #590, #65181, #109368, #118812, #119500, #142717, #10739, #43407, #55012, #99175, #77488, #130428, #31116, #75334, #85457, #129683, #107908, #52823, #23798, #123842, #12190, #101346, #45581, #135434, #69463, #133289, #100651, #59313, #103468, #68751, #58626, #112240, #102798, #78914, #112934, #136113, #124535, #13600, #81047, #57884, #57171, #44888, #125246, #122366, #36116, #102068, #67310, #1297, #133983, #2740, #47039, #1986, #25205 ),
 .UNSPECIFIED., .F., .T. ) 
 B_SPLINE_CURVE_WITH_KNOTS ( ( 3, 2, 2, 2, 2, 2, 2, 2, 2, 2, 2, 2, 2, 2, 2, 2, 2, 2, 2, 2, 2, 2, 2, 2, 2, 2, 2, 2, 2, 2, 2, 2, 2, 2, 2, 2, 2, 2, 2, 2, 2, 2, 2, 2, 2, 2, 2, 2, 2, 2, 2, 2, 2, 2, 2, 2, 2, 2, 2, 2, 2, 2, 2, 2, 2, 2, 2, 2, 2, 2, 2, 2, 2, 2, 2, 2, 2, 2, 2, 2, 2, 2, 2, 2, 2, 2, 2, 2, 3 ),
 ( 0.05679457295752499135, 0.05833333333333333426, 0.06666666666666666574, 0.07499999999999999722, 0.08333333333333332871, 0.09166666666666666019, 0.1000000000000000056, 0.1083333333333333370, 0.1166666666666666685, 0.1250000000000000000, 0.1333333333333333315, 0.1416666666666666630, 0.1499999999999999944, 0.1583333333333333259, 0.1666666666666666574, 0.1749999999999999889, 0.1833333333333333204, 0.1916666666666666796, 0.2000000000000000111, 0.2083333333333333426, 0.2166666666666666741, 0.2250000000000000056, 0.2333333333333333093, 0.2416666666666666685, 0.2500000000000000000, 0.2583333333333333592, 0.2666666666666666630, 0.2750000000000000222, 0.2833333333333333259, 0.2916666666666666852, 0.2999999999999999889, 0.3083333333333333481, 0.3166666666666666519, 0.3250000000000000111, 0.3333333333333333148, 0.3416666666666666741, 0.3499999999999999778, 0.3583333333333333370, 0.3666666666666666408, 0.3750000000000000000, 0.3833333333333333592, 0.3916666666666666630, 0.4000000000000000222, 0.4083333333333333259, 0.4166666666666666297, 0.4249999999999999889, 0.4333333333333333481, 0.4416666666666666519, 0.4500000000000000666, 0.4583333333333332593, 0.4666666666666666741, 0.4749999999999999778, 0.4833333333333333370, 0.4916666666666666408, 0.5000000000000000000, 0.5083333333333333037, 0.5166666666666668295, 0.5250000000000001332, 0.5333333333333332149, 0.5416666666666665186, 0.5500000000000000444, 0.5583333333333333481, 0.5666666666666666519, 0.5749999999999999556, 0.5833333333333333703, 0.5916666666666666741, 0.5999999999999999778, 0.6083333333333332815, 0.6166666666666666963, 0.6250000000000000000, 0.6333333333333333037, 0.6416666666666667185, 0.6500000000000000222, 0.6583333333333333259, 0.6666666666666666297, 0.6750000000000000444, 0.6833333333333333481, 0.6916666666666666519, 0.6999999999999999556, 0.7083333333333333703, 0.7166666666666666741, 0.7249999999999999778, 0.7333333333333332815, 0.7416666666666666963, 0.7500000000000000000, 0.7583333333333333037, 0.7666666666666667185, 0.7750000000000001332, 0.7779834993852963176 ),
 .UNSPECIFIED. ) 
 CURVE ( )  GEOMETRIC_REPRESENTATION_ITEM ( )  RATIONAL_B_SPLINE_CURVE ( ( 0.9897399144606364718, 0.9937081613986249451, 1.000000000000000000, 0.9659258262890683122, 1.000000000000000000, 0.9659258262890683122, 1.000000000000000000, 0.9659258262890683122, 1.000000000000000000, 0.9659258262890683122, 1.000000000000000000, 0.9659258262890683122, 1.000000000000000000, 0.9659258262890683122, 1.000000000000000000, 0.9659258262890683122, 1.000000000000000000, 0.9659258262890683122, 1.000000000000000000, 0.9659258262890683122, 1.000000000000000000, 0.9659258262890683122, 1.000000000000000000, 0.9659258262890683122, 1.000000000000000000, 0.9659258262890683122, 1.000000000000000000, 0.9659258262890683122, 1.000000000000000000, 0.9659258262890683122, 1.000000000000000000, 0.9659258262890683122, 1.000000000000000000, 0.9659258262890683122, 1.000000000000000000, 0.9659258262890683122, 1.000000000000000000, 0.9659258262890683122, 1.000000000000000000, 0.9659258262890683122, 1.000000000000000000, 0.9659258262890683122, 1.000000000000000000, 0.9659258262890683122, 1.000000000000000000, 0.9659258262890683122, 1.000000000000000000, 0.9659258262890683122, 1.000000000000000000, 0.9659258262890683122, 1.000000000000000000, 0.9659258262890683122, 1.000000000000000000, 0.9659258262890683122, 1.000000000000000000, 0.9659258262890683122, 1.000000000000000000, 0.9659258262890683122, 1.000000000000000000, 0.9659258262890683122, 1.000000000000000000, 0.9659258262890683122, 1.000000000000000000, 0.9659258262890683122, 1.000000000000000000, 0.9659258262890683122, 1.000000000000000000, 0.9659258262890683122, 1.000000000000000000, 0.9659258262890683122, 1.000000000000000000, 0.9659258262890683122, 1.000000000000000000, 0.9659258262890683122, 1.000000000000000000, 0.9659258262890683122, 1.000000000000000000, 0.9659258262890683122, 1.000000000000000000, 0.9659258262890683122, 1.000000000000000000, 0.9659258262890683122, 1.000000000000000000, 0.9659258262890683122, 1.000000000000000000, 0.9659258262890683122, 1.000000000000000000, 0.9659258262890683122, 1.000000000000000000, 0.9659258262890683122, 1.000000000000000000, 0.9659258262890683122, 1.000000000000000000, 0.9659258262890683122, 1.000000000000000000, 0.9659258262890683122, 1.000000000000000000, 0.9659258262890683122, 1.000000000000000000, 0.9659258262890683122, 1.000000000000000000, 0.9659258262890683122, 1.000000000000000000, 0.9659258262890683122, 1.000000000000000000, 0.9659258262890683122, 1.000000000000000000, 0.9659258262890683122, 1.000000000000000000, 0.9659258262890683122, 1.000000000000000000, 0.9659258262890683122, 1.000000000000000000, 0.9659258262890683122, 1.000000000000000000, 0.9659258262890683122, 1.000000000000000000, 0.9659258262890683122, 1.000000000000000000, 0.9659258262890683122, 1.000000000000000000, 0.9659258262890683122, 1.000000000000000000, 0.9659258262890683122, 1.000000000000000000, 0.9659258262890683122, 1.000000000000000000, 0.9659258262890683122, 1.000000000000000000, 0.9659258262890683122, 1.000000000000000000, 0.9659258262890683122, 1.000000000000000000, 0.9659258262890683122, 1.000000000000000000, 0.9659258262890683122, 1.000000000000000000, 0.9659258262890683122, 1.000000000000000000, 0.9659258262890683122, 1.000000000000000000, 0.9659258262890683122, 1.000000000000000000, 0.9659258262890683122, 1.000000000000000000, 0.9659258262890683122, 1.000000000000000000, 0.9659258262890683122, 1.000000000000000000, 0.9659258262890683122, 1.000000000000000000, 0.9659258262890683122, 1.000000000000000000, 0.9659258262890683122, 1.000000000000000000, 0.9659258262890683122, 1.000000000000000000, 0.9659258262890683122, 1.000000000000000000, 0.9659258262890683122, 1.000000000000000000, 0.9659258262890683122, 1.000000000000000000, 0.9659258262890683122, 1.000000000000000000, 0.9659258262890683122, 1.000000000000000000, 0.9659258262890683122, 1.000000000000000000, 0.9659258262890683122, 1.000000000000000000, 0.9659258262890683122, 1.000000000000000000, 0.9659258262890683122, 1.000000000000000000, 0.9878007668414741094, 0.9843366707940401916 ) ) 
 REPRESENTATION_ITEM ( '' )  );
#120854=CARTESIAN_POINT ( 'NONE',  ( 19.83333333333333570, 5.278424836066143655, -3.047499999999997655 ) ) ;
#120855=CARTESIAN_POINT ( 'NONE',  ( 181.1500000000000057, -43.14999999999999147, 40.92499999999998295 ) ) ;
#120870=CARTESIAN_POINT ( 'NONE',  ( 18.12913961620377279, 5.278424836066147208, 3.047499999999990550 ) ) ;
#120887=PRESENTATION_STYLE_ASSIGNMENT (( #90413 ) ) ;
#120891=CARTESIAN_POINT ( 'NONE',  ( 6.562500000000000888, 4.461849672132300881, 4.461849672132299105 ) ) ;
#120892=CARTESIAN_POINT ( 'NONE',  ( 15.87456980810188867, 6.871911579029510442, -3.967499999999998916 ) ) ;
#120912=CARTESIAN_POINT ( 'NONE',  ( 130.9531400719789929, -48.66302742222529076, -38.53170190052241395 ) ) ;
#120916=ADVANCED_FACE ( 'NONE', ( #110037 ), #86885, .F. ) ;
#120959=EDGE_CURVE ( 'NONE', #33799, #99786, #47623, .T. ) ;
#120967=SURFACE_STYLE_USAGE ( .BOTH. , #52840 ) ;
#120974=CARTESIAN_POINT ( 'NONE',  ( 25.39999999999999858, -14.29000000000013593, 12.69999999999954632 ) ) ;
#120978=ORIENTED_EDGE ( 'NONE', *, *, #18097, .F. ) ;
#120995=AXIS2_PLACEMENT_3D ( 'NONE', #64094, #87277, #108263 ) ;
#121023=CARTESIAN_POINT ( 'NONE',  ( 19.75456980810189123, -6.871911579029512218, 3.967499999999996252 ) ) ;
#121044=FILL_AREA_STYLE ('',( #76872 ) ) ;
#121127=ORIENTED_EDGE ( 'NONE', *, *, #64815, .F. ) ;
#121140=( BOUNDED_CURVE ( )  B_SPLINE_CURVE ( 2, ( #69586, #92009, #23919, #136226, #1408, #13710, #36911, #24613, #81162, #34089, #70318, #68867, #58004, #135541, #78299, #34798, #125367, #23161, #45693, #89863, #79040, #84711, #60125, #93449, #137684, #71709, #72453, #50651, #18709, #118006, #84033, #105025, #71005, #136949, #29596, #16574, #94140, #62258, #73834, #115155, #73146, #60865, #4955, #105715, #62987, #107162, #106413, #139106, #38358, #15829, #7841, #128229, #81899, #17982, #61566, #92715, #127499, #28906, #115876, #126089, #82573, #39064, #128921, #17304, #117310, #37660, #49259, #126766, #6375, #7104, #28193, #51379, #104293, #26756, #27448, #138378, #5692, #49959, #83287, #95576, #116621, #139838, #40509, #94841, #39808, #20145, #65861, #31761, #52084, #8523, #64385, #98441, #96260, #65127, #88293, #121603, #97721, #85400, #119448, #108556, #66538, #10683, #142664, #54956, #129625, #141973, #76721, #96966, #120892, #110016, #20862, #141215, #132539, #131792, #130372, #19448, #140505, #21600, #22271, #110706, #99120, #75978, #143365, #9236, #44071, #41193, #33230, #53517, #42663, #77439, #52772, #30328, #120149, #74563, #109312, #118754, #63697, #86864, #131073, #9997, #107858, #41934, #54261, #43356, #87567, #32481, #86143, #31064, #75283, #34616, #80287, #44828, #45524, #78852, #102012, #133928, #57822, #1931, #13543, #124476, #55665, #23735, #25877, #14283, #122305, #2677, #123061, #46975, #12129, #68007, #47676, #24444, #25148, #99867, #69400 ),
 .UNSPECIFIED., .F., .F. ) 
 B_SPLINE_CURVE_WITH_KNOTS ( ( 3, 2, 2, 2, 2, 2, 2, 2, 2, 2, 2, 2, 2, 2, 2, 2, 2, 2, 2, 2, 2, 2, 2, 2, 2, 2, 2, 2, 2, 2, 2, 2, 2, 2, 2, 2, 2, 2, 2, 2, 2, 2, 2, 2, 2, 2, 2, 2, 2, 2, 2, 2, 2, 2, 2, 2, 2, 2, 2, 2, 2, 2, 2, 2, 2, 2, 2, 2, 2, 2, 2, 2, 2, 2, 2, 2, 2, 2, 2, 2, 2, 2, 2, 2, 2, 2, 2, 3 ),
 ( 0.01770235391886232357, 0.02500000000000000139, 0.03333333333333333287, 0.04166666666666666435, 0.05000000000000000278, 0.05833333333333333426, 0.06666666666666665186, 0.07499999999999998335, 0.08333333333333332871, 0.09166666666666666019, 0.1000000000000000056, 0.1083333333333333370, 0.1166666666666666685, 0.1250000000000000000, 0.1333333333333333315, 0.1416666666666666630, 0.1499999999999999944, 0.1583333333333333259, 0.1666666666666666574, 0.1749999999999999889, 0.1833333333333333204, 0.1916666666666666796, 0.1999999999999999833, 0.2083333333333333426, 0.2166666666666666463, 0.2250000000000000056, 0.2333333333333333093, 0.2416666666666666685, 0.2499999999999999722, 0.2583333333333334147, 0.2666666666666666630, 0.2750000000000000222, 0.2833333333333333259, 0.2916666666666666852, 0.2999999999999999889, 0.3083333333333333481, 0.3166666666666666519, 0.3250000000000000111, 0.3333333333333333148, 0.3416666666666666741, 0.3499999999999999778, 0.3583333333333333370, 0.3666666666666666408, 0.3750000000000000000, 0.3833333333333333592, 0.3916666666666666630, 0.4000000000000000222, 0.4083333333333333259, 0.4166666666666666852, 0.4249999999999999889, 0.4333333333333333481, 0.4416666666666666519, 0.4500000000000000111, 0.4583333333333333703, 0.4666666666666666741, 0.4749999999999999778, 0.4833333333333333370, 0.4916666666666666963, 0.5000000000000000000, 0.5083333333333333037, 0.5166666666666667185, 0.5250000000000000222, 0.5333333333333333259, 0.5416666666666666297, 0.5500000000000000444, 0.5583333333333333481, 0.5666666666666666519, 0.5749999999999999556, 0.5833333333333333703, 0.5916666666666666741, 0.5999999999999999778, 0.6083333333333332815, 0.6166666666666666963, 0.6250000000000000000, 0.6333333333333333037, 0.6416666666666667185, 0.6500000000000000222, 0.6583333333333333259, 0.6666666666666666297, 0.6750000000000000444, 0.6833333333333333481, 0.6916666666666666519, 0.6999999999999999556, 0.7083333333333333703, 0.7166666666666666741, 0.7249999999999999778, 0.7333333333333332815, 0.7388014923403734002 ),
 .UNSPECIFIED. ) 
 CURVE ( )  GEOMETRIC_REPRESENTATION_ITEM ( )  RATIONAL_B_SPLINE_CURVE ( ( 0.9925829834361643567, 0.9701606487700498160, 1.000000000000000000, 0.9659258262890683122, 1.000000000000000000, 0.9659258262890683122, 1.000000000000000000, 0.9659258262890683122, 1.000000000000000000, 0.9659258262890683122, 1.000000000000000000, 0.9659258262890683122, 1.000000000000000000, 0.9659258262890683122, 1.000000000000000000, 0.9659258262890683122, 1.000000000000000000, 0.9659258262890683122, 1.000000000000000000, 0.9659258262890683122, 1.000000000000000000, 0.9659258262890683122, 1.000000000000000000, 0.9659258262890683122, 1.000000000000000000, 0.9659258262890683122, 1.000000000000000000, 0.9659258262890683122, 1.000000000000000000, 0.9659258262890683122, 1.000000000000000000, 0.9659258262890683122, 1.000000000000000000, 0.9659258262890683122, 1.000000000000000000, 0.9659258262890683122, 1.000000000000000000, 0.9659258262890683122, 1.000000000000000000, 0.9659258262890683122, 1.000000000000000000, 0.9659258262890683122, 1.000000000000000000, 0.9659258262890683122, 1.000000000000000000, 0.9659258262890683122, 1.000000000000000000, 0.9659258262890683122, 1.000000000000000000, 0.9659258262890683122, 1.000000000000000000, 0.9659258262890683122, 1.000000000000000000, 0.9659258262890683122, 1.000000000000000000, 0.9659258262890683122, 1.000000000000000000, 0.9659258262890683122, 1.000000000000000000, 0.9659258262890683122, 1.000000000000000000, 0.9659258262890683122, 1.000000000000000000, 0.9659258262890683122, 1.000000000000000000, 0.9659258262890683122, 1.000000000000000000, 0.9659258262890683122, 1.000000000000000000, 0.9659258262890683122, 1.000000000000000000, 0.9659258262890683122, 1.000000000000000000, 0.9659258262890683122, 1.000000000000000000, 0.9659258262890683122, 1.000000000000000000, 0.9659258262890683122, 1.000000000000000000, 0.9659258262890683122, 1.000000000000000000, 0.9659258262890683122, 1.000000000000000000, 0.9659258262890683122, 1.000000000000000000, 0.9659258262890683122, 1.000000000000000000, 0.9659258262890683122, 1.000000000000000000, 0.9659258262890683122, 1.000000000000000000, 0.9659258262890683122, 1.000000000000000000, 0.9659258262890683122, 1.000000000000000000, 0.9659258262890683122, 1.000000000000000000, 0.9659258262890683122, 1.000000000000000000, 0.9659258262890683122, 1.000000000000000000, 0.9659258262890683122, 1.000000000000000000, 0.9659258262890683122, 1.000000000000000000, 0.9659258262890683122, 1.000000000000000000, 0.9659258262890683122, 1.000000000000000000, 0.9659258262890683122, 1.000000000000000000, 0.9659258262890683122, 1.000000000000000000, 0.9659258262890683122, 1.000000000000000000, 0.9659258262890683122, 1.000000000000000000, 0.9659258262890683122, 1.000000000000000000, 0.9659258262890683122, 1.000000000000000000, 0.9659258262890683122, 1.000000000000000000, 0.9659258262890683122, 1.000000000000000000, 0.9659258262890683122, 1.000000000000000000, 0.9659258262890683122, 1.000000000000000000, 0.9659258262890683122, 1.000000000000000000, 0.9659258262890683122, 1.000000000000000000, 0.9659258262890683122, 1.000000000000000000, 0.9659258262890683122, 1.000000000000000000, 0.9659258262890683122, 1.000000000000000000, 0.9659258262890683122, 1.000000000000000000, 0.9659258262890683122, 1.000000000000000000, 0.9659258262890683122, 1.000000000000000000, 0.9659258262890683122, 1.000000000000000000, 0.9659258262890683122, 1.000000000000000000, 0.9659258262890683122, 1.000000000000000000, 0.9659258262890683122, 1.000000000000000000, 0.9659258262890683122, 1.000000000000000000, 0.9659258262890683122, 1.000000000000000000, 0.9659258262890683122, 1.000000000000000000, 0.9659258262890683122, 1.000000000000000000, 0.9659258262890683122, 1.000000000000000000, 0.9659258262890683122, 1.000000000000000000, 0.9659258262890683122, 1.000000000000000000, 0.9659258262890683122, 1.000000000000000000, 0.9659258262890683122, 1.000000000000000000, 0.9659258262890683122, 1.000000000000000000, 0.9776412400138145831, 0.9846251811807589238 ) ) 
 REPRESENTATION_ITEM ( '' )  );
#121153=CARTESIAN_POINT ( 'NONE',  ( 2.999999999999999112, 1.399999999999986366, 20.40202195861970580 ) ) ;
#121154=ORIENTED_EDGE ( 'NONE', *, *, #125963, .F. ) ;
#121189=CARTESIAN_POINT ( 'NONE',  ( 16.40040314143521982, -7.934999999999989839, 2.126176841940957907 ) ) ;
#121198=VERTEX_POINT ( 'NONE', #15008 ) ;
#121258=FACE_OUTER_BOUND ( 'NONE', #25776, .T. ) ;
#121283=CARTESIAN_POINT ( 'NONE',  ( 0.1600000000000007527, 1.128416843727507501, -7.874460342569484794 ) ) ;
#121298=DIRECTION ( 'NONE',  ( 0.000000000000000000, 0.000000000000000000, 1.000000000000000000 ) ) ;
#121300=FILL_AREA_STYLE ('',( #43054 ) ) ;
#121349=DIRECTION ( 'NONE',  ( -1.000000000000000000, -0.000000000000000000, 0.000000000000000000 ) ) ;
#121363=CARTESIAN_POINT ( 'NONE',  ( 25.42080628287044064, 3.047499999999997655, 5.278424836066143655 ) ) ;
#121402=FILL_AREA_STYLE_COLOUR ( '', #23366 ) ;
#121406=SURFACE_STYLE_FILL_AREA ( #122117 ) ;
#121424=LINE ( 'NONE', #99666, #6799 ) ;
#121432=UNCERTAINTY_MEASURE_WITH_UNIT (LENGTH_MEASURE( 1.000000000000000082E-05 ), #1627, 'distance_accuracy_value', 'NONE');
#121446=CARTESIAN_POINT ( 'NONE',  ( 184.1500000000000057, -30.18000000000009564, 12.69999999999954454 ) ) ;
#121473=( GEOMETRIC_REPRESENTATION_CONTEXT ( 3 ) GLOBAL_UNCERTAINTY_ASSIGNED_CONTEXT ( ( #43507 ) ) GLOBAL_UNIT_ASSIGNED_CONTEXT ( ( #29495, #15725, #126666 ) ) REPRESENTATION_CONTEXT ( 'NONE', 'WORKASPACE' ) );
#121490=DIRECTION ( 'NONE',  ( -1.000000000000000000, -0.000000000000000000, -0.000000000000000000 ) ) ;
#121492=SURFACE_SIDE_STYLE ('',( #65749 ) ) ;
#121493=FILL_AREA_STYLE_COLOUR ( '', #85998 ) ;
#121495=VERTEX_POINT ( 'NONE', #11982 ) ;
#121530=CARTESIAN_POINT ( 'NONE',  ( 0.7749729495371054933, 4.461849672132300881, 4.461849672132299105 ) ) ;
#121557=COLOUR_RGB ( '', 0.66274510, 0.83137255, 0.94901961) ;
#121559=CARTESIAN_POINT ( 'NONE',  ( 15.72873647476855297, 5.808823158059031044, -5.808823158059038150 ) ) ;
#121562=CARTESIAN_POINT ( 'NONE',  ( 27.99999999999996803, -57.14999999999999147, 49.92499999999997584 ) ) ;
#121569=( NAMED_UNIT ( * ) PLANE_ANGLE_UNIT ( ) SI_UNIT ( $, .RADIAN. ) );
#121592=UNCERTAINTY_MEASURE_WITH_UNIT (LENGTH_MEASURE( 1.000000000000000082E-05 ), #83434, 'distance_accuracy_value', 'NONE');
#121597=PRESENTATION_STYLE_ASSIGNMENT (( #77433 ) ) ;
#121602=CARTESIAN_POINT ( 'NONE',  ( 15.16666666666666785, -5.278424836066145431, -3.047499999999993658 ) ) ;
#121603=CARTESIAN_POINT ( 'NONE',  ( 13.97873647476855119, -5.808823158059033709, 5.808823158059035485 ) ) ;
#121614=CARTESIAN_POINT ( 'NONE',  ( 128.5065401839123069, -48.97294124528379911, -39.12804664298174373 ) ) ;
#121620=( LENGTH_UNIT ( ) NAMED_UNIT ( * ) SI_UNIT ( .MILLI., .METRE. ) );
#121645=AXIS2_PLACEMENT_3D ( 'NONE', #75968, #9986, #87558 ) ;
#121647=DIRECTION ( 'NONE',  ( -1.000000000000000000, -0.000000000000000000, -0.000000000000000000 ) ) ;
#121665=LINE ( 'NONE', #22335, #94239 ) ;
#121676=CYLINDRICAL_SURFACE ( 'NONE', #111274, 6.094999999999989093 ) ;
#121693=( LENGTH_UNIT ( ) NAMED_UNIT ( * ) SI_UNIT ( .MILLI., .METRE. ) );
#121694=DIRECTION ( 'NONE',  ( -0.000000000000000000, 0.000000000000000000, 1.000000000000000000 ) ) ;
#121703=LINE ( 'NONE', #20969, #94536 ) ;
#121722=EDGE_CURVE ( 'NONE', #81702, #46533, #40862, .T. ) ;
#121725=CARTESIAN_POINT ( 'NONE',  ( 16.69206980810189123, -7.934999999999991616, -2.126176841940955242 ) ) ;
#121754=VERTEX_POINT ( 'NONE', #130785 ) ;
#121756=UNCERTAINTY_MEASURE_WITH_UNIT (LENGTH_MEASURE( 1.000000000000000082E-05 ), #136385, 'distance_accuracy_value', 'NONE');
#121757=EDGE_CURVE ( 'NONE', #59558, #31597, #140209, .T. ) ;
#121769=CARTESIAN_POINT ( 'NONE',  ( 21.27040314143522437, -7.934999999999989839, 2.126176841940957907 ) ) ;
#121797=CARTESIAN_POINT ( 'NONE',  ( 61.46640106136307935, -43.14999999999999147, 34.92499999999998295 ) ) ;
#121829=ORIENTED_EDGE ( 'NONE', *, *, #109684, .T. ) ;
#121832=( NAMED_UNIT ( * ) PLANE_ANGLE_UNIT ( ) SI_UNIT ( $, .RADIAN. ) );
#121836=( GEOMETRIC_REPRESENTATION_CONTEXT ( 3 ) GLOBAL_UNCERTAINTY_ASSIGNED_CONTEXT ( ( #50640 ) ) GLOBAL_UNIT_ASSIGNED_CONTEXT ( ( #38963, #50550, #62883 ) ) REPRESENTATION_CONTEXT ( 'NONE', 'WORKASPACE' ) );
#121842=EDGE_LOOP ( 'NONE', ( #62510, #138893, #46739, #53191 ) ) ;
#121847=CARTESIAN_POINT ( 'NONE',  ( 24.69163961620376924, 6.094999999999988205, -1.633150327867694651 ) ) ;
#121851=VECTOR ( 'NONE', #119843, 1000.000000000000000 ) ;
#121860=SURFACE_SIDE_STYLE ('',( #54515 ) ) ;
#121889=CARTESIAN_POINT ( 'NONE',  ( 31.42123647476855552, -9.717572351234235426E-16, -7.934999999999990727 ) ) ;
#121896=EDGE_CURVE ( 'NONE', #121495, #108472, #124877, .T. ) ;
#121904=CARTESIAN_POINT ( 'NONE',  ( 184.1500000000000057, -49.85820393249935023, -34.92499999999998295 ) ) ;
#121949=CARTESIAN_POINT ( 'NONE',  ( 25.39999999999999858, 3.495127910064749877, 5.104374744108353568 ) ) ;
#121987=CARTESIAN_POINT ( 'NONE',  ( 184.1499999999998067, -49.14999999999999147, 34.92500000000001847 ) ) ;
#121992=EDGE_LOOP ( 'NONE', ( #61294, #118421 ) ) ;
#121997=CYLINDRICAL_SURFACE ( 'NONE', #109390, 6.094999999999989093 ) ;
#122009=MECHANICAL_DESIGN_GEOMETRIC_PRESENTATION_REPRESENTATION('',(#84981),#89632);
#122069=CARTESIAN_POINT ( 'NONE',  ( 31.54580628287043709, 5.278424836066143655, -3.047499999999997655 ) ) ;
#122075=VECTOR ( 'NONE', #105586, 1000.000000000000000 ) ;
#122100=ORIENTED_EDGE ( 'NONE', *, *, #97359, .T. ) ;
#122113=( LENGTH_UNIT ( ) NAMED_UNIT ( * ) SI_UNIT ( .MILLI., .METRE. ) );
#122117=FILL_AREA_STYLE ('',( #77239 ) ) ;
#122157=( NAMED_UNIT ( * ) PLANE_ANGLE_UNIT ( ) SI_UNIT ( $, .RADIAN. ) );
#122168=VECTOR ( 'NONE', #134018, 1000.000000000000000 ) ;
#122220=CARTESIAN_POINT ( 'NONE',  ( 2.379139616203772789, -5.278424836066145431, -3.047499999999993658 ) ) ;
#122235=CARTESIAN_POINT ( 'NONE',  ( 5.441639616203772789, -6.094999999999989093, 1.633150327867691765 ) ) ;
#122261=EDGE_CURVE ( 'NONE', #105963, #78350, #15455, .T. ) ;
#122263=CARTESIAN_POINT ( 'NONE',  ( 13.39540314143521904, 2.126176841940962348, 7.934999999999989839 ) ) ;
#122273=ADVANCED_FACE ( 'NONE', ( #55905 ), #13094, .F. ) ;
#122294=( LENGTH_UNIT ( ) NAMED_UNIT ( * ) SI_UNIT ( .MILLI., .METRE. ) );
#122304=CARTESIAN_POINT ( 'NONE',  ( 12.97916666666666607, 6.094999999999988205, -1.633150327867694651 ) ) ;
#122305=CARTESIAN_POINT ( 'NONE',  ( 24.04123647476855652, 0.000000000000000000, 7.934999999999990727 ) ) ;
#122325=EDGE_CURVE ( 'NONE', #96698, #107938, #15029, .T. ) ;
#122336=EDGE_CURVE ( 'NONE', #92907, #120201, #38236, .T. ) ;
#122366=CARTESIAN_POINT ( 'NONE',  ( 24.27540314143521982, -2.126176841940958351, -7.934999999999988951 ) ) ;
#122371=CARTESIAN_POINT ( 'NONE',  ( 166.3107925015840749, 26.96999999999993847, 33.18280220445518580 ) ) ;
#122375=ORIENTED_EDGE ( 'NONE', *, *, #60900, .F. ) ;
#122379=EDGE_CURVE ( 'NONE', #66916, #46533, #23816, .T. ) ;
#122442=CARTESIAN_POINT ( 'NONE',  ( 14.65040314143522338, 7.934999999999989839, -2.126176841940961904 ) ) ;
#122461=CARTESIAN_POINT ( 'NONE',  ( 28.00000000000002487, -52.14999999999999147, -34.92499999999976978 ) ) ;
#122462=AXIS2_PLACEMENT_3D ( 'NONE', #71434, #48242, #37377 ) ;
#122483=CARTESIAN_POINT ( 'NONE',  ( 19.81206980810188156, 7.934999999999993392, 2.126176841940951689 ) ) ;
#122531=CARTESIAN_POINT ( 'NONE',  ( 24.39999999999999858, 1.126161369193133366, -16.41140641659140798 ) ) ;
#122533=DIRECTION ( 'NONE',  ( 0.000000000000000000, 0.000000000000000000, 1.000000000000000000 ) ) ;
#122561=DIRECTION ( 'NONE',  ( 0.000000000000000000, 0.000000000000000000, 1.000000000000000000 ) ) ;
#122574=ORIENTED_EDGE ( 'NONE', *, *, #13671, .F. ) ;
#122609=CARTESIAN_POINT ( 'NONE',  ( 161.1275701981784039, 26.96999999999993491, -34.89911187425553862 ) ) ;
#122618=CARTESIAN_POINT ( 'NONE',  ( 32.29623647476855552, 7.934999999999990727, -1.457635852685135314E-15 ) ) ;
#122655=VERTEX_POINT ( 'NONE', #14148 ) ;
#122662=ORIENTED_EDGE ( 'NONE', *, *, #3843, .F. ) ;
#122669=CARTESIAN_POINT ( 'NONE',  ( 0.6598099656846050376, -7.271130854732376747, -1.582424676226277249 ) ) ;
#122686=CARTESIAN_POINT ( 'NONE',  ( 0.5657828326232884342, 7.338134074686143649, -1.735840177847257859 ) ) ;
#122692=EDGE_CURVE ( 'NONE', #21837, #103874, #99737, .T. ) ;
#122729=DIRECTION ( 'NONE',  ( -1.000000000000000000, -0.000000000000000000, -0.000000000000000000 ) ) ;
#122799=SURFACE_STYLE_FILL_AREA ( #133686 ) ;
#122800=CARTESIAN_POINT ( 'NONE',  ( 30.96247294953710494, -7.464222240803106570E-16, -6.094999999999989981 ) ) ;
#122813=ORIENTED_EDGE ( 'NONE', *, *, #68373, .T. ) ;
#122838=( NAMED_UNIT ( * ) SI_UNIT ( $, .STERADIAN. ) SOLID_ANGLE_UNIT ( ) );
#122841=STYLED_ITEM ( 'NONE', ( #138018 ), #41038 ) ;
#122867=UNCERTAINTY_MEASURE_WITH_UNIT (LENGTH_MEASURE( 1.000000000000000082E-05 ), #52406, 'distance_accuracy_value', 'NONE');
#122895=( GEOMETRIC_REPRESENTATION_CONTEXT ( 3 ) GLOBAL_UNCERTAINTY_ASSIGNED_CONTEXT ( ( #46203 ) ) GLOBAL_UNIT_ASSIGNED_CONTEXT ( ( #135310, #125850, #115621 ) ) REPRESENTATION_CONTEXT ( 'NONE', 'WORKASPACE' ) );
#122935=MECHANICAL_DESIGN_GEOMETRIC_PRESENTATION_REPRESENTATION('',(#127479),#65007);
#122976=CARTESIAN_POINT ( 'NONE',  ( 8.795806282870438864, -5.278424836066144543, 3.047499999999995879 ) ) ;
#122999=VECTOR ( 'NONE', #15129, 1000.000000000000000 ) ;
#123007=TOROIDAL_SURFACE ( 'NONE', #16490, 6.000000000000000000, 3.000000000000000000 ) ;
#123010=CARTESIAN_POINT ( 'NONE',  ( 14.12456980810188689, -6.871911579029512218, 3.967499999999996252 ) ) ;
#123038=CARTESIAN_POINT ( 'NONE',  ( 18.27497294953710494, 4.461849672132300881, 4.461849672132299105 ) ) ;
#123042=SURFACE_STYLE_FILL_AREA ( #12821 ) ;
#123048=UNCERTAINTY_MEASURE_WITH_UNIT (LENGTH_MEASURE( 1.000000000000000082E-05 ), #57990, 'distance_accuracy_value', 'NONE');
#123052=CARTESIAN_POINT ( 'NONE',  ( 152.4000000000000057, -17.48000000000005016, -12.70000000000043272 ) ) ;
#123059=CARTESIAN_POINT ( 'NONE',  ( 17.35416666666666075, 1.633150327867695095, 6.094999999999988205 ) ) ;
#123061=CARTESIAN_POINT ( 'NONE',  ( 24.33290314143522437, -3.967499999999994476, 6.871911579029513106 ) ) ;
#123062=DIRECTION ( 'NONE',  ( 0.000000000000000000, -5.075120898959323014E-15, -1.000000000000000000 ) ) ;
#123076=CARTESIAN_POINT ( 'NONE',  ( 123.3803752239611384, -44.19516442797115019, -34.92499999999998295 ) ) ;
#123080=SURFACE_STYLE_USAGE ( .BOTH. , #35380 ) ;
#123087=FILL_AREA_STYLE_COLOUR ( '', #60881 ) ;
#123103=DIRECTION ( 'NONE',  ( -1.000000000000000000, -0.000000000000000000, -0.000000000000000000 ) ) ;
#123110=AXIS2_PLACEMENT_3D ( 'NONE', #10440, #121349, #142421 ) ;
#123118=EDGE_CURVE ( 'NONE', #5341, #31146, #76893, .T. ) ;
#123124=ORIENTED_EDGE ( 'NONE', *, *, #81815, .F. ) ;
#123129=FILL_AREA_STYLE_COLOUR ( '', #38679 ) ;
#123140=AXIS2_PLACEMENT_3D ( 'NONE', #99039, #76629, #142583 ) ;
#123196=CARTESIAN_POINT ( 'NONE',  ( 20.33790314143522338, -6.871911579029513106, -3.967499999999993587 ) ) ;
#123201=CARTESIAN_POINT ( 'NONE',  ( 131.8806778009766276, -49.14999999999999147, -40.92499999999998295 ) ) ;
#123226=CARTESIAN_POINT ( 'NONE',  ( 61.46640106136302961, -43.14999999999999147, -34.92499999999998295 ) ) ;
#123233=FILL_AREA_STYLE ('',( #79025 ) ) ;
#123244=CARTESIAN_POINT ( 'NONE',  ( 19.95790314143522437, 6.871911579029515771, 3.967499999999989146 ) ) ;
#123291=( BOUNDED_CURVE ( )  B_SPLINE_CURVE ( 2, ( #77353, #120055, #133837, #20775, #122220, #43979, #65028, #67156, #88930 ),
 .UNSPECIFIED., .F., .F. ) 
 B_SPLINE_CURVE_WITH_KNOTS ( ( 3, 2, 2, 2, 3 ),
 ( 0.1224767841415644182, 0.1250000000000000000, 0.1333333333333333315, 0.1416666666666666907, 0.1500000000000000222 ),
 .UNSPECIFIED. ) 
 CURVE ( )  GEOMETRIC_REPRESENTATION_ITEM ( )  RATIONAL_B_SPLINE_CURVE ( ( 0.9856134340836057994, 0.9896828205435386216, 1.000000000000000000, 0.9659258262890683122, 1.000000000000000000, 0.9659258262890683122, 1.000000000000000000, 0.9659258262890682012, 1.000000000000000222 ) ) 
 REPRESENTATION_ITEM ( '' )  );
#123325=CYLINDRICAL_SURFACE ( 'NONE', #108574, 1.000000000000000888 ) ;
#123362=CARTESIAN_POINT ( 'NONE',  ( 166.7103603248079651, 26.96999999999993491, -32.60912447188198371 ) ) ;
#123372=CARTESIAN_POINT ( 'NONE',  ( 29.96290314143522338, -3.967499999999994476, 6.871911579029513106 ) ) ;
#123410=EDGE_CURVE ( 'NONE', #57246, #112167, #8609, .T. ) ;
#123424=VECTOR ( 'NONE', #127833, 1000.000000000000000 ) ;
#123436=CARTESIAN_POINT ( 'NONE',  ( 1.032389698926723387, -5.330271677715373357, -4.643458396899380780 ) ) ;
#123451=CARTESIAN_POINT ( 'NONE',  ( 1.260906555256695372, 1.651889767224451688, 6.634712388435225705 ) ) ;
#123452=( LENGTH_UNIT ( ) NAMED_UNIT ( * ) SI_UNIT ( .MILLI., .METRE. ) );
#123476=DIRECTION ( 'NONE',  ( 0.000000000000000000, -1.000000000000000000, 0.000000000000000000 ) ) ;
#123483=DIRECTION ( 'NONE',  ( 0.000000000000000000, 0.000000000000000000, 1.000000000000000000 ) ) ;
#123542=EDGE_CURVE ( 'NONE', #143110, #66688, #89093, .T. ) ;
#123551=CARTESIAN_POINT ( 'NONE',  ( 1.962903141435219601, -3.967499999999994476, 6.871911579029513106 ) ) ;
#123583=EDGE_CURVE ( 'NONE', #58706, #98679, #110793, .T. ) ;
#123586=PRESENTATION_STYLE_ASSIGNMENT (( #88799 ) ) ;
#123598=PRESENTATION_STYLE_ASSIGNMENT (( #111991 ) ) ;
#123601=DIRECTION ( 'NONE',  ( 0.000000000000000000, 0.000000000000000000, -1.000000000000000000 ) ) ;
#123712=CARTESIAN_POINT ( 'NONE',  ( 7.920806282870441528, 3.047499999999997655, 5.278424836066143655 ) ) ;
#123731=FILL_AREA_STYLE_COLOUR ( '', #7651 ) ;
#123742=CARTESIAN_POINT ( 'NONE',  ( 26.08290314143522082, 3.967499999999992699, -6.871911579029513994 ) ) ;
#123788=CARTESIAN_POINT ( 'NONE',  ( 12.25000000000000000, -7.464222240803106570E-16, -6.094999999999989981 ) ) ;
#123794=ORIENTED_EDGE ( 'NONE', *, *, #28551, .F. ) ;
#123800=CARTESIAN_POINT ( 'NONE',  ( 122.6835989386368055, -43.15000000000001279, -34.92499999999998295 ) ) ;
#123803=( LENGTH_UNIT ( ) NAMED_UNIT ( * ) SI_UNIT ( .MILLI., .METRE. ) );
#123841=SURFACE_STYLE_FILL_AREA ( #59312 ) ;
#123842=CARTESIAN_POINT ( 'NONE',  ( 20.77540314143522338, -2.126176841940958351, -7.934999999999988951 ) ) ;
#123844=CARTESIAN_POINT ( 'NONE',  ( 3.000000000000000444, -47.87246431468549446, -37.20487561447684755 ) ) ;
#123858=COLOUR_RGB ( '', 0.08235294, 0.09019608, 0.10196078) ;
#123863=DIRECTION ( 'NONE',  ( 0.000000000000000000, -0.000000000000000000, -1.000000000000000000 ) ) ;
#123871=ORIENTED_EDGE ( 'NONE', *, *, #119154, .F. ) ;
#123910=CARTESIAN_POINT ( 'NONE',  ( 28.79623647476855197, 7.934999999999990727, -1.457635852685135314E-15 ) ) ;
#123925=SURFACE_SIDE_STYLE ('',( #112325 ) ) ;
#123951=CARTESIAN_POINT ( 'NONE',  ( 16.60373647476855297, 5.808823158059036373, 5.808823158059032821 ) ) ;
#123962=ORIENTED_EDGE ( 'NONE', *, *, #112591, .F. ) ;
#123981=VECTOR ( 'NONE', #116645, 1000.000000000000000 ) ;
#124045=LINE ( 'NONE', #33494, #58673 ) ;
#124049=ORIENTED_EDGE ( 'NONE', *, *, #27226, .T. ) ;
#124061=CARTESIAN_POINT ( 'NONE',  ( 25.58790314143521982, 6.871911579029515771, 3.967499999999989146 ) ) ;
#124113=CARTESIAN_POINT ( 'NONE',  ( 0.3933287082456937700, -7.643270253734883113, 1.126925465033841833 ) ) ;
#124116=( BOUNDED_SURFACE ( )  B_SPLINE_SURFACE ( 3, 2, ( 
 ( #21398, #41715, #65660 ),
 ( #111230, #10492, #131586 ),
 ( #43867, #85927, #130166 ),
 ( #141761, #42462, #48150 ) ),
 .UNSPECIFIED., .F., .F., .T. ) 
 B_SPLINE_SURFACE_WITH_KNOTS ( ( 4, 4 ),
 ( 3, 3 ),
 ( 0.000000000000000000, 0.001630001914283318388 ),
 ( 0.000000000000000000, 1.000000000000000000 ),
 .UNSPECIFIED. ) 
 GEOMETRIC_REPRESENTATION_ITEM ( )  RATIONAL_B_SPLINE_SURFACE ( (
 ( 1.000000000000000000, 0.7071067811865475727, 1.000000000000000000),
 ( 1.000000000000000000, 0.7121002461815024720, 1.000000000000000000),
 ( 1.000000000000000000, 0.7157206429707747564, 1.000000000000000000),
 ( 1.000000000000000000, 0.7180326832784528213, 1.000000000000000000) ) ) 
 REPRESENTATION_ITEM ( '' )  SURFACE ( )  );
#124138=VECTOR ( 'NONE', #66594, 1000.000000000000000 ) ;
#124177=ORIENTED_EDGE ( 'NONE', *, *, #34017, .F. ) ;
#124178=AXIS2_PLACEMENT_3D ( 'NONE', #5141, #22782, #115321 ) ;
#124184=SURFACE_SIDE_STYLE ('',( #81424 ) ) ;
#124228=CARTESIAN_POINT ( 'NONE',  ( -0.6620968585647807325, -6.871911579029513106, -3.967499999999993587 ) ) ;
#124251=CARTESIAN_POINT ( 'NONE',  ( 52.26932219902325727, -52.14999999999999147, 40.92499999999998295 ) ) ;
#124252=CARTESIAN_POINT ( 'NONE',  ( 22.21247294953710494, 0.000000000000000000, 6.094999999999989981 ) ) ;
#124261=( NAMED_UNIT ( * ) PLANE_ANGLE_UNIT ( ) SI_UNIT ( $, .RADIAN. ) );
#124271=UNCERTAINTY_MEASURE_WITH_UNIT (LENGTH_MEASURE( 1.000000000000000082E-05 ), #105053, 'distance_accuracy_value', 'NONE');
#124272=CARTESIAN_POINT ( 'NONE',  ( 26.40000000000000568, -16.48000000000005016, 12.69999999999954454 ) ) ;
#124297=( BOUNDED_CURVE ( )  B_SPLINE_CURVE ( 2, ( #81911, #38370, #47855, #48526, #71724, #28206, #139117, #15158, #49273, #60880, #116633, #115167, #59438 ),
 .UNSPECIFIED., .F., .T. ) 
 B_SPLINE_CURVE_WITH_KNOTS ( ( 3, 2, 2, 2, 2, 2, 3 ),
 ( 0.7000000000000000666, 0.7083333333333334814, 0.7166666666666667851, 0.7250000000000000888, 0.7333333333333333925, 0.7416666666666668073, 0.7500000000000001110 ),
 .UNSPECIFIED. ) 
 CURVE ( )  GEOMETRIC_REPRESENTATION_ITEM ( )  RATIONAL_B_SPLINE_CURVE ( ( 0.9999999999999995559, 0.9659258262890687563, 1.000000000000000000, 0.9659258262890683122, 1.000000000000000000, 0.9659258262890683122, 1.000000000000000000, 0.9659258262890683122, 1.000000000000000000, 0.9659258262890683122, 1.000000000000000000, 0.9659258262890678681, 1.000000000000000444 ) ) 
 REPRESENTATION_ITEM ( '' )  );
#124337=ADVANCED_FACE ( 'NONE', ( #44368, #54523 ), #64667, .T. ) ;
#124386=EDGE_LOOP ( 'NONE', ( #72581, #109532, #100081, #89423 ) ) ;
#124398=CARTESIAN_POINT ( 'NONE',  ( 6.754139616203771901, 3.047499999999993214, -5.278424836066146320 ) ) ;
#124402=EDGE_CURVE ( 'NONE', #19621, #117948, #134213, .T. ) ;
#124425=CARTESIAN_POINT ( 'NONE',  ( 20.97873647476855652, -5.808823158059033709, 5.808823158059035485 ) ) ;
#124433=DIRECTION ( 'NONE',  ( 0.000000000000000000, -1.000000000000000000, 0.000000000000000000 ) ) ;
#124455=( GEOMETRIC_REPRESENTATION_CONTEXT ( 3 ) GLOBAL_UNCERTAINTY_ASSIGNED_CONTEXT ( ( #83678 ) ) GLOBAL_UNIT_ASSIGNED_CONTEXT ( ( #33804, #97597, #109912 ) ) REPRESENTATION_CONTEXT ( 'NONE', 'WORKASPACE' ) );
#124457=( NAMED_UNIT ( * ) PLANE_ANGLE_UNIT ( ) SI_UNIT ( $, .RADIAN. ) );
#124475=CARTESIAN_POINT ( 'NONE',  ( 21.43750000000000000, -4.461849672132299105, 4.461849672132299993 ) ) ;
#124476=CARTESIAN_POINT ( 'NONE',  ( 23.31206980810188512, 7.934999999999992504, 2.126176841940951689 ) ) ;
#124478=DIRECTION ( 'NONE',  ( 0.000000000000000000, -1.000000000000000000, 5.075120898959323014E-15 ) ) ;
#124488=CARTESIAN_POINT ( 'NONE',  ( 123.7287633666124265, -43.84677628532222116, -34.92499999999998295 ) ) ;
#124535=CARTESIAN_POINT ( 'NONE',  ( 23.25456980810188767, -6.871911579029512218, 3.967499999999996252 ) ) ;
#124537=DIRECTION ( 'NONE',  ( 0.000000000000000000, -1.000000000000000000, 0.000000000000000000 ) ) ;
#124542=AXIS2_PLACEMENT_3D ( 'NONE', #89605, #133145, #34518 ) ;
#124544=CARTESIAN_POINT ( 'NONE',  ( 9.770833333333333925, 6.094999999999991758, 1.633150327867686880 ) ) ;
#124564=ORIENTED_EDGE ( 'NONE', *, *, #67762, .F. ) ;
#124570=EDGE_CURVE ( 'NONE', #120201, #110351, #105821, .T. ) ;
#124598=EDGE_LOOP ( 'NONE', ( #5063, #2572, #15726, #45949 ) ) ;
#124600=CARTESIAN_POINT ( 'NONE',  ( 25.87956980810188767, 3.967499999999998916, 6.871911579029510442 ) ) ;
#124623=CARTESIAN_POINT ( 'NONE',  ( 57.88343899890125499, -48.52444309369082731, -36.09967824800666136 ) ) ;
#124642=CARTESIAN_POINT ( 'NONE',  ( 25.49956980810189222, -3.967499999999998028, -6.871911579029511330 ) ) ;
#124659=( GEOMETRIC_REPRESENTATION_CONTEXT ( 3 ) GLOBAL_UNCERTAINTY_ASSIGNED_CONTEXT ( ( #85229 ) ) GLOBAL_UNIT_ASSIGNED_CONTEXT ( ( #73057, #49864, #82481 ) ) REPRESENTATION_CONTEXT ( 'NONE', 'WORKASPACE' ) );
#124669=LINE ( 'NONE', #113065, #98280 ) ;
#124687=EDGE_CURVE ( 'NONE', #117948, #40407, #121703, .T. ) ;
#124703=CARTESIAN_POINT ( 'NONE',  ( 2.108736474768552860, -5.808823158059033709, 5.808823158059035485 ) ) ;
#124712=CIRCLE ( 'NONE', #94580, 3.999999999999989786 ) ;
#124722=DIRECTION ( 'NONE',  ( 0.000000000000000000, 0.000000000000000000, 1.000000000000000000 ) ) ;
#124743=SURFACE_SIDE_STYLE ('',( #69686 ) ) ;
#124769=CARTESIAN_POINT ( 'NONE',  ( -1.682930191898113881, -2.126176841940956130, 7.934999999999991616 ) ) ;
#124780=( NAMED_UNIT ( * ) PLANE_ANGLE_UNIT ( ) SI_UNIT ( $, .RADIAN. ) );
#124783=CARTESIAN_POINT ( 'NONE',  ( 180.9285571751891837, -48.88296141031964481, -39.14553452061820593 ) ) ;
#124796=EDGE_CURVE ( 'NONE', #45028, #5277, #110559, .T. ) ;
#124803=CARTESIAN_POINT ( 'NONE',  ( 28.00000000000002487, -49.14999999999999147, 34.92500000000003268 ) ) ;
#124814=CARTESIAN_POINT ( 'NONE',  ( 152.4000000000000057, 7.919999999999947526, -21.52769999999997808 ) ) ;
#124838=CARTESIAN_POINT ( 'NONE',  ( 1.021278265688378539, 4.989057771970841770, 5.031783612235352088 ) ) ;
#124845=ORIENTED_EDGE ( 'NONE', *, *, #100972, .T. ) ;
#124849=ORIENTED_EDGE ( 'NONE', *, *, #85006, .F. ) ;
#124860=CARTESIAN_POINT ( 'NONE',  ( 183.3316408629057435, -52.14999999999999147, -41.64500000000001023 ) ) ;
#124861=( GEOMETRIC_REPRESENTATION_CONTEXT ( 3 ) GLOBAL_UNCERTAINTY_ASSIGNED_CONTEXT ( ( #116055 ) ) GLOBAL_UNIT_ASSIGNED_CONTEXT ( ( #44317, #42891, #130614 ) ) REPRESENTATION_CONTEXT ( 'NONE', 'WORKASPACE' ) );
#124874=CARTESIAN_POINT ( 'NONE',  ( 2.999999999999999112, -43.14999999999999147, -40.92499999999998295 ) ) ;
#124877=LINE ( 'NONE', #81407, #6042 ) ;
#124881=ADVANCED_FACE ( 'NONE', ( #100699 ), #138324, .T. ) ;
#124903=FACE_BOUND ( 'NONE', #59323, .T. ) ;
#124930=ORIENTED_EDGE ( 'NONE', *, *, #47309, .F. ) ;
#124935=CARTESIAN_POINT ( 'NONE',  ( 2.837903141435219379, -6.871911579029513106, -3.967499999999993587 ) ) ;
#124947=CARTESIAN_POINT ( 'NONE',  ( 156.1500000000000057, -49.14999999999999147, 49.92499999999997584 ) ) ;
#124950=PRESENTATION_STYLE_ASSIGNMENT (( #111207 ) ) ;
#124960=CARTESIAN_POINT ( 'NONE',  ( 6.608306282870438864, 1.633150327867687324, -6.094999999999991758 ) ) ;
#124972=EDGE_CURVE ( 'NONE', #16103, #71793, #32165, .T. ) ;
#124973=CARTESIAN_POINT ( 'NONE',  ( 6.978736474768552966, -5.808823158059033709, 5.808823158059035485 ) ) ;
#124980=ADVANCED_FACE ( 'NONE', ( #39003 ), #142970, .T. ) ;
#124981=SURFACE_SIDE_STYLE ('',( #101801 ) ) ;
#124985=FACE_OUTER_BOUND ( 'NONE', #14138, .T. ) ;
#124990=DIRECTION ( 'NONE',  ( 0.000000000000000000, -1.000000000000000000, 0.000000000000000000 ) ) ;
#124995=AXIS2_PLACEMENT_3D ( 'NONE', #66393, #99708, #64973 ) ;
#125045=( NAMED_UNIT ( * ) PLANE_ANGLE_UNIT ( ) SI_UNIT ( $, .RADIAN. ) );
#125071=FILL_AREA_STYLE ('',( #38087 ) ) ;
#125078=CARTESIAN_POINT ( 'NONE',  ( 19.25000000000000355, -7.464222240803106570E-16, -6.094999999999989981 ) ) ;
#125083=( GEOMETRIC_REPRESENTATION_CONTEXT ( 3 ) GLOBAL_UNCERTAINTY_ASSIGNED_CONTEXT ( ( #14086 ) ) GLOBAL_UNIT_ASSIGNED_CONTEXT ( ( #43043, #40890, #63389 ) ) REPRESENTATION_CONTEXT ( 'NONE', 'WORKASPACE' ) );
#125095=AXIS2_PLACEMENT_3D ( 'NONE', #6022, #104655, #82929 ) ;
#125105=CARTESIAN_POINT ( 'NONE',  ( 3.399972949537105826, 4.461849672132297329, -4.461849672132302658 ) ) ;
#125113=ORIENTED_EDGE ( 'NONE', *, *, #98585, .T. ) ;
#125136=CARTESIAN_POINT ( 'NONE',  ( 25.79123647476855652, -9.717572351234235426E-16, -7.934999999999990727 ) ) ;
#125145=SURFACE_STYLE_USAGE ( .BOTH. , #23696 ) ;
#125174=DIRECTION ( 'NONE',  ( -1.000000000000000000, -0.000000000000000000, 0.000000000000000000 ) ) ;
#125191=CARTESIAN_POINT ( 'NONE',  ( 26.25000000000000355, -7.464222240803106570E-16, -6.094999999999989981 ) ) ;
#125225=MECHANICAL_DESIGN_GEOMETRIC_PRESENTATION_REPRESENTATION('',(#122841),#141349);
#125229=CIRCLE ( 'NONE', #18708, 3.999999999999989786 ) ;
#125246=CARTESIAN_POINT ( 'NONE',  ( 24.12956980810188767, -3.967499999999998028, -6.871911579029511330 ) ) ;
#125249=FACE_OUTER_BOUND ( 'NONE', #65554, .T. ) ;
#125255=CARTESIAN_POINT ( 'NONE',  ( 8.750000000000000000, -7.464222240803106570E-16, -6.094999999999989981 ) ) ;
#125320=COLOUR_RGB ( '', 0.66274510, 0.83137255, 0.94901961) ;
#125321=CARTESIAN_POINT ( 'NONE',  ( 27.62956980810189123, -3.967499999999998028, -6.871911579029511330 ) ) ;
#125335=SURFACE_SIDE_STYLE ('',( #59389 ) ) ;
#125366=CARTESIAN_POINT ( 'NONE',  ( 31.91623647476855297, -7.934999999999990727, 4.858786175617117713E-16 ) ) ;
#125367=CARTESIAN_POINT ( 'NONE',  ( 2.457903141435219485, 6.871911579029515771, 3.967499999999989146 ) ) ;
#125369=CIRCLE ( 'NONE', #62881, 3.999999999999996447 ) ;
#125379=ORIENTED_EDGE ( 'NONE', *, *, #40579, .F. ) ;
#125400=DIRECTION ( 'NONE',  ( 0.000000000000000000, 0.000000000000000000, 1.000000000000000000 ) ) ;
#125477=SURFACE_STYLE_USAGE ( .BOTH. , #134949 ) ;
#125485=SURFACE_SIDE_STYLE ('',( #114578 ) ) ;
#125496=CARTESIAN_POINT ( 'NONE',  ( 5.025403141435220711, 2.126176841940962348, 7.934999999999989839 ) ) ;
#125526=EDGE_CURVE ( 'NONE', #138987, #24260, #85125, .T. ) ;
#125561=PRESENTATION_STYLE_ASSIGNMENT (( #37845 ) ) ;
#125574=CARTESIAN_POINT ( 'NONE',  ( 0.3964375652403131500, 6.305472576662640272, -4.436123002877206289 ) ) ;
#125597=MECHANICAL_DESIGN_GEOMETRIC_PRESENTATION_REPRESENTATION('',(#113985),#70045);
#125603=STYLED_ITEM ( 'NONE', ( #16051 ), #130635 ) ;
#125624=PRODUCT_DEFINITION_CONTEXT ( 'detailed design', #112406, 'design' ) ;
#125647=CARTESIAN_POINT ( 'NONE',  ( 56.09683561313696032, -51.20434817233908831, -36.87500513592858198 ) ) ;
#125671=CARTESIAN_POINT ( 'NONE',  ( 10.12956980810188767, -3.967499999999998028, -6.871911579029511330 ) ) ;
#125702=CARTESIAN_POINT ( 'NONE',  ( 7.483306282870439752, 6.094999999999991758, 1.633150327867686880 ) ) ;
#125711=CARTESIAN_POINT ( 'NONE',  ( 8.145403141435220817, -2.126176841940958351, -7.934999999999989839 ) ) ;
#125738=FILL_AREA_STYLE_COLOUR ( '', #140293 ) ;
#125742=UNCERTAINTY_MEASURE_WITH_UNIT (LENGTH_MEASURE( 1.000000000000000082E-05 ), #130108, 'distance_accuracy_value', 'NONE');
#125781=( NAMED_UNIT ( * ) SI_UNIT ( $, .STERADIAN. ) SOLID_ANGLE_UNIT ( ) );
#125798=AXIS2_PLACEMENT_3D ( 'NONE', #124874, #111867, #123483 ) ;
#125832=( BOUNDED_CURVE ( )  B_SPLINE_CURVE ( 2, ( #72771, #139437, #27058, #38664, #29200, #82893, #51691, #60443, #18294, #106021, #37963, #49570, #62565 ),
 .UNSPECIFIED., .F., .T. ) 
 B_SPLINE_CURVE_WITH_KNOTS ( ( 3, 2, 2, 2, 2, 2, 3 ),
 ( 0.3500000000000000333, 0.3583333333333333925, 0.3666666666666666963, 0.3750000000000001110, 0.3833333333333334703, 0.3916666666666667740, 0.4000000000000001332 ),
 .UNSPECIFIED. ) 
 CURVE ( )  GEOMETRIC_REPRESENTATION_ITEM ( )  RATIONAL_B_SPLINE_CURVE ( ( 0.9999999999999997780, 0.9659258262890685343, 1.000000000000000000, 0.9659258262890683122, 1.000000000000000000, 0.9659258262890683122, 1.000000000000000000, 0.9659258262890683122, 1.000000000000000000, 0.9659258262890683122, 1.000000000000000000, 0.9659258262890678681, 1.000000000000000444 ) ) 
 REPRESENTATION_ITEM ( '' )  );
#125843=CARTESIAN_POINT ( 'NONE',  ( 12.58747294953710671, -6.094999999999989981, 3.732111120401553285E-16 ) ) ;
#125850=( NAMED_UNIT ( * ) PLANE_ANGLE_UNIT ( ) SI_UNIT ( $, .RADIAN. ) );
#125866=SURFACE_STYLE_FILL_AREA ( #101228 ) ;
#125873=( GEOMETRIC_REPRESENTATION_CONTEXT ( 3 ) GLOBAL_UNCERTAINTY_ASSIGNED_CONTEXT ( ( #27111 ) ) GLOBAL_UNIT_ASSIGNED_CONTEXT ( ( #49107, #16422, #94700 ) ) REPRESENTATION_CONTEXT ( 'NONE', 'WORKASPACE' ) );
#125876=CARTESIAN_POINT ( 'NONE',  ( 23.02040314143522082, 7.934999999999989839, -2.126176841940961904 ) ) ;
#125920=CARTESIAN_POINT ( 'NONE',  ( 25.52083333333332860, -6.094999999999989981, -1.633150327867689100 ) ) ;
#125942=FILL_AREA_STYLE ('',( #116480 ) ) ;
#125963=EDGE_CURVE ( 'NONE', #24682, #96698, #3503, .T. ) ;
#125976=CARTESIAN_POINT ( 'NONE',  ( 2.999999999999999112, -47.62213595499956398, -36.92499999999996874 ) ) ;
#125982=VERTEX_POINT ( 'NONE', #39020 ) ;
#125984=CARTESIAN_POINT ( 'NONE',  ( 10.20833333333333570, 3.047499999999997655, 5.278424836066143655 ) ) ;
#126002=ORIENTED_EDGE ( 'NONE', *, *, #48904, .T. ) ;
#126046=CARTESIAN_POINT ( 'NONE',  ( 24.42123647476855552, -9.717572351234235426E-16, -7.934999999999990727 ) ) ;
#126078=UNCERTAINTY_MEASURE_WITH_UNIT (LENGTH_MEASURE( 1.000000000000000082E-05 ), #1733, 'distance_accuracy_value', 'NONE');
#126088=CARTESIAN_POINT ( 'NONE',  ( 25.93706980810189222, 2.126176841940952134, -7.934999999999993392 ) ) ;
#126089=CARTESIAN_POINT ( 'NONE',  ( 8.728736474768551190, 5.808823158059031044, -5.808823158059037262 ) ) ;
#126109=EDGE_CURVE ( 'NONE', #129906, #137014, #41336, .T. ) ;
#126122=FILL_AREA_STYLE ('',( #15868 ) ) ;
#126123=DIRECTION ( 'NONE',  ( -0.5150380749100710309, 1.049727191138606123E-16, -0.8571673007021021196 ) ) ;
#126128=TOROIDAL_SURFACE ( 'NONE', #21900, 25.00000000000002487, 3.000000000000000000 ) ;
#126133=SURFACE_SIDE_STYLE ('',( #100277 ) ) ;
#126140=CARTESIAN_POINT ( 'NONE',  ( 10.12956980810188767, -3.967499999999998028, -6.871911579029511330 ) ) ;
#126180=SURFACE_STYLE_USAGE ( .BOTH. , #124743 ) ;
#126190=( NAMED_UNIT ( * ) PLANE_ANGLE_UNIT ( ) SI_UNIT ( $, .RADIAN. ) );
#126192=EDGE_CURVE ( 'NONE', #46533, #81376, #120057, .T. ) ;
#126195=CARTESIAN_POINT ( 'NONE',  ( 156.1500000000000057, -57.14999999999999147, 49.92499999999997584 ) ) ;
#126203=CARTESIAN_POINT ( 'NONE',  ( -1.828763525231447584, 0.000000000000000000, 7.934999999999990727 ) ) ;
#126208=( NAMED_UNIT ( * ) PLANE_ANGLE_UNIT ( ) SI_UNIT ( $, .RADIAN. ) );
#126216=DIRECTION ( 'NONE',  ( 0.000000000000000000, -0.000000000000000000, -1.000000000000000000 ) ) ;
#126219=( BOUNDED_CURVE ( )  B_SPLINE_CURVE ( 2, ( #102527, #124960, #25646, #15447, #114092, #59052, #103203, #125702, #70633, #59736, #103898, #48853, #93053 ),
 .UNSPECIFIED., .F., .T. ) 
 B_SPLINE_CURVE_WITH_KNOTS ( ( 3, 2, 2, 2, 2, 2, 3 ),
 ( 0.2500000000000000000, 0.2583333333333333592, 0.2666666666666666630, 0.2750000000000000222, 0.2833333333333333814, 0.2916666666666667407, 0.3000000000000000444 ),
 .UNSPECIFIED. ) 
 CURVE ( )  GEOMETRIC_REPRESENTATION_ITEM ( )  RATIONAL_B_SPLINE_CURVE ( ( 1.000000000000000000, 0.9659258262890683122, 1.000000000000000000, 0.9659258262890683122, 1.000000000000000000, 0.9659258262890683122, 1.000000000000000000, 0.9659258262890683122, 1.000000000000000000, 0.9659258262890683122, 1.000000000000000000, 0.9659258262890680902, 1.000000000000000222 ) ) 
 REPRESENTATION_ITEM ( '' )  );
#126231=VERTEX_POINT ( 'NONE', #80242 ) ;
#126274=CARTESIAN_POINT ( 'NONE',  ( 149.2199999999997999, -3.180000000000061444, -34.92499999999998295 ) ) ;
#126288=FILL_AREA_STYLE ('',( #71939 ) ) ;
#126308=AXIS2_PLACEMENT_3D ( 'NONE', #59811, #103980, #36604 ) ;
#126346=CARTESIAN_POINT ( 'NONE',  ( 17.35416666666666430, 1.633150327867695095, 6.094999999999988205 ) ) ;
#126352=ORIENTED_EDGE ( 'NONE', *, *, #45968, .F. ) ;
#126360=CARTESIAN_POINT ( 'NONE',  ( 4.442069808101886785, 7.934999999999993392, 2.126176841940951689 ) ) ;
#126393=CARTESIAN_POINT ( 'NONE',  ( 9.457903141435219041, 6.871911579029515771, 3.967499999999989146 ) ) ;
#126417=CARTESIAN_POINT ( 'NONE',  ( 11.52083333333333393, -6.094999999999989981, -1.633150327867689322 ) ) ;
#126506=CARTESIAN_POINT ( 'NONE',  ( 181.1391930515557931, -48.09618305010687322, -37.50858089739956824 ) ) ;
#126523=CIRCLE ( 'NONE', #142694, 17.45000000000002061 ) ;
#126524=CARTESIAN_POINT ( 'NONE',  ( 16.52497294953710494, -4.461849672132299993, -4.461849672132299105 ) ) ;
#126550=CARTESIAN_POINT ( 'NONE',  ( 22.72873647476856007, 5.808823158059031044, -5.808823158059038150 ) ) ;
#126590=( LENGTH_UNIT ( ) NAMED_UNIT ( * ) SI_UNIT ( .MILLI., .METRE. ) );
#126596=CARTESIAN_POINT ( 'NONE',  ( 19.97916666666667140, 6.094999999999988205, -1.633150327867694651 ) ) ;
#126666=( NAMED_UNIT ( * ) SI_UNIT ( $, .STERADIAN. ) SOLID_ANGLE_UNIT ( ) );
#126693=DIRECTION ( 'NONE',  ( -1.000000000000000000, -0.000000000000000000, -0.000000000000000000 ) ) ;
#126700=CARTESIAN_POINT ( 'NONE',  ( 131.5423521607622490, -49.05583548141700589, 39.86617647058822911 ) ) ;
#126712=( NAMED_UNIT ( * ) PLANE_ANGLE_UNIT ( ) SI_UNIT ( $, .RADIAN. ) );
#126717=CARTESIAN_POINT ( 'NONE',  ( 30.10873647476854842, -5.808823158059033709, 5.808823158059035485 ) ) ;
#126722=ORIENTED_EDGE ( 'NONE', *, *, #5143, .F. ) ;
#126765=CARTESIAN_POINT ( 'NONE',  ( 33.95790314143522437, 6.871911579029515771, 3.967499999999989146 ) ) ;
#126766=CARTESIAN_POINT ( 'NONE',  ( 9.895403141435220817, 2.126176841940962348, 7.934999999999988951 ) ) ;
#126777=( NAMED_UNIT ( * ) SI_UNIT ( $, .STERADIAN. ) SOLID_ANGLE_UNIT ( ) );
#126785=DIRECTION ( 'NONE',  ( 0.000000000000000000, -1.091707662666338270E-16, 1.000000000000000000 ) ) ;
#126795=FILL_AREA_STYLE ('',( #80482 ) ) ;
#126824=CARTESIAN_POINT ( 'NONE',  ( 4.296236474768552860, 7.934999999999990727, -1.457635852685135314E-15 ) ) ;
#126827=FACE_OUTER_BOUND ( 'NONE', #21802, .T. ) ;
#126834=EDGE_CURVE ( 'NONE', #141737, #106911, #117881, .T. ) ;
#126839=CARTESIAN_POINT ( 'NONE',  ( 6.854166666666666963, 1.633150327867685103, 6.094999999999992646 ) ) ;
#126852=AXIS2_PLACEMENT_3D ( 'NONE', #77691, #22542, #34905 ) ;
#126861=DIRECTION ( 'NONE',  ( 0.000000000000000000, 0.000000000000000000, -1.000000000000000000 ) ) ;
#126873=PLANE ( 'NONE',  #51708 ) ;
#126875=ORIENTED_EDGE ( 'NONE', *, *, #65035, .F. ) ;
#126885=CARTESIAN_POINT ( 'NONE',  ( 4.150403141435219823, 7.934999999999989839, -2.126176841940961904 ) ) ;
#126900=ORIENTED_EDGE ( 'NONE', *, *, #25823, .T. ) ;
#126933=CARTESIAN_POINT ( 'NONE',  ( 2.000000000000011546, 2.638703287232806449, -5.494203305479936184 ) ) ;
#126945=EDGE_CURVE ( 'NONE', #74861, #46809, #11402, .T. ) ;
#127052=CARTESIAN_POINT ( 'NONE',  ( 17.50000000000000000, 0.000000000000000000, 6.094999999999989981 ) ) ;
#127069=ORIENTED_EDGE ( 'NONE', *, *, #58611, .F. ) ;
#127074=CARTESIAN_POINT ( 'NONE',  ( 11.58790314143521982, 6.871911579029515771, 3.967499999999989146 ) ) ;
#127076=ORIENTED_EDGE ( 'NONE', *, *, #107743, .F. ) ;
#127078=CARTESIAN_POINT ( 'NONE',  ( 24.79166666666667140, -3.047499999999994547, 5.278424836066145431 ) ) ;
#127101=CARTESIAN_POINT ( 'NONE',  ( 5.374569808101886892, 6.871911579029510442, -3.967499999999998916 ) ) ;
#127117=( NAMED_UNIT ( * ) SI_UNIT ( $, .STERADIAN. ) SOLID_ANGLE_UNIT ( ) );
#127136=UNCERTAINTY_MEASURE_WITH_UNIT (LENGTH_MEASURE( 1.000000000000000082E-05 ), #59065, 'distance_accuracy_value', 'NONE');
#127230=ORIENTED_EDGE ( 'NONE', *, *, #96776, .F. ) ;
#127236=( BOUNDED_SURFACE ( )  B_SPLINE_SURFACE ( 3, 2, ( 
 ( #58766, #47868, #15861 ),
 ( #70348, #94169, #113074 ),
 ( #26088, #114495, #71034 ),
 ( #115182, #48547, #13744 ),
 ( #58034, #7130, #73175 ),
 ( #84737, #28225, #51412 ),
 ( #63018, #139137, #8549 ),
 ( #127527, #50683, #118038 ),
 ( #75307, #141245, #18741 ),
 ( #95604, #116646, #97753 ),
 ( #107192, #52794, #139861 ),
 ( #31089, #107881, #74595 ),
 ( #7867, #52106, #61591 ),
 ( #29622, #96994, #94875 ),
 ( #39840, #40536, #41958 ),
 ( #84060, #96287, #18008 ) ),
 .UNSPECIFIED., .F., .F., .F. ) 
 B_SPLINE_SURFACE_WITH_KNOTS ( ( 4, 2, 2, 2, 2, 2, 2, 4 ),
 ( 3, 3 ),
 ( 6.460584911619955406, 6.634759501914270885, 6.808934092208587252, 6.983108682502903619, 7.157283272797219098, 7.331457863091534577, 7.505632453385850944, 7.853981633974482790 ),
 ( 0.000000000000000000, 1.000000000000000000 ),
 .UNSPECIFIED. ) 
 GEOMETRIC_REPRESENTATION_ITEM ( )  RATIONAL_B_SPLINE_SURFACE ( (
 ( 1.000000000000000000, 0.7180326832784528213, 1.000000000000000000),
 ( 1.000000000000000000, 0.7250426641247393889, 1.000000000000000000),
 ( 1.000000000000000000, 0.7353122387369821489, 1.000000000000000000),
 ( 1.000000000000000000, 0.7604116155349861517, 1.000000000000000000),
 ( 1.000000000000000000, 0.7752313834058587316, 1.000000000000000000),
 ( 1.000000000000000000, 0.8070860741949156258, 1.000000000000000000),
 ( 1.000000000000000000, 0.8241077986061052796, 1.000000000000000000),
 ( 1.000000000000000000, 0.8581174656086261177, 1.000000000000000000),
 ( 1.000000000000000000, 0.8751006588767553662, 1.000000000000000000),
 ( 1.000000000000000000, 0.9071649184812575761, 1.000000000000000000),
 ( 1.000000000000000000, 0.9222453908328933636, 1.000000000000000000),
 ( 1.000000000000000000, 0.9490805577170023932, 1.000000000000000000),
 ( 1.000000000000000000, 0.9608359430471253848, 1.000000000000000000),
 ( 1.000000000000000000, 0.9896287210067384876, 1.000000000000000000),
 ( 1.000000000000000000, 1.000097732991006572, 1.000000000000000000),
 ( 1.000000000000000000, 1.000000000000000000, 1.000000000000000000) ) ) 
 REPRESENTATION_ITEM ( '' )  SURFACE ( )  );
#127238=CARTESIAN_POINT ( 'NONE',  ( 14.62913961620377101, 5.278424836066147208, 3.047499999999990550 ) ) ;
#127273=CARTESIAN_POINT ( 'NONE',  ( 30.31206980810188512, 7.934999999999993392, 2.126176841940951689 ) ) ;
#127282=CARTESIAN_POINT ( 'NONE',  ( 55.56056557994604361, -52.00875322212549179, -39.86617647058817937 ) ) ;
#127284=UNCERTAINTY_MEASURE_WITH_UNIT (LENGTH_MEASURE( 1.000000000000000082E-05 ), #7776, 'distance_accuracy_value', 'NONE');
#127288=CARTESIAN_POINT ( 'NONE',  ( 3.060608989244803180, -48.47007572038050682, -38.12657027910872642 ) ) ;
#127303=VERTEX_POINT ( 'NONE', #70101 ) ;
#127305=EDGE_CURVE ( 'NONE', #28418, #89687, #112144, .T. ) ;
#127311=SURFACE_STYLE_USAGE ( .BOTH. , #59249 ) ;
#127321=CARTESIAN_POINT ( 'NONE',  ( 20.41666666666667140, 5.278424836066147208, 3.047499999999990550 ) ) ;
#127323=EDGE_CURVE ( 'NONE', #25649, #104004, #115596, .T. ) ;
#127349=CARTESIAN_POINT ( 'NONE',  ( 1.729826228151208900, -4.601789674110575490, 4.401668811681049398 ) ) ;
#127374=MECHANICAL_DESIGN_GEOMETRIC_PRESENTATION_REPRESENTATION('',(#55688),#136685);
#127377=CARTESIAN_POINT ( 'NONE',  ( 25.39999999999999503, -6.374147713795669468, -2.268615643378129043 ) ) ;
#127390=PRESENTATION_STYLE_ASSIGNMENT (( #128136 ) ) ;
#127405=CARTESIAN_POINT ( 'NONE',  ( 12.87913961620377279, -5.278424836066145431, -3.047499999999993658 ) ) ;
#127429=SURFACE_STYLE_FILL_AREA ( #83225 ) ;
#127447=CARTESIAN_POINT ( 'NONE',  ( 4.499569808101886004, -3.967499999999998028, -6.871911579029511330 ) ) ;
#127455=CARTESIAN_POINT ( 'NONE',  ( 152.4000000000000057, 0.000000000000000000, 33.92499999999998295 ) ) ;
#127479=STYLED_ITEM ( 'NONE', ( #119093 ), #82437 ) ;
#127485=UNCERTAINTY_MEASURE_WITH_UNIT (LENGTH_MEASURE( 1.000000000000000082E-05 ), #31779, 'distance_accuracy_value', 'NONE');
#127497=CARTESIAN_POINT ( 'NONE',  ( 33.22873647476855297, 5.808823158059031044, -5.808823158059038150 ) ) ;
#127499=CARTESIAN_POINT ( 'NONE',  ( 8.291236474768552966, -9.717572351234235426E-16, -7.934999999999990727 ) ) ;
#127505=ORIENTED_EDGE ( 'NONE', *, *, #12704, .F. ) ;
#127512=( GEOMETRIC_REPRESENTATION_CONTEXT ( 3 ) GLOBAL_UNCERTAINTY_ASSIGNED_CONTEXT ( ( #12993 ) ) GLOBAL_UNIT_ASSIGNED_CONTEXT ( ( #36176, #126712, #27400 ) ) REPRESENTATION_CONTEXT ( 'NONE', 'WORKASPACE' ) );
#127527=CARTESIAN_POINT ( 'NONE',  ( 57.10144406050385868, -49.69743550128991671, 36.79359617903139679 ) ) ;
#127533=CARTESIAN_POINT ( 'NONE',  ( 122.6835989386367345, -43.14999999999999147, 34.92499999999998295 ) ) ;
#127534=CARTESIAN_POINT ( 'NONE',  ( 8.312500000000000000, -4.461849672132299993, -4.461849672132299105 ) ) ;
#127560=CARTESIAN_POINT ( 'NONE',  ( 12.02540314143521982, 2.126176841940962348, 7.934999999999988951 ) ) ;
#127602=CIRCLE ( 'NONE', #30321, 3.000000000000000444 ) ;
#127605=( NAMED_UNIT ( * ) SI_UNIT ( $, .STERADIAN. ) SOLID_ANGLE_UNIT ( ) );
#127610=DIRECTION ( 'NONE',  ( 0.000000000000000000, -1.000000000000000000, -1.286409696682840916E-16 ) ) ;
#127627=DIRECTION ( 'NONE',  ( 0.000000000000000000, 0.000000000000000000, 1.000000000000000000 ) ) ;
#127636=CARTESIAN_POINT ( 'NONE',  ( -0.3704301918981141029, -3.967499999999998028, -6.871911579029511330 ) ) ;
#127648=STYLED_ITEM ( 'NONE', ( #37048 ), #73585 ) ;
#127667=CARTESIAN_POINT ( 'NONE',  ( 0.2535635638417852444, -51.76057561339556656, -38.69631370864703257 ) ) ;
#127691=MECHANICAL_DESIGN_GEOMETRIC_PRESENTATION_REPRESENTATION('',(#67586),#90655);
#127697=ORIENTED_EDGE ( 'NONE', *, *, #28551, .T. ) ;
#127704=SURFACE_STYLE_FILL_AREA ( #83490 ) ;
#127714=SURFACE_SIDE_STYLE ('',( #87581 ) ) ;
#127716=( NAMED_UNIT ( * ) SI_UNIT ( $, .STERADIAN. ) SOLID_ANGLE_UNIT ( ) );
#127736=AXIS2_PLACEMENT_3D ( 'NONE', #634, #99222, #143460 ) ;
#127765=( NAMED_UNIT ( * ) PLANE_ANGLE_UNIT ( ) SI_UNIT ( $, .RADIAN. ) );
#127792=PRESENTATION_STYLE_ASSIGNMENT (( #63954 ) ) ;
#127800=CARTESIAN_POINT ( 'NONE',  ( 16.62500000000000000, 6.094999999999989981, -1.119633336120465690E-15 ) ) ;
#127818=SURFACE_STYLE_FILL_AREA ( #129207 ) ;
#127819=CARTESIAN_POINT ( 'NONE',  ( 7.796236474768553748, 7.934999999999990727, -1.457635852685135314E-15 ) ) ;
#127825=EDGE_CURVE ( 'NONE', #104004, #45858, #244, .T. ) ;
#127833=DIRECTION ( 'NONE',  ( -0.000000000000000000, 0.000000000000000000, 1.000000000000000000 ) ) ;
#127855=CARTESIAN_POINT ( 'NONE',  ( 7.562069808101887780, -7.934999999999991616, -2.126176841940955242 ) ) ;
#127863=CARTESIAN_POINT ( 'NONE',  ( 128.8219055147127960, -52.14999999999999147, 41.05261164187028555 ) ) ;
#127870=CARTESIAN_POINT ( 'NONE',  ( 183.8964364361580692, -51.76057561339556656, -38.69631370864702546 ) ) ;
#127880=AXIS2_PLACEMENT_3D ( 'NONE', #8925, #141658, #53195 ) ;
#127902=COLOUR_RGB ( '', 0.31764706, 0.68627451, 0.89019608) ;
#127912=( GEOMETRIC_REPRESENTATION_CONTEXT ( 3 ) GLOBAL_UNCERTAINTY_ASSIGNED_CONTEXT ( ( #108546 ) ) GLOBAL_UNIT_ASSIGNED_CONTEXT ( ( #60894, #79800, #102934 ) ) REPRESENTATION_CONTEXT ( 'NONE', 'WORKASPACE' ) );
#127923=CARTESIAN_POINT ( 'NONE',  ( 61.46640106136307935, -57.15000000000009095, 34.92499999999998295 ) ) ;
#127995=CARTESIAN_POINT ( 'NONE',  ( 20.31663961620377279, -1.633150327867691987, -6.094999999999989093 ) ) ;
#128027=CARTESIAN_POINT ( 'NONE',  ( 33.52040314143522437, 7.934999999999989839, -2.126176841940961904 ) ) ;
#128040=CARTESIAN_POINT ( 'NONE',  ( 0.8183591370940841436, -49.14999999999998437, -41.64500000000001023 ) ) ;
#128060=SURFACE_SIDE_STYLE ('',( #140340 ) ) ;
#128070=CARTESIAN_POINT ( 'NONE',  ( 30.77083333333333215, 6.094999999999991758, 1.633150327867687102 ) ) ;
#128093=CARTESIAN_POINT ( 'NONE',  ( 1.419567793309648884, -0.7546808561705602436, 6.635328531539133934 ) ) ;
#128099=STYLED_ITEM ( 'NONE', ( #26922 ), #102640 ) ;
#128119=CARTESIAN_POINT ( 'NONE',  ( 27.99999999999996803, -49.14999999999999147, 49.92499999999997584 ) ) ;
#128120=( BOUNDED_CURVE ( )  B_SPLINE_CURVE ( 2, ( #130664, #119728, #31336, #20424, #106718, #108852, #117581, #51665, #53817, #87138, #95144, #139412, #128510 ),
 .UNSPECIFIED., .F., .T. ) 
 B_SPLINE_CURVE_WITH_KNOTS ( ( 3, 2, 2, 2, 2, 2, 3 ),
 ( 0.6000000000000000888, 0.6083333333333333925, 0.6166666666666668073, 0.6250000000000001110, 0.6333333333333334147, 0.6416666666666668295, 0.6500000000000001332 ),
 .UNSPECIFIED. ) 
 CURVE ( )  GEOMETRIC_REPRESENTATION_ITEM ( )  RATIONAL_B_SPLINE_CURVE ( ( 0.9999999999999995559, 0.9659258262890687563, 1.000000000000000000, 0.9659258262890683122, 1.000000000000000000, 0.9659258262890683122, 1.000000000000000000, 0.9659258262890683122, 1.000000000000000000, 0.9659258262890683122, 1.000000000000000000, 0.9659258262890678681, 1.000000000000000444 ) ) 
 REPRESENTATION_ITEM ( '' )  );
#128132=ADVANCED_FACE ( 'NONE', ( #136207 ), #27131, .T. ) ;
#128133=FACE_OUTER_BOUND ( 'NONE', #137135, .T. ) ;
#128136=SURFACE_STYLE_USAGE ( .BOTH. , #93348 ) ;
#128150=CARTESIAN_POINT ( 'NONE',  ( 13.17080628287043886, -3.047499999999997211, -5.278424836066143655 ) ) ;
#128153=CIRCLE ( 'NONE', #65686, 28.00000000000002487 ) ;
#128184=( LENGTH_UNIT ( ) NAMED_UNIT ( * ) SI_UNIT ( .MILLI., .METRE. ) );
#128189=CARTESIAN_POINT ( 'NONE',  ( 7.562069808101886892, -7.934999999999991616, -2.126176841940955242 ) ) ;
#128208=ORIENTED_EDGE ( 'NONE', *, *, #14870, .T. ) ;
#128217=DIRECTION ( 'NONE',  ( -1.000000000000000000, 0.000000000000000000, 0.000000000000000000 ) ) ;
#128228=CARTESIAN_POINT ( 'NONE',  ( 26.66623647476855652, 7.934999999999990727, -1.457635852685135314E-15 ) ) ;
#128229=CARTESIAN_POINT ( 'NONE',  ( 7.562069808101886892, -7.934999999999990727, -2.126176841940955242 ) ) ;
#128231=LINE ( 'NONE', #37661, #25117 ) ;
#128264=SURFACE_STYLE_USAGE ( .BOTH. , #83328 ) ;
#128283=CARTESIAN_POINT ( 'NONE',  ( 12.17123647476855375, 0.000000000000000000, 7.934999999999990727 ) ) ;
#128289=EDGE_CURVE ( 'NONE', #52479, #115565, #11715, .T. ) ;
#128342=ORIENTED_EDGE ( 'NONE', *, *, #18839, .T. ) ;
#128358=CARTESIAN_POINT ( 'NONE',  ( 12.90040314143522160, -7.934999999999989839, 2.126176841940957907 ) ) ;
#128370=CARTESIAN_POINT ( 'NONE',  ( 184.1173099067128192, -47.89015928895675955, -37.22465919495432729 ) ) ;
#128421=CARTESIAN_POINT ( 'NONE',  ( 151.4000000000000057, -18.48000000000005372, 34.92499999999998295 ) ) ;
#128437=MECHANICAL_DESIGN_GEOMETRIC_PRESENTATION_REPRESENTATION('',(#28868),#121473);
#128444=SURFACE_STYLE_FILL_AREA ( #106645 ) ;
#128461=CARTESIAN_POINT ( 'NONE',  ( 128.5894344200537773, -49.14999999999999147, -39.86617647058817226 ) ) ;
#128486=FILL_AREA_STYLE_COLOUR ( '', #11011 ) ;
#128499=ORIENTED_EDGE ( 'NONE', *, *, #138395, .T. ) ;
#128510=CARTESIAN_POINT ( 'NONE',  ( 20.46247294953710849, -7.464222240803106570E-16, -6.094999999999989981 ) ) ;
#128518=DIRECTION ( 'NONE',  ( -0.7071067811865487940, 8.659560562354918067E-17, -0.7071067811865463515 ) ) ;
#128524=CARTESIAN_POINT ( 'NONE',  ( 10.27540314143522160, -2.126176841940958351, -7.934999999999989839 ) ) ;
#128552=CARTESIAN_POINT ( 'NONE',  ( 14.70790314143522082, -6.871911579029513106, -3.967499999999993587 ) ) ;
#128557=FACE_OUTER_BOUND ( 'NONE', #138070, .T. ) ;
#128560=CARTESIAN_POINT ( 'NONE',  ( 2.999999999999999112, -4.599999999999996980, -17.44999999999995310 ) ) ;
#128592=AXIS2_PLACEMENT_3D ( 'NONE', #59295, #114346, #103450 ) ;
#128607=FILL_AREA_STYLE ('',( #71378 ) ) ;
#128636=ORIENTED_EDGE ( 'NONE', *, *, #99577, .F. ) ;
#128644=PLANE ( 'NONE',  #58263 ) ;
#128681=CARTESIAN_POINT ( 'NONE',  ( 19.14997294953710849, -4.461849672132299105, 4.461849672132299993 ) ) ;
#128693=ORIENTED_EDGE ( 'NONE', *, *, #28806, .F. ) ;
#128700=ORIENTED_EDGE ( 'NONE', *, *, #67653, .T. ) ;
#128733=ORIENTED_EDGE ( 'NONE', *, *, #126945, .F. ) ;
#128756=CARTESIAN_POINT ( 'NONE',  ( 33.25000000000000000, -7.464222240803106570E-16, -6.094999999999989981 ) ) ;
#128776=CARTESIAN_POINT ( 'NONE',  ( 13.41666666666666785, 5.278424836066147208, 3.047499999999990550 ) ) ;
#128778=CARTESIAN_POINT ( 'NONE',  ( 2.000000000000256239, -6.019044215166783118, 0.9592349742722835471 ) ) ;
#128802=CARTESIAN_POINT ( 'NONE',  ( 180.4193221990230143, -49.14999999999999147, 40.92499999999998295 ) ) ;
#128805=FACE_OUTER_BOUND ( 'NONE', #15015, .T. ) ;
#128818=CARTESIAN_POINT ( 'NONE',  ( 180.8518557880187529, -48.98056306480232536, 39.49745726092412212 ) ) ;
#128858=ORIENTED_EDGE ( 'NONE', *, *, #85776, .T. ) ;
#128868=CARTESIAN_POINT ( 'NONE',  ( 0.3252437201521669041, -48.93522302958528769, 39.28544916627436123 ) ) ;
#128871=CARTESIAN_POINT ( 'NONE',  ( 2.020403141435219485, 7.934999999999989839, -2.126176841940961904 ) ) ;
#128902=UNCERTAINTY_MEASURE_WITH_UNIT (LENGTH_MEASURE( 1.000000000000000082E-05 ), #122294, 'distance_accuracy_value', 'NONE');
#128908=( GEOMETRIC_REPRESENTATION_CONTEXT ( 3 ) GLOBAL_UNCERTAINTY_ASSIGNED_CONTEXT ( ( #115512 ) ) GLOBAL_UNIT_ASSIGNED_CONTEXT ( ( #87579, #21612, #11399 ) ) REPRESENTATION_CONTEXT ( 'NONE', 'WORKASPACE' ) );
#128920=CARTESIAN_POINT ( 'NONE',  ( 1.604166666666666297, -1.633150327867691987, -6.094999999999989093 ) ) ;
#128921=CARTESIAN_POINT ( 'NONE',  ( 9.166236474768552966, 7.934999999999990727, -1.457635852685135314E-15 ) ) ;
#128958=CARTESIAN_POINT ( 'NONE',  ( 128.0580420323229873, -46.73296206246176610, 36.09967824800666136 ) ) ;
#128977=CARTESIAN_POINT ( 'NONE',  ( 181.1500000000000057, -43.14999999999999147, -34.92499999999998295 ) ) ;
#128978=CARTESIAN_POINT ( 'NONE',  ( 6.629569808101885897, -3.967499999999998028, -6.871911579029511330 ) ) ;
#128979=CARTESIAN_POINT ( 'NONE',  ( 22.60416666666666785, -1.633150327867672447, -6.094999999999999751 ) ) ;
#129002=EDGE_CURVE ( 'NONE', #49688, #140587, #138024, .T. ) ;
#129044=CARTESIAN_POINT ( 'NONE',  ( 12.02540314143521982, 2.126176841940962348, 7.934999999999989839 ) ) ;
#129095=ORIENTED_EDGE ( 'NONE', *, *, #38407, .F. ) ;
#129207=FILL_AREA_STYLE ('',( #83604 ) ) ;
#129208=CARTESIAN_POINT ( 'NONE',  ( 20.62956980810188412, -3.967499999999998028, -6.871911579029511330 ) ) ;
#129240=CARTESIAN_POINT ( 'NONE',  ( 12.22873647476855119, 5.808823158059031044, -5.808823158059038150 ) ) ;
#129243=CARTESIAN_POINT ( 'NONE',  ( 0.8183591370940056509, -52.14999999999999147, 41.64499999999997470 ) ) ;
#129244=ORIENTED_EDGE ( 'NONE', *, *, #111916, .F. ) ;
#129266=EDGE_CURVE ( 'NONE', #127303, #16103, #31803, .T. ) ;
#129278=EDGE_CURVE ( 'NONE', #106598, #89590, #58867, .T. ) ;
#129280=ORIENTED_EDGE ( 'NONE', *, *, #83119, .F. ) ;
#129299=( NAMED_UNIT ( * ) SI_UNIT ( $, .STERADIAN. ) SOLID_ANGLE_UNIT ( ) );
#129311=( GEOMETRIC_REPRESENTATION_CONTEXT ( 3 ) GLOBAL_UNCERTAINTY_ASSIGNED_CONTEXT ( ( #36029 ) ) GLOBAL_UNIT_ASSIGNED_CONTEXT ( ( #89960, #68970, #137059 ) ) REPRESENTATION_CONTEXT ( 'NONE', 'WORKASPACE' ) );
#129378=CARTESIAN_POINT ( 'NONE',  ( 26.14997294953710139, -4.461849672132299105, 4.461849672132299993 ) ) ;
#129403=COLOUR_RGB ( '', 0.08235294, 0.09019608, 0.10196078) ;
#129415=CARTESIAN_POINT ( 'NONE',  ( 29.87456980810189222, 6.871911579029510442, -3.967499999999998916 ) ) ;
#129428=CARTESIAN_POINT ( 'NONE',  ( 0.6130698085681498544, -49.19053253528764458, -40.77637019027829979 ) ) ;
#129432=COLOUR_RGB ( '', 0.66274510, 0.83137255, 0.94901961) ;
#129436=ORIENTED_EDGE ( 'NONE', *, *, #22688, .T. ) ;
#129464=CARTESIAN_POINT ( 'NONE',  ( 34.27083333333333570, 6.094999999999991758, 1.633150327867687102 ) ) ;
#129505=CARTESIAN_POINT ( 'NONE',  ( 180.9587832221920110, -48.83231052142031814, 38.98973348322100918 ) ) ;
#129507=FILL_AREA_STYLE_COLOUR ( '', #37421 ) ;
#129519=CARTESIAN_POINT ( 'NONE',  ( 183.6085471140771403, -52.10163751122425424, 40.43817685074128576 ) ) ;
#129575=CARTESIAN_POINT ( 'NONE',  ( 0.000000000000000000, -14.29000000000013593, -12.70000000000045404 ) ) ;
#129578=CARTESIAN_POINT ( 'NONE',  ( 5.666236474768552078, 7.934999999999990727, -1.457635852685135314E-15 ) ) ;
#129609=CARTESIAN_POINT ( 'NONE',  ( 56.62524208092768419, -47.99115898044231443, -37.22402166429051817 ) ) ;
#129624=CARTESIAN_POINT ( 'NONE',  ( 4.375000000000000000, -6.094999999999989981, 3.732111120401553285E-16 ) ) ;
#129625=CARTESIAN_POINT ( 'NONE',  ( 15.29123647476855297, -9.717572351234235426E-16, -7.934999999999990727 ) ) ;
#129630=ORIENTED_EDGE ( 'NONE', *, *, #93280, .F. ) ;
#129632=VECTOR ( 'NONE', #26442, 1000.000000000000000 ) ;
#129639=FACE_OUTER_BOUND ( 'NONE', #73221, .T. ) ;
#129650=CARTESIAN_POINT ( 'NONE',  ( 2.999999999999999112, -1.600000000000055600, -28.92500000000001492 ) ) ;
#129652=( LENGTH_UNIT ( ) NAMED_UNIT ( * ) SI_UNIT ( .MILLI., .METRE. ) );
#129662=CARTESIAN_POINT ( 'NONE',  ( 127.0485559394950457, -49.69743550128772824, 36.79359617903031676 ) ) ;
#129665=ORIENTED_EDGE ( 'NONE', *, *, #34650, .F. ) ;
#129667=DIRECTION ( 'NONE',  ( 0.000000000000000000, -1.000000000000000000, -1.286409696682840916E-16 ) ) ;
#129683=CARTESIAN_POINT ( 'NONE',  ( 20.19206980810188767, -7.934999999999990727, -2.126176841940955242 ) ) ;
#129684=CARTESIAN_POINT ( 'NONE',  ( 22.75000000000000355, -7.464222240803106570E-16, -6.094999999999989981 ) ) ;
#129692=STYLED_ITEM ( 'NONE', ( #16450 ), #116432 ) ;
#129702=COLOUR_RGB ( '', 0.40784314, 0.44705882, 0.49803922) ;
#129707=FACE_OUTER_BOUND ( 'NONE', #57384, .T. ) ;
#129710=CARTESIAN_POINT ( 'NONE',  ( 25.40000000000000568, 3.273809073538042291, -7.239615486481085327 ) ) ;
#129752=AXIS2_PLACEMENT_3D ( 'NONE', #1203, #88251, #119410 ) ;
#129760=CARTESIAN_POINT ( 'NONE',  ( 14.21290314143522160, 3.967499999999992699, -6.871911579029513994 ) ) ;
#129775=CARTESIAN_POINT ( 'NONE',  ( 184.1499999999998067, -47.62213595499957819, -36.92499999999998295 ) ) ;
#129776=ORIENTED_EDGE ( 'NONE', *, *, #93032, .F. ) ;
#129793=FACE_OUTER_BOUND ( 'NONE', #18470, .T. ) ;
#129799=CARTESIAN_POINT ( 'NONE',  ( 0.1600000000000005862, -5.232655156125630924, -5.974607078898705126 ) ) ;
#129823=( GEOMETRIC_REPRESENTATION_CONTEXT ( 3 ) GLOBAL_UNCERTAINTY_ASSIGNED_CONTEXT ( ( #22943 ) ) GLOBAL_UNIT_ASSIGNED_CONTEXT ( ( #114451, #15120, #23897 ) ) REPRESENTATION_CONTEXT ( 'NONE', 'WORKASPACE' ) );
#129828=MECHANICAL_DESIGN_GEOMETRIC_PRESENTATION_REPRESENTATION('',(#9438),#122895);
#129874=CARTESIAN_POINT ( 'NONE',  ( 152.4000000000000057, 25.96999999999993847, 0.000000000000000000 ) ) ;
#129891=DIRECTION ( 'NONE',  ( 0.000000000000000000, 0.000000000000000000, 1.000000000000000000 ) ) ;
#129906=VERTEX_POINT ( 'NONE', #133080 ) ;
#129945=CARTESIAN_POINT ( 'NONE',  ( 22.96290314143522338, -3.967499999999994476, 6.871911579029513106 ) ) ;
#129953=DIRECTION ( 'NONE',  ( 1.000000000000000000, 0.000000000000000000, -0.000000000000000000 ) ) ;
#129978=CARTESIAN_POINT ( 'NONE',  ( 13.54123647476855474, 0.000000000000000000, 7.934999999999990727 ) ) ;
#130006=CARTESIAN_POINT ( 'NONE',  ( 3.000000000000000000, -4.600000000000055600, -28.92500000000000071 ) ) ;
#130022=STYLED_ITEM ( 'NONE', ( #35828 ), #131026 ) ;
#130045=CARTESIAN_POINT ( 'NONE',  ( 9.670806282870438864, -3.047499999999997211, -5.278424836066143655 ) ) ;
#130054=ORIENTED_EDGE ( 'NONE', *, *, #11053, .T. ) ;
#130108=( LENGTH_UNIT ( ) NAMED_UNIT ( * ) SI_UNIT ( .MILLI., .METRE. ) );
#130112=ORIENTED_EDGE ( 'NONE', *, *, #71815, .F. ) ;
#130121=CARTESIAN_POINT ( 'NONE',  ( 25.56663961620377634, 1.633150327867695095, 6.094999999999988205 ) ) ;
#130141=CARTESIAN_POINT ( 'NONE',  ( 156.1499999999997783, -57.14999999999999147, -34.92499999999975557 ) ) ;
#130143=ORIENTED_EDGE ( 'NONE', *, *, #21656, .F. ) ;
#130160=CARTESIAN_POINT ( 'NONE',  ( 33.81206980810188156, 7.934999999999993392, 2.126176841940951689 ) ) ;
#130166=CARTESIAN_POINT ( 'NONE',  ( 52.51281677483339649, -49.11905619111360721, 40.21880474160332142 ) ) ;
#130207=CARTESIAN_POINT ( 'NONE',  ( 33.54166666666667140, 3.047499999999993214, -5.278424836066146320 ) ) ;
#130227=CARTESIAN_POINT ( 'NONE',  ( 128.7663314791150242, -49.19090614205754974, -40.79110616923124866 ) ) ;
#130247=VECTOR ( 'NONE', #10462, 1000.000000000000000 ) ;
#130273=PRESENTATION_STYLE_ASSIGNMENT (( #87473 ) ) ;
#130295=EDGE_CURVE ( 'NONE', #60012, #106911, #63378, .T. ) ;
#130313=LINE ( 'NONE', #73085, #28968 ) ;
#130327=CARTESIAN_POINT ( 'NONE',  ( 2.312069808101886448, 7.934999999999993392, 2.126176841940951689 ) ) ;
#130354=ORIENTED_EDGE ( 'NONE', *, *, #43473, .F. ) ;
#130371=CARTESIAN_POINT ( 'NONE',  ( 7.145833333333333925, -1.633150327867689988, 6.094999999999989981 ) ) ;
#130372=CARTESIAN_POINT ( 'NONE',  ( 16.74956980810188867, 3.967499999999998916, 6.871911579029510442 ) ) ;
#130391=CARTESIAN_POINT ( 'NONE',  ( 0.2535635638417512716, -51.76057561339555946, 38.69631370864701836 ) ) ;
#130395=DIRECTION ( 'NONE',  ( -1.000000000000000000, -0.000000000000000000, -0.000000000000000000 ) ) ;
#130420=AXIS2_PLACEMENT_3D ( 'NONE', #38776, #59826, #60563 ) ;
#130428=CARTESIAN_POINT ( 'NONE',  ( 19.60873647476855197, -5.808823158059033709, 5.808823158059035485 ) ) ;
#130443=CARTESIAN_POINT ( 'NONE',  ( 18.37500000000000355, -6.094999999999989981, 3.732111120401553285E-16 ) ) ;
#130471=DIRECTION ( 'NONE',  ( 0.000000000000000000, -0.000000000000000000, -1.000000000000000000 ) ) ;
#130484=VERTEX_POINT ( 'NONE', #25532 ) ;
#130504=CARTESIAN_POINT ( 'NONE',  ( 9.254569808101885897, -6.871911579029512218, 3.967499999999996252 ) ) ;
#130518=CARTESIAN_POINT ( 'NONE',  ( 184.0821179325846515, -51.13011358081446645, -36.94363806876467748 ) ) ;
#130524=ORIENTED_EDGE ( 'NONE', *, *, #80551, .F. ) ;
#130592=CARTESIAN_POINT ( 'NONE',  ( 149.2199999999997999, -3.180000000000061444, 31.92499999999998295 ) ) ;
#130614=( NAMED_UNIT ( * ) SI_UNIT ( $, .STERADIAN. ) SOLID_ANGLE_UNIT ( ) );
#130618=( BOUNDED_SURFACE ( )  B_SPLINE_SURFACE ( 3, 2, ( 
 ( #135882, #36562, #28563 ),
 ( #27107, #80805, #37288 ),
 ( #81536, #26416, #53898 ),
 ( #40853, #96610, #140852 ) ),
 .UNSPECIFIED., .F., .F., .F. ) 
 B_SPLINE_SURFACE_WITH_KNOTS ( ( 4, 4 ),
 ( 3, 3 ),
 ( 0.000000000000000000, 0.001630001914283312967 ),
 ( 0.000000000000000000, 1.000000000000000000 ),
 .UNSPECIFIED. ) 
 GEOMETRIC_REPRESENTATION_ITEM ( )  RATIONAL_B_SPLINE_SURFACE ( (
 ( 1.000000000000000000, 0.7180326832784529323, 1.000000000000000000),
 ( 1.000000000000000000, 0.7157206429707735351, 1.000000000000000000),
 ( 1.000000000000000000, 0.7121002461815040263, 1.000000000000000000),
 ( 1.000000000000000000, 0.7071067811865475727, 1.000000000000000000) ) ) 
 REPRESENTATION_ITEM ( '' )  SURFACE ( )  );
#130626=CIRCLE ( 'NONE', #127736, 1.000000000000000888 ) ;
#130635=ADVANCED_FACE ( 'NONE', ( #137893 ), #82109, .F. ) ;
#130642=DIRECTION ( 'NONE',  ( 1.000000000000000000, 0.000000000000000000, 0.000000000000000000 ) ) ;
#130664=CARTESIAN_POINT ( 'NONE',  ( 18.71247294953710494, 0.000000000000000000, 6.094999999999989981 ) ) ;
#130679=CARTESIAN_POINT ( 'NONE',  ( 16.69206980810189123, -7.934999999999991616, -2.126176841940955242 ) ) ;
#130692=CARTESIAN_POINT ( 'NONE',  ( 152.4000000000000057, -16.48000000000005016, -12.70000000000045404 ) ) ;
#130706=CARTESIAN_POINT ( 'NONE',  ( 5.250000000000000000, -7.464222240803106570E-16, -6.094999999999989981 ) ) ;
#130717=( GEOMETRIC_REPRESENTATION_CONTEXT ( 3 ) GLOBAL_UNCERTAINTY_ASSIGNED_CONTEXT ( ( #76682 ) ) GLOBAL_UNIT_ASSIGNED_CONTEXT ( ( #58354, #124261, #89488 ) ) REPRESENTATION_CONTEXT ( 'NONE', 'WORKASPACE' ) );
#130721=CARTESIAN_POINT ( 'NONE',  ( 152.4000000000000057, 7.919999999999947526, 19.12499999999998224 ) ) ;
#130747=FILL_AREA_STYLE_COLOUR ( '', #93060 ) ;
#130785=CARTESIAN_POINT ( 'NONE',  ( 7.000000000000000888, 0.000000000000000000, 6.094999999999989981 ) ) ;
#130832=DIRECTION ( 'NONE',  ( -0.1737853339090456306, -0.1737853339090452420, 0.9693282805305142302 ) ) ;
#130842=LINE ( 'NONE', #109040, #97608 ) ;
#130852=CARTESIAN_POINT ( 'NONE',  ( 22.79580628287044064, -5.278424836066144543, 3.047499999999995879 ) ) ;
#130877=CARTESIAN_POINT ( 'NONE',  ( 27.99999999999996803, -49.14999999999999147, 49.92499999999997584 ) ) ;
#130925=CARTESIAN_POINT ( 'NONE',  ( 25.39999999999999858, 1.126161369193132478, 16.41140641659140798 ) ) ;
#130931=CARTESIAN_POINT ( 'NONE',  ( 28.87500000000000000, -6.094999999999989981, 3.732111120401553285E-16 ) ) ;
#130938=SURFACE_SIDE_STYLE ('',( #42506 ) ) ;
#130940=ORIENTED_EDGE ( 'NONE', *, *, #57603, .T. ) ;
#130948=ORIENTED_EDGE ( 'NONE', *, *, #116370, .T. ) ;
#130949=CARTESIAN_POINT ( 'NONE',  ( 131.6371832251712135, -49.11905619111362142, -40.21880474160340668 ) ) ;
#130987=CARTESIAN_POINT ( 'NONE',  ( 181.1500000013235478, -47.86718710719740244, 37.19897551713948047 ) ) ;
#131026=ADVANCED_FACE ( 'NONE', ( #78590 ), #54708, .F. ) ;
#131032=CARTESIAN_POINT ( 'NONE',  ( 14.70790314143522082, -6.871911579029513106, -3.967499999999993587 ) ) ;
#131040=CARTESIAN_POINT ( 'NONE',  ( 19.25000000000000355, -7.464222240803106570E-16, -6.094999999999989981 ) ) ;
#131072=CARTESIAN_POINT ( 'NONE',  ( 0.8750000000000001110, -6.094999999999989981, 3.732111120401553285E-16 ) ) ;
#131073=CARTESIAN_POINT ( 'NONE',  ( 20.24956980810188867, 3.967499999999998916, 6.871911579029510442 ) ) ;
#131086=CARTESIAN_POINT ( 'NONE',  ( 128.5279624519184836, -51.91654526992326879, -39.52330221398023014 ) ) ;
#131113=CARTESIAN_POINT ( 'NONE',  ( 125.6094186379952049, -46.07581969935596078, 35.63601533997828597 ) ) ;
#131129=CARTESIAN_POINT ( 'NONE',  ( 17.85873647476855197, 5.808823158059031044, -5.808823158059037262 ) ) ;
#131132=CARTESIAN_POINT ( 'NONE',  ( 166.7105211023042841, 26.96999999999993491, 32.60830646801873201 ) ) ;
#131137=ORIENTED_EDGE ( 'NONE', *, *, #143348, .F. ) ;
#131146=DIRECTION ( 'NONE',  ( 1.000000000000000000, 0.000000000000000000, -0.000000000000000000 ) ) ;
#131164=DIRECTION ( 'NONE',  ( 0.000000000000000000, -1.000000000000000000, 0.000000000000000000 ) ) ;
#131194=ADVANCED_FACE ( 'NONE', ( #138694 ), #105320, .T. ) ;
#131197=CARTESIAN_POINT ( 'NONE',  ( 20.77540314143522338, -2.126176841940958351, -7.934999999999989839 ) ) ;
#131202=CARTESIAN_POINT ( 'NONE',  ( 55.18164086290597226, -52.14999999999999147, -41.64500000000000313 ) ) ;
#131211=CARTESIAN_POINT ( 'NONE',  ( 181.1499999999998067, -47.62213595499956398, -36.92499999999996163 ) ) ;
#131229=LINE ( 'NONE', #74735, #37319 ) ;
#131238=SURFACE_STYLE_FILL_AREA ( #97902 ) ;
#131246=ORIENTED_EDGE ( 'NONE', *, *, #80816, .T. ) ;
#131310=EDGE_LOOP ( 'NONE', ( #54075, #28379, #44783, #127505 ) ) ;
#131331=ORIENTED_EDGE ( 'NONE', *, *, #142429, .T. ) ;
#131341=ORIENTED_EDGE ( 'NONE', *, *, #118575, .T. ) ;
#131364=EDGE_CURVE ( 'NONE', #61426, #141239, #95336, .T. ) ;
#131371=CARTESIAN_POINT ( 'NONE',  ( 19.46290314143521982, -3.967499999999994476, 6.871911579029513106 ) ) ;
#131377=STYLED_ITEM ( 'NONE', ( #27475 ), #4147 ) ;
#131410=STYLED_ITEM ( 'NONE', ( #119016 ), #137587 ) ;
#131440=CARTESIAN_POINT ( 'NONE',  ( 152.4000000000000057, 7.919999999999947526, -18.97500000000001918 ) ) ;
#131478=SURFACE_STYLE_FILL_AREA ( #42345 ) ;
#131527=FILL_AREA_STYLE_COLOUR ( '', #127902 ) ;
#131535=( GEOMETRIC_REPRESENTATION_CONTEXT ( 3 ) GLOBAL_UNCERTAINTY_ASSIGNED_CONTEXT ( ( #69193 ) ) GLOBAL_UNIT_ASSIGNED_CONTEXT ( ( #102998, #60223, #137051 ) ) REPRESENTATION_CONTEXT ( 'NONE', 'WORKASPACE' ) );
#131540=CARTESIAN_POINT ( 'NONE',  ( 22.94163961620376568, -6.094999999999989093, 1.633150327867691765 ) ) ;
#131571=EDGE_CURVE ( 'NONE', #116882, #77069, #16577, .T. ) ;
#131586=CARTESIAN_POINT ( 'NONE',  ( 52.40027281129884784, -49.14999999999999147, 40.57187971031920171 ) ) ;
#131625=ORIENTED_EDGE ( 'NONE', *, *, #58049, .T. ) ;
#131638=AXIS2_PLACEMENT_3D ( 'NONE', #90603, #55846, #47154 ) ;
#131678=CARTESIAN_POINT ( 'NONE',  ( 181.1391930515558215, -48.09618305010690875, 37.50858089739960377 ) ) ;
#131681=CARTESIAN_POINT ( 'NONE',  ( 184.1500000000000057, -57.15000000000003411, -15.92500000000064730 ) ) ;
#131710=ORIENTED_EDGE ( 'NONE', *, *, #51179, .T. ) ;
#131749=CARTESIAN_POINT ( 'NONE',  ( 16.45790314143522082, 6.871911579029515771, 3.967499999999989146 ) ) ;
#131758=UNCERTAINTY_MEASURE_WITH_UNIT (LENGTH_MEASURE( 1.000000000000000082E-05 ), #50087, 'distance_accuracy_value', 'NONE');
#131773=CARTESIAN_POINT ( 'NONE',  ( 18.71247294953710494, 0.000000000000000000, 6.094999999999989981 ) ) ;
#131787=CYLINDRICAL_SURFACE ( 'NONE', #27384, 3.000000000000002665 ) ;
#131791=CARTESIAN_POINT ( 'NONE',  ( 5.250000000000000000, -7.464222240803106570E-16, -6.094999999999989981 ) ) ;
#131792=CARTESIAN_POINT ( 'NONE',  ( 16.60373647476855297, 5.808823158059035485, 5.808823158059032821 ) ) ;
#131802=CARTESIAN_POINT ( 'NONE',  ( 131.5423521607622774, -49.05583548141699168, -39.86617647058817226 ) ) ;
#131807=PRESENTATION_STYLE_ASSIGNMENT (( #28397 ) ) ;
#131813=SURFACE_STYLE_FILL_AREA ( #107184 ) ;
#131823=ORIENTED_EDGE ( 'NONE', *, *, #96957, .F. ) ;
#131827=CARTESIAN_POINT ( 'NONE',  ( 128.6786164994711044, -49.14501756083436845, 40.36361034346624876 ) ) ;
#131832=CARTESIAN_POINT ( 'NONE',  ( 183.3316408629058287, -52.14999999999999147, 41.64499999999997470 ) ) ;
#131834=STYLED_ITEM ( 'NONE', ( #14662 ), #96714 ) ;
#131853=CARTESIAN_POINT ( 'NONE',  ( 166.8257598198775895, 26.96999999999993847, 32.27759070793130292 ) ) ;
#131876=SURFACE_STYLE_USAGE ( .BOTH. , #87649 ) ;
#131877=VERTEX_POINT ( 'NONE', #69533 ) ;
#131887=SURFACE_STYLE_USAGE ( .BOTH. , #141319 ) ;
#131900=ORIENTED_EDGE ( 'NONE', *, *, #115152, .F. ) ;
#131911=CARTESIAN_POINT ( 'NONE',  ( 0.000000000000000000, -30.18000000000009564, 15.92499999999935945 ) ) ;
#131917=MECHANICAL_DESIGN_GEOMETRIC_PRESENTATION_REPRESENTATION('',(#57851),#9224);
#131919=( BOUNDED_CURVE ( )  B_SPLINE_CURVE ( 2, ( #112168, #67229, #45503, #21581, #33208, #78828, #77419, #46216, #120870, #123038, #87546, #54241, #131773 ),
 .UNSPECIFIED., .F., .T. ) 
 B_SPLINE_CURVE_WITH_KNOTS ( ( 3, 2, 2, 2, 2, 2, 3 ),
 ( 0.5500000000000001554, 0.5583333333333334592, 0.5666666666666667629, 0.5750000000000000666, 0.5833333333333334814, 0.5916666666666667851, 0.6000000000000000888 ),
 .UNSPECIFIED. ) 
 CURVE ( )  GEOMETRIC_REPRESENTATION_ITEM ( )  RATIONAL_B_SPLINE_CURVE ( ( 0.9999999999999995559, 0.9659258262890687563, 1.000000000000000000, 0.9659258262890683122, 1.000000000000000000, 0.9659258262890683122, 1.000000000000000000, 0.9659258262890683122, 1.000000000000000000, 0.9659258262890683122, 1.000000000000000000, 0.9659258262890678681, 1.000000000000000444 ) ) 
 REPRESENTATION_ITEM ( '' )  );
#131922=CARTESIAN_POINT ( 'NONE',  ( 16.25456980810188767, -6.871911579029512218, 3.967499999999996252 ) ) ;
#131937=DIRECTION ( 'NONE',  ( 0.000000000000000000, 0.000000000000000000, 1.000000000000000000 ) ) ;
#131943=AXIS2_PLACEMENT_3D ( 'NONE', #73344, #139328, #109335 ) ;
#131951=VECTOR ( 'NONE', #40169, 1000.000000000000000 ) ;
#131959=AXIS2_PLACEMENT_3D ( 'NONE', #52442, #11054, #57482 ) ;
#131985=CARTESIAN_POINT ( 'NONE',  ( 128.5894344200537489, -57.14999999999999147, 39.86617647058822911 ) ) ;
#131986=VECTOR ( 'NONE', #128518, 1000.000000000000000 ) ;
#131989=( NAMED_UNIT ( * ) SI_UNIT ( $, .STERADIAN. ) SOLID_ANGLE_UNIT ( ) );
#132020=DIRECTION ( 'NONE',  ( 1.000000000000000000, 0.000000000000000000, -0.000000000000000000 ) ) ;
#132048=SURFACE_STYLE_FILL_AREA ( #100827 ) ;
#132087=DIRECTION ( 'NONE',  ( 0.9707728879609287542, 0.000000000000000000, -0.2399999999999954392 ) ) ;
#132100=CARTESIAN_POINT ( 'NONE',  ( 19.90040314143521982, -7.934999999999989839, 2.126176841940957907 ) ) ;
#132131=EDGE_LOOP ( 'NONE', ( #66271, #77541, #315, #25799 ) ) ;
#132167=CYLINDRICAL_SURFACE ( 'NONE', #141740, 2.552699999999959779 ) ;
#132189=CARTESIAN_POINT ( 'NONE',  ( 0.1600000000000026401, -9.717572351234235426E-16, -7.934999999999990727 ) ) ;
#132191=ORIENTED_EDGE ( 'NONE', *, *, #123542, .T. ) ;
#132207=DIRECTION ( 'NONE',  ( -1.000000000000000000, -0.000000000000000000, 0.000000000000000000 ) ) ;
#132256=EDGE_CURVE ( 'NONE', #8597, #137404, #81790, .T. ) ;
#132268=EDGE_CURVE ( 'NONE', #71833, #8723, #126219, .T. ) ;
#132286=CARTESIAN_POINT ( 'NONE',  ( 27.75413961620377279, 3.047499999999993214, -5.278424836066146320 ) ) ;
#132292=AXIS2_PLACEMENT_3D ( 'NONE', #115710, #94693, #62109 ) ;
#132313=ORIENTED_EDGE ( 'NONE', *, *, #34017, .T. ) ;
#132328=DIRECTION ( 'NONE',  ( -0.000000000000000000, -1.000000000000000000, -0.000000000000000000 ) ) ;
#132329=( LENGTH_UNIT ( ) NAMED_UNIT ( * ) SI_UNIT ( .MILLI., .METRE. ) );
#132340=CARTESIAN_POINT ( 'NONE',  ( 153.4000000000000057, 26.96999999999993847, 34.92499999999998295 ) ) ;
#132355=ORIENTED_EDGE ( 'NONE', *, *, #112591, .T. ) ;
#132378=( NAMED_UNIT ( * ) SI_UNIT ( $, .STERADIAN. ) SOLID_ANGLE_UNIT ( ) );
#132384=DIRECTION ( 'NONE',  ( 0.000000000000000000, 0.000000000000000000, 1.000000000000000000 ) ) ;
#132442=AXIS2_PLACEMENT_3D ( 'NONE', #73084, #117237, #17916 ) ;
#132466=CARTESIAN_POINT ( 'NONE',  ( -0.1000270504628942014, 4.461849672132297329, -4.461849672132302658 ) ) ;
#132475=AXIS2_PLACEMENT_3D ( 'NONE', #57725, #23646, #136677 ) ;
#132477=ORIENTED_EDGE ( 'NONE', *, *, #97475, .T. ) ;
#132494=CARTESIAN_POINT ( 'NONE',  ( 12.22873647476855119, 5.808823158059031044, -5.808823158059038150 ) ) ;
#132500=ORIENTED_EDGE ( 'NONE', *, *, #107412, .F. ) ;
#132521=CARTESIAN_POINT ( 'NONE',  ( 152.4000000000000057, 7.919999999999947526, -18.97500000000001918 ) ) ;
#132538=CARTESIAN_POINT ( 'NONE',  ( 15.89583333333333393, 1.633150327867687324, -6.094999999999991758 ) ) ;
#132539=CARTESIAN_POINT ( 'NONE',  ( 16.45790314143522082, 6.871911579029515771, 3.967499999999989146 ) ) ;
#132547=AXIS2_PLACEMENT_3D ( 'NONE', #138871, #70077, #37405 ) ;
#132554=CARTESIAN_POINT ( 'NONE',  ( 128.6723146205780779, -49.13871568196854867, -40.16438383193010964 ) ) ;
#132665=CARTESIAN_POINT ( 'NONE',  ( 22.67123647476855552, 0.000000000000000000, 7.934999999999990727 ) ) ;
#132682=( NAMED_UNIT ( * ) SI_UNIT ( $, .STERADIAN. ) SOLID_ANGLE_UNIT ( ) );
#132700=CARTESIAN_POINT ( 'NONE',  ( 25.39999999999999858, -1.600000000000086020, -34.92499999999998295 ) ) ;
#132709=CARTESIAN_POINT ( 'NONE',  ( 16.31206980810189222, 7.934999999999993392, 2.126176841940951689 ) ) ;
#132757=CIRCLE ( 'NONE', #70264, 2.000000000000001776 ) ;
#132776=DIRECTION ( 'NONE',  ( -1.000000000000000000, 0.000000000000000000, 0.000000000000000000 ) ) ;
#132809=CARTESIAN_POINT ( 'NONE',  ( 152.4000000000000057, 7.919999999999947526, 21.67769999999997310 ) ) ;
#132827=DIRECTION ( 'NONE',  ( -0.000000000000000000, 1.000000000000000000, 0.000000000000000000 ) ) ;
#132828=CARTESIAN_POINT ( 'NONE',  ( 29.37956980810188412, 3.967499999999998916, 6.871911579029510442 ) ) ;
#132885=CARTESIAN_POINT ( 'NONE',  ( 130.7379471109758526, -48.51956544822608208, 36.87500513592861040 ) ) ;
#132948=( NAMED_UNIT ( * ) PLANE_ANGLE_UNIT ( ) SI_UNIT ( $, .RADIAN. ) );
#132958=DIRECTION ( 'NONE',  ( -0.000000000000000000, 1.000000000000000000, -0.000000000000000000 ) ) ;
#132965=ORIENTED_EDGE ( 'NONE', *, *, #51233, .F. ) ;
#132969=VERTEX_POINT ( 'NONE', #98580 ) ;
#132984=ORIENTED_EDGE ( 'NONE', *, *, #115152, .T. ) ;
#132990=VERTEX_POINT ( 'NONE', #55824 ) ;
#132995=CARTESIAN_POINT ( 'NONE',  ( 122.6835989386367771, -43.14999999999999147, -34.92499999999998295 ) ) ;
#132999=CARTESIAN_POINT ( 'NONE',  ( 31.25413961620377634, 3.047499999999993214, -5.278424836066146320 ) ) ;
#133028=LINE ( 'NONE', #67035, #66476 ) ;
#133029=CARTESIAN_POINT ( 'NONE',  ( 128.9683591370938416, -52.14999999999999147, -41.64500000000001023 ) ) ;
#133041=PRESENTATION_STYLE_ASSIGNMENT (( #44621 ) ) ;
#133044=AXIS2_PLACEMENT_3D ( 'NONE', #30433, #121694, #74667 ) ;
#133057=SURFACE_STYLE_FILL_AREA ( #43179 ) ;
#133064=UNCERTAINTY_MEASURE_WITH_UNIT (LENGTH_MEASURE( 1.000000000000000082E-05 ), #114168, 'distance_accuracy_value', 'NONE');
#133080=CARTESIAN_POINT ( 'NONE',  ( 27.99999999999996803, -57.14999999999999147, 45.92499999999999005 ) ) ;
#133099=DIRECTION ( 'NONE',  ( -1.000000000000000000, -0.000000000000000000, 0.000000000000000000 ) ) ;
#133126=SURFACE_STYLE_USAGE ( .BOTH. , #121492 ) ;
#133138=CARTESIAN_POINT ( 'NONE',  ( 3.254139616203772345, 3.047499999999993214, -5.278424836066146320 ) ) ;
#133145=DIRECTION ( 'NONE',  ( -1.000000000000000000, 0.000000000000000000, 0.000000000000000000 ) ) ;
#133161=CARTESIAN_POINT ( 'NONE',  ( 1.649972949537105604, -4.461849672132299105, 4.461849672132299993 ) ) ;
#133190=CARTESIAN_POINT ( 'NONE',  ( 15.29123647476855297, -9.717572351234235426E-16, -7.934999999999990727 ) ) ;
#133202=UNCERTAINTY_MEASURE_WITH_UNIT (LENGTH_MEASURE( 1.000000000000000082E-05 ), #108989, 'distance_accuracy_value', 'NONE');
#133220=FILL_AREA_STYLE_COLOUR ( '', #113435 ) ;
#133229=( BOUNDED_CURVE ( )  B_SPLINE_CURVE ( 3, ( #100889, #134250, #24056, #58151 ),
 .UNSPECIFIED., .F., .T. ) 
 B_SPLINE_CURVE_WITH_KNOTS ( ( 4, 4 ),
 ( 4.712388980384689674, 6.105785702739217058 ),
 .UNSPECIFIED. ) 
 CURVE ( )  GEOMETRIC_REPRESENTATION_ITEM ( )  RATIONAL_B_SPLINE_CURVE ( ( 1.000000000000000000, 0.8446433258982466441, 0.8446433258982466441, 1.000000000000000000 ) ) 
 REPRESENTATION_ITEM ( '' )  );
#133233=SURFACE_STYLE_FILL_AREA ( #110012 ) ;
#133236=CARTESIAN_POINT ( 'NONE',  ( 18.52083333333333570, -6.094999999999989981, -1.633150327867689100 ) ) ;
#133240=ORIENTED_EDGE ( 'NONE', *, *, #96957, .T. ) ;
#133255=SURFACE_SIDE_STYLE ('',( #84234 ) ) ;
#133289=CARTESIAN_POINT ( 'NONE',  ( 21.65040314143522693, 7.934999999999988951, -2.126176841940961904 ) ) ;
#133313=DIRECTION ( 'NONE',  ( -1.000000000000000000, -0.000000000000000000, -0.000000000000000000 ) ) ;
#133330=DIRECTION ( 'NONE',  ( -0.000000000000000000, 1.000000000000000000, 1.286409696682840916E-16 ) ) ;
#133338=ORIENTED_EDGE ( 'NONE', *, *, #104332, .F. ) ;
#133343=CARTESIAN_POINT ( 'NONE',  ( 15.21247294953710671, 0.000000000000000000, 6.094999999999989981 ) ) ;
#133352=CARTESIAN_POINT ( 'NONE',  ( 20.48373647476854842, -5.808823158059035485, -5.808823158059033709 ) ) ;
#133399=CARTESIAN_POINT ( 'NONE',  ( 20.24956980810188867, 3.967499999999998916, 6.871911579029510442 ) ) ;
#133422=CARTESIAN_POINT ( 'NONE',  ( 25.39999999999999858, -1.600000000000094458, 34.92499999999998295 ) ) ;
#133444=CARTESIAN_POINT ( 'NONE',  ( 25.39999999999999858, -57.15000000000003411, -15.92500000000064730 ) ) ;
#133490=( NAMED_UNIT ( * ) SI_UNIT ( $, .STERADIAN. ) SOLID_ANGLE_UNIT ( ) );
#133500=ORIENTED_EDGE ( 'NONE', *, *, #15131, .T. ) ;
#133514=CARTESIAN_POINT ( 'NONE',  ( 29.23373647476855552, 5.808823158059036373, 5.808823158059032821 ) ) ;
#133604=AXIS2_PLACEMENT_3D ( 'NONE', #87947, #77108, #87240 ) ;
#133686=FILL_AREA_STYLE ('',( #89452 ) ) ;
#133688=CARTESIAN_POINT ( 'NONE',  ( -1.828763525231447584, 0.000000000000000000, 7.934999999999990727 ) ) ;
#133699=( LENGTH_UNIT ( ) NAMED_UNIT ( * ) SI_UNIT ( .MILLI., .METRE. ) );
#133709=FILL_AREA_STYLE ('',( #113349 ) ) ;
#133719=EDGE_CURVE ( 'NONE', #143089, #11916, #26893, .T. ) ;
#133722=CARTESIAN_POINT ( 'NONE',  ( 25.39999999999999858, -1.600000000000094458, 34.92499999999998295 ) ) ;
#133732=( NAMED_UNIT ( * ) SI_UNIT ( $, .STERADIAN. ) SOLID_ANGLE_UNIT ( ) );
#133740=( NAMED_UNIT ( * ) PLANE_ANGLE_UNIT ( ) SI_UNIT ( $, .RADIAN. ) );
#133744=EDGE_LOOP ( 'NONE', ( #131331, #106313, #12439, #80715 ) ) ;
#133755=CARTESIAN_POINT ( 'NONE',  ( 16.67080628287043709, -3.047499999999997211, -5.278424836066143655 ) ) ;
#133789=MECHANICAL_DESIGN_GEOMETRIC_PRESENTATION_REPRESENTATION('',(#103637),#82883);
#133811=LINE ( 'NONE', #112763, #80282 ) ;
#133828=CARTESIAN_POINT ( 'NONE',  ( 4.712472949537106715, 0.000000000000000000, 6.094999999999989981 ) ) ;
#133829=COLOUR_RGB ( '', 0.08235294, 0.09019608, 0.10196078) ;
#133837=CARTESIAN_POINT ( 'NONE',  ( 2.087472949537105826, -6.094999999999989981, 3.732111120401553285E-16 ) ) ;
#133850=CARTESIAN_POINT ( 'NONE',  ( 3.837472949537105826, 6.094999999999989981, -1.119633336120465690E-15 ) ) ;
#133882=CARTESIAN_POINT ( 'NONE',  ( 13.10373647476855297, 5.808823158059036373, 5.808823158059032821 ) ) ;
#133883=DIRECTION ( 'NONE',  ( 0.000000000000000000, 0.000000000000000000, 1.000000000000000000 ) ) ;
#133890=CARTESIAN_POINT ( 'NONE',  ( 20.27083333333333570, 6.094999999999991758, 1.633150327867686880 ) ) ;
#133914=SURFACE_SIDE_STYLE ('',( #100581 ) ) ;
#133921=( NAMED_UNIT ( * ) SI_UNIT ( $, .STERADIAN. ) SOLID_ANGLE_UNIT ( ) );
#133927=CARTESIAN_POINT ( 'NONE',  ( 10.79166666666666785, -3.047499999999994547, 5.278424836066145431 ) ) ;
#133928=CARTESIAN_POINT ( 'NONE',  ( 22.72873647476855652, 5.808823158059031044, -5.808823158059037262 ) ) ;
#133948=EDGE_LOOP ( 'NONE', ( #137435, #122375 ) ) ;
#133982=( NAMED_UNIT ( * ) PLANE_ANGLE_UNIT ( ) SI_UNIT ( $, .RADIAN. ) );
#133983=CARTESIAN_POINT ( 'NONE',  ( 25.00456980810188767, 6.871911579029510442, -3.967499999999998916 ) ) ;
#133985=VECTOR ( 'NONE', #18084, 1000.000000000000000 ) ;
#134008=CARTESIAN_POINT ( 'NONE',  ( 128.5894344200537489, -52.00875322212550600, 39.86617647058822911 ) ) ;
#134017=ORIENTED_EDGE ( 'NONE', *, *, #55334, .T. ) ;
#134018=DIRECTION ( 'NONE',  ( -0.000000000000000000, -0.000000000000000000, 1.000000000000000000 ) ) ;
#134042=ORIENTED_EDGE ( 'NONE', *, *, #31591, .F. ) ;
#134062=CARTESIAN_POINT ( 'NONE',  ( 15.08790314143521982, 6.871911579029515771, 3.967499999999989146 ) ) ;
#134093=CARTESIAN_POINT ( 'NONE',  ( 152.4000000000000057, 7.919999999999947526, 16.57230000000002335 ) ) ;
#134095=DIRECTION ( 'NONE',  ( 1.000000000000000000, 0.000000000000000000, 0.000000000000000000 ) ) ;
#134107=CARTESIAN_POINT ( 'NONE',  ( 25.06206980810188512, -7.934999999999991616, -2.126176841940955242 ) ) ;
#134111=CIRCLE ( 'NONE', #69327, 28.00000000000001776 ) ;
#134140=STYLED_ITEM ( 'NONE', ( #135657 ), #57143 ) ;
#134162=CARTESIAN_POINT ( 'NONE',  ( 4.004569808101885897, 6.871911579029510442, -3.967499999999998916 ) ) ;
#134167=EDGE_LOOP ( 'NONE', ( #119400, #100390, #67669 ) ) ;
#134213=LINE ( 'NONE', #79148, #25094 ) ;
#134217=ORIENTED_EDGE ( 'NONE', *, *, #126834, .T. ) ;
#134223=MECHANICAL_DESIGN_GEOMETRIC_PRESENTATION_REPRESENTATION('',(#25110),#64788);
#134233=CARTESIAN_POINT ( 'NONE',  ( 25.00456980810188767, 6.871911579029510442, -3.967499999999998916 ) ) ;
#134245=VERTEX_POINT ( 'NONE', #115879 ) ;
#134250=CARTESIAN_POINT ( 'NONE',  ( 58.42753753994787047, -47.70829528212280479, 34.92499999999998295 ) ) ;
#134252=CARTESIAN_POINT ( 'NONE',  ( 131.8806778009765708, -49.14999999999999147, 40.92499999999998295 ) ) ;
#134294=CARTESIAN_POINT ( 'NONE',  ( 25.39999999999998792, 7.299101704619667785, 2.356075668539098444 ) ) ;
#134345=STYLED_ITEM ( 'NONE', ( #17035 ), #41826 ) ;
#134395=MECHANICAL_DESIGN_GEOMETRIC_PRESENTATION_REPRESENTATION('',(#104343),#129823);
#134409=CARTESIAN_POINT ( 'NONE',  ( -1.537096858564780844, -3.967499999999994476, 6.871911579029513106 ) ) ;
#134419=CYLINDRICAL_SURFACE ( 'NONE', #49597, 3.000000000000002665 ) ;
#134441=FILL_AREA_STYLE_COLOUR ( '', #3906 ) ;
#134540=ORIENTED_EDGE ( 'NONE', *, *, #107714, .T. ) ;
#134543=TOROIDAL_SURFACE ( 'NONE', #81251, 3.000000000000000000, 3.000000000000000000 ) ;
#134551=STYLED_ITEM ( 'NONE', ( #66177 ), #41202 ) ;
#134568=AXIS2_PLACEMENT_3D ( 'NONE', #108485, #64318, #119379 ) ;
#134573=CARTESIAN_POINT ( 'NONE',  ( 131.5423521607622774, -49.05583548141699168, -39.86617647058817226 ) ) ;
#134587=CARTESIAN_POINT ( 'NONE',  ( 6.899972949537105826, 4.461849672132297329, -4.461849672132302658 ) ) ;
#134616=CARTESIAN_POINT ( 'NONE',  ( 21.85373647476855297, -5.808823158059035485, -5.808823158059033709 ) ) ;
#134625=( NAMED_UNIT ( * ) PLANE_ANGLE_UNIT ( ) SI_UNIT ( $, .RADIAN. ) );
#134629=FILL_AREA_STYLE ('',( #26561 ) ) ;
#134650=SURFACE_STYLE_USAGE ( .BOTH. , #133914 ) ;
#134657=DIRECTION ( 'NONE',  ( 0.000000000000000000, -1.000000000000000000, 0.000000000000000000 ) ) ;
#134664=CARTESIAN_POINT ( 'NONE',  ( 12.54166666666666785, 3.047499999999993214, -5.278424836066146320 ) ) ;
#134677=FILL_AREA_STYLE ('',( #46245 ) ) ;
#134684=FACE_OUTER_BOUND ( 'NONE', #82690, .T. ) ;
#134769=DIRECTION ( 'NONE',  ( -0.000000000000000000, 1.000000000000000000, 0.000000000000000000 ) ) ;
#134780=FILL_AREA_STYLE ('',( #46350 ) ) ;
#134797=CARTESIAN_POINT ( 'NONE',  ( 30.83790314143522338, -6.871911579029513106, -3.967499999999993587 ) ) ;
#134823=CARTESIAN_POINT ( 'NONE',  ( 58.77385498567181799, -47.18881911353551573, -35.55177538329067488 ) ) ;
#134827=EDGE_CURVE ( 'NONE', #142647, #4395, #107657, .T. ) ;
#134844=CARTESIAN_POINT ( 'NONE',  ( 16.89540314143521726, 2.126176841940962348, 7.934999999999989839 ) ) ;
#134854=ORIENTED_EDGE ( 'NONE', *, *, #107947, .T. ) ;
#134857=ORIENTED_EDGE ( 'NONE', *, *, #101637, .F. ) ;
#134875=CARTESIAN_POINT ( 'NONE',  ( 152.4000000000000057, 26.55578643762684266, 34.51078643762689069 ) ) ;
#134882=VECTOR ( 'NONE', #20556, 1000.000000000000000 ) ;
#134888=ADVANCED_FACE ( 'NONE', ( #11790 ), #11064, .T. ) ;
#134905=VERTEX_POINT ( 'NONE', #124860 ) ;
#134949=SURFACE_SIDE_STYLE ('',( #13110 ) ) ;
#134966=CARTESIAN_POINT ( 'NONE',  ( 27.19206980810188767, -7.934999999999991616, -2.126176841940955242 ) ) ;
#135012=LINE ( 'NONE', #91487, #58648 ) ;
#135015=DIRECTION ( 'NONE',  ( 0.000000000000000000, 0.000000000000000000, 1.000000000000000000 ) ) ;
#135028=CARTESIAN_POINT ( 'NONE',  ( 1.195149646228581108, -4.118442677489636772, -5.569367250693685101 ) ) ;
#135033=CARTESIAN_POINT ( 'NONE',  ( 25.39999999999998082, 6.833818690505176541, 2.948798542676217327 ) ) ;
#135099=AXIS2_PLACEMENT_3D ( 'NONE', #100912, #90031, #15301 ) ;
#135100=CARTESIAN_POINT ( 'NONE',  ( 28.00000000000002487, -52.14999999999999147, 59.92500000000006111 ) ) ;
#135107=CARTESIAN_POINT ( 'NONE',  ( 22.21247294953710494, 0.000000000000000000, 6.094999999999989981 ) ) ;
#135142=CARTESIAN_POINT ( 'NONE',  ( 1.671236474768553082, 0.000000000000000000, 7.934999999999990727 ) ) ;
#135160=DIRECTION ( 'NONE',  ( 0.000000000000000000, 0.000000000000000000, 1.000000000000000000 ) ) ;
#135165=CARTESIAN_POINT ( 'NONE',  ( 21.77497294953710494, 4.461849672132300881, 4.461849672132299105 ) ) ;
#135170=( NAMED_UNIT ( * ) SI_UNIT ( $, .STERADIAN. ) SOLID_ANGLE_UNIT ( ) );
#135182=CARTESIAN_POINT ( 'NONE',  ( 122.6835989386367345, -1.600000000000094458, 34.92499999999998295 ) ) ;
#135192=ORIENTED_EDGE ( 'NONE', *, *, #11271, .F. ) ;
#135214=DIRECTION ( 'NONE',  ( 0.2400000000000085398, -0.000000000000000000, 0.9707728879609256456 ) ) ;
#135230=FILL_AREA_STYLE ('',( #110561 ) ) ;
#135233=DIRECTION ( 'NONE',  ( -1.000000000000000000, -0.000000000000000000, 0.000000000000000000 ) ) ;
#135250=ORIENTED_EDGE ( 'NONE', *, *, #98117, .T. ) ;
#135255=MECHANICAL_DESIGN_GEOMETRIC_PRESENTATION_REPRESENTATION('',(#91271),#19519);
#135301=B_SPLINE_CURVE_WITH_KNOTS ( 'NONE', 3,
 ( #90731, #32785, #34194, #123362, #80, #68287, #78412, #87852, #79161, #79879, #77011, #21874, #44383, #122609, #13119, #23281 ),
 .UNSPECIFIED., .F., .F.,
 ( 4, 2, 2, 2, 2, 2, 2, 4 ),
 ( 0.000000000000000000, 0.0005244841081218725408, 0.001048968216243745082, 0.002097936432487507077, 0.003146904648731268638, 0.004195872864975030633, 0.006293809297462554624, 0.008391745729950078614 ),
 .UNSPECIFIED. ) ;
#135304=CARTESIAN_POINT ( 'NONE',  ( 8.649972949537106715, -4.461849672132299105, 4.461849672132299993 ) ) ;
#135310=( LENGTH_UNIT ( ) NAMED_UNIT ( * ) SI_UNIT ( .MILLI., .METRE. ) );
#135329=AXIS2_PLACEMENT_3D ( 'NONE', #110997, #78406, #132087 ) ;
#135331=CIRCLE ( 'NONE', #40439, 2.000000000000001776 ) ;
#135332=CARTESIAN_POINT ( 'NONE',  ( 25.49956980810189222, -3.967499999999998028, -6.871911579029511330 ) ) ;
#135340=EDGE_LOOP ( 'NONE', ( #58051, #57783, #141933, #47158 ) ) ;
#135371=STYLED_ITEM ( 'NONE', ( #86068 ), #8773 ) ;
#135373=EDGE_CURVE ( 'NONE', #24682, #100698, #60728, .T. ) ;
#135383=CARTESIAN_POINT ( 'NONE',  ( 12.83333333333333393, 5.278424836066143655, -3.047499999999997655 ) ) ;
#135388=CIRCLE ( 'NONE', #63583, 5.999999999999998224 ) ;
#135395=CARTESIAN_POINT ( 'NONE',  ( 152.4000000000000057, -17.48000000000005016, 12.69999999999954454 ) ) ;
#135423=CARTESIAN_POINT ( 'NONE',  ( 24.39999999999999858, -1.600000000000013634, 20.40202195861969159 ) ) ;
#135434=CARTESIAN_POINT ( 'NONE',  ( 21.35873647476855552, 5.808823158059031044, -5.808823158059037262 ) ) ;
#135436=SURFACE_STYLE_USAGE ( .BOTH. , #13604 ) ;
#135442=( GEOMETRIC_REPRESENTATION_CONTEXT ( 3 ) GLOBAL_UNCERTAINTY_ASSIGNED_CONTEXT ( ( #47503 ) ) GLOBAL_UNIT_ASSIGNED_CONTEXT ( ( #116815, #21614, #45540 ) ) REPRESENTATION_CONTEXT ( 'NONE', 'WORKASPACE' ) );
#135443=CARTESIAN_POINT ( 'NONE',  ( 8.895833333333333925, 1.633150327867687324, -6.094999999999991758 ) ) ;
#135448=COLOUR_RGB ( '', 0.40784314, 0.44705882, 0.49803922) ;
#135481=DIRECTION ( 'NONE',  ( 1.000000000000000000, 0.000000000000000000, -0.000000000000000000 ) ) ;
#135493=CYLINDRICAL_SURFACE ( 'NONE', #7115, 2.552699999999959779 ) ;
#135496=CARTESIAN_POINT ( 'NONE',  ( 25.73373647476855552, 5.808823158059036373, 5.808823158059032821 ) ) ;
#135519=CARTESIAN_POINT ( 'NONE',  ( 61.46640106136302961, -43.14999999999999147, -34.92499999999998295 ) ) ;
#135522=ORIENTED_EDGE ( 'NONE', *, *, #122336, .T. ) ;
#135540=CARTESIAN_POINT ( 'NONE',  ( 24.77040314143521726, -7.934999999999989839, 2.126176841940957907 ) ) ;
#135541=CARTESIAN_POINT ( 'NONE',  ( 2.020403141435219485, 7.934999999999988951, -2.126176841940961904 ) ) ;
#135576=AXIS2_PLACEMENT_3D ( 'NONE', #29799, #30544, #74776 ) ;
#135584=CARTESIAN_POINT ( 'NONE',  ( 25.39999999999999858, -2.600000000000060929, 28.92500000000001492 ) ) ;
#135655=CARTESIAN_POINT ( 'NONE',  ( 25.87956980810188767, 3.967499999999998916, 6.871911579029510442 ) ) ;
#135657=PRESENTATION_STYLE_ASSIGNMENT (( #83423 ) ) ;
#135672=PRESENTATION_STYLE_ASSIGNMENT (( #61009 ) ) ;
#135693=( BOUNDED_CURVE ( )  B_SPLINE_CURVE ( 2, ( #8836, #74903, #53093, #107490, #119768, #20466, #108170, #63320, #42265, #8154, #141565, #86476, #130706 ),
 .UNSPECIFIED., .F., .T. ) 
 B_SPLINE_CURVE_WITH_KNOTS ( ( 3, 2, 2, 2, 2, 2, 3 ),
 ( 0.1000000000000000333, 0.1083333333333333648, 0.1166666666666666963, 0.1250000000000000278, 0.1333333333333333592, 0.1416666666666666907, 0.1500000000000000222 ),
 .UNSPECIFIED. ) 
 CURVE ( )  GEOMETRIC_REPRESENTATION_ITEM ( )  RATIONAL_B_SPLINE_CURVE ( ( 0.9999999999999998890, 0.9659258262890684232, 1.000000000000000000, 0.9659258262890683122, 1.000000000000000000, 0.9659258262890683122, 1.000000000000000000, 0.9659258262890683122, 1.000000000000000000, 0.9659258262890683122, 1.000000000000000000, 0.9659258262890682012, 1.000000000000000222 ) ) 
 REPRESENTATION_ITEM ( '' )  );
#135712=CARTESIAN_POINT ( 'NONE',  ( 0.5689546957196583987, -7.499959106704563006, -0.6961060096647321283 ) ) ;
#135724=CARTESIAN_POINT ( 'NONE',  ( 0.8668240023198436894, 6.544601550655485767, 3.096248083358116965 ) ) ;
#135726=( BOUNDED_CURVE ( )  B_SPLINE_CURVE ( 2, ( #18047, #75348, #52836, #62337, #84779, #107233, #130443, #119510, #41258, #64452, #25763, #113475, #125078 ),
 .UNSPECIFIED., .F., .T. ) 
 B_SPLINE_CURVE_WITH_KNOTS ( ( 3, 2, 2, 2, 2, 2, 3 ),
 ( 0.5000000000000000000, 0.5083333333333333037, 0.5166666666666667185, 0.5250000000000001332, 0.5333333333333334370, 0.5416666666666667407, 0.5500000000000001554 ),
 .UNSPECIFIED. ) 
 CURVE ( )  GEOMETRIC_REPRESENTATION_ITEM ( )  RATIONAL_B_SPLINE_CURVE ( ( 1.000000000000000000, 0.9659258262890683122, 1.000000000000000000, 0.9659258262890683122, 1.000000000000000000, 0.9659258262890683122, 1.000000000000000000, 0.9659258262890683122, 1.000000000000000000, 0.9659258262890683122, 1.000000000000000000, 0.9659258262890678681, 1.000000000000000444 ) ) 
 REPRESENTATION_ITEM ( '' )  );
#135754=DIRECTION ( 'NONE',  ( 0.000000000000000000, 0.000000000000000000, 1.000000000000000000 ) ) ;
#135799=MECHANICAL_DESIGN_GEOMETRIC_PRESENTATION_REPRESENTATION('',(#17696),#38732);
#135811=ORIENTED_EDGE ( 'NONE', *, *, #22966, .F. ) ;
#135824=CARTESIAN_POINT ( 'NONE',  ( -1.391263525231447584, -5.808823158059033709, 5.808823158059035485 ) ) ;
#135859=CARTESIAN_POINT ( 'NONE',  ( 7.270403141435219041, -7.934999999999989839, 2.126176841940957907 ) ) ;
#135874=CARTESIAN_POINT ( 'NONE',  ( 23.96247294953710849, -7.464222240803106570E-16, -6.094999999999989981 ) ) ;
#135882=CARTESIAN_POINT ( 'NONE',  ( 128.5894344200537489, -52.00875322212550600, 39.86617647058822911 ) ) ;
#135926=DIRECTION ( 'NONE',  ( -0.000000000000000000, -1.000000000000000000, 0.000000000000000000 ) ) ;
#135928=B_SPLINE_CURVE_WITH_KNOTS ( 'NONE', 3,
 ( #139853, #28216, #54796, #84727 ),
 .UNSPECIFIED., .F., .F.,
 ( 4, 4 ),
 ( 0.000000000000000000, 0.001824211539880441196 ),
 .UNSPECIFIED. ) ;
#135948=AXIS2_PLACEMENT_3D ( 'NONE', #62330, #106483, #19512 ) ;
#135986=CARTESIAN_POINT ( 'NONE',  ( 8.941639616203772789, -6.094999999999989093, 1.633150327867691765 ) ) ;
#136013=CARTESIAN_POINT ( 'NONE',  ( 19.52040314143522437, 7.934999999999989839, -2.126176841940961904 ) ) ;
#136038=AXIS2_PLACEMENT_3D ( 'NONE', #139772, #137616, #104961 ) ;
#136057=ORIENTED_EDGE ( 'NONE', *, *, #99734, .T. ) ;
#136061=CARTESIAN_POINT ( 'NONE',  ( 23.62500000000000355, 6.094999999999989981, -1.119633336120465690E-15 ) ) ;
#136086=AXIS2_PLACEMENT_3D ( 'NONE', #71104, #38457, #126861 ) ;
#136091=VERTEX_POINT ( 'NONE', #21989 ) ;
#136098=LINE ( 'NONE', #24482, #105599 ) ;
#136113=CARTESIAN_POINT ( 'NONE',  ( 23.10873647476855552, -5.808823158059033709, 5.808823158059035485 ) ) ;
#136183=ORIENTED_EDGE ( 'NONE', *, *, #22966, .T. ) ;
#136186=CARTESIAN_POINT ( 'NONE',  ( 28.65040314143521982, 7.934999999999989839, -2.126176841940961904 ) ) ;
#136207=FACE_OUTER_BOUND ( 'NONE', #23346, .T. ) ;
#136224=( NAMED_UNIT ( * ) SI_UNIT ( $, .STERADIAN. ) SOLID_ANGLE_UNIT ( ) );
#136225=CARTESIAN_POINT ( 'NONE',  ( 31.04123647476855297, 0.000000000000000000, 7.934999999999990727 ) ) ;
#136226=CARTESIAN_POINT ( 'NONE',  ( 0.5620698081018861147, -7.934999999999990727, -2.126176841940955242 ) ) ;
#136251=DIRECTION ( 'NONE',  ( -0.000000000000000000, -0.000000000000000000, -1.000000000000000000 ) ) ;
#136258=SURFACE_SIDE_STYLE ('',( #92034 ) ) ;
#136282=CARTESIAN_POINT ( 'NONE',  ( 0.1600000000000011136, 3.289720434613005118, -7.220939306079887210 ) ) ;
#136311=SURFACE_SIDE_STYLE ('',( #92082 ) ) ;
#136319=ORIENTED_EDGE ( 'NONE', *, *, #28016, .F. ) ;
#136332=ORIENTED_EDGE ( 'NONE', *, *, #43922, .F. ) ;
#136360=CARTESIAN_POINT ( 'NONE',  ( 0.8183591370940799248, -52.14999999999999147, -41.64500000000001023 ) ) ;
#136367=( NAMED_UNIT ( * ) SI_UNIT ( $, .STERADIAN. ) SOLID_ANGLE_UNIT ( ) );
#136370=AXIS2_PLACEMENT_3D ( 'NONE', #51757, #54610, #84394 ) ;
#136385=( LENGTH_UNIT ( ) NAMED_UNIT ( * ) SI_UNIT ( .MILLI., .METRE. ) );
#136394=SURFACE_SIDE_STYLE ('',( #91485 ) ) ;
#136400=ORIENTED_EDGE ( 'NONE', *, *, #105654, .F. ) ;
#136419=CARTESIAN_POINT ( 'NONE',  ( 0.4557000896773421572, 6.785346537228469366, -3.515855491508740105 ) ) ;
#136441=EDGE_LOOP ( 'NONE', ( #60962, #20992, #114136, #46258, #73132, #518, #124845, #98035, #135522, #108824, #75795, #84319, #130940, #81862, #33382, #90477 ) ) ;
#136464=MECHANICAL_DESIGN_GEOMETRIC_PRESENTATION_REPRESENTATION('',(#13711),#67048);
#136484=FILL_AREA_STYLE_COLOUR ( '', #6331 ) ;
#136509=EDGE_LOOP ( 'NONE', ( #128858, #61143, #135192, #52641 ) ) ;
#136517=CARTESIAN_POINT ( 'NONE',  ( 9.692069808101887674, -7.934999999999991616, -2.126176841940955242 ) ) ;
#136550=CARTESIAN_POINT ( 'NONE',  ( 8.874569808101886892, 6.871911579029510442, -3.967499999999998916 ) ) ;
#136557=LINE ( 'NONE', #135182, #25650 ) ;
#136561=CYLINDRICAL_SURFACE ( 'NONE', #96733, 3.000000000000000000 ) ;
#136563=CARTESIAN_POINT ( 'NONE',  ( 183.9346320274809443, -51.67626207039722175, -38.40320453011149482 ) ) ;
#136565=ORIENTED_EDGE ( 'NONE', *, *, #23573, .F. ) ;
#136578=( NAMED_UNIT ( * ) PLANE_ANGLE_UNIT ( ) SI_UNIT ( $, .RADIAN. ) );
#136610=PRESENTATION_STYLE_ASSIGNMENT (( #23766 ) ) ;
#136626=SURFACE_SIDE_STYLE ('',( #72866 ) ) ;
#136663=CARTESIAN_POINT ( 'NONE',  ( 184.1499999999998067, -43.14999999999999147, 34.92499999999998295 ) ) ;
#136677=DIRECTION ( 'NONE',  ( -1.000000000000000000, 0.000000000000000000, 0.000000000000000000 ) ) ;
#136685=( GEOMETRIC_REPRESENTATION_CONTEXT ( 3 ) GLOBAL_UNCERTAINTY_ASSIGNED_CONTEXT ( ( #92356 ) ) GLOBAL_UNIT_ASSIGNED_CONTEXT ( ( #54916, #121569, #10649 ) ) REPRESENTATION_CONTEXT ( 'NONE', 'WORKASPACE' ) );
#136690=CARTESIAN_POINT ( 'NONE',  ( 9.670806282870438864, -3.047499999999997211, -5.278424836066143655 ) ) ;
#136712=FACE_BOUND ( 'NONE', #8644, .T. ) ;
#136720=CARTESIAN_POINT ( 'NONE',  ( 19.22873647476855652, 5.808823158059031044, -5.808823158059038150 ) ) ;
#136727=FILL_AREA_STYLE_COLOUR ( '', #30204 ) ;
#136772=CARTESIAN_POINT ( 'NONE',  ( 22.02083333333333925, -6.094999999999989981, -1.633150327867689100 ) ) ;
#136796=COLOUR_RGB ( '', 0.72549020, 0.75294118, 0.79215686) ;
#136822=CARTESIAN_POINT ( 'NONE',  ( 52.26932219902319332, -49.14999999999999147, -40.92499999999998295 ) ) ;
#136837=CARTESIAN_POINT ( 'NONE',  ( 10.50000000000000000, 0.000000000000000000, 6.094999999999989981 ) ) ;
#136844=CYLINDRICAL_SURFACE ( 'NONE', #76023, 1.000000000000000888 ) ;
#136879=EDGE_CURVE ( 'NONE', #74851, #98477, #27178, .T. ) ;
#136886=( NAMED_UNIT ( * ) SI_UNIT ( $, .STERADIAN. ) SOLID_ANGLE_UNIT ( ) );
#136900=CARTESIAN_POINT ( 'NONE',  ( 152.4000000000000057, 7.919999999999947526, -18.97500000000001918 ) ) ;
#136904=CARTESIAN_POINT ( 'NONE',  ( 27.48373647476854842, -5.808823158059035485, -5.808823158059033709 ) ) ;
#136909=CIRCLE ( 'NONE', #76822, 34.92999999999999972 ) ;
#136922=ORIENTED_EDGE ( 'NONE', *, *, #52176, .T. ) ;
#136928=SURFACE_SIDE_STYLE ('',( #70979 ) ) ;
#136948=CARTESIAN_POINT ( 'NONE',  ( 33.66623647476855297, 7.934999999999990727, -1.457635852685135314E-15 ) ) ;
#136949=CARTESIAN_POINT ( 'NONE',  ( 4.937069808101886004, 2.126176841940952134, -7.934999999999992504 ) ) ;
#136966=AXIS2_PLACEMENT_3D ( 'NONE', #39796, #60111, #128217 ) ;
#137000=EDGE_LOOP ( 'NONE', ( #64299, #56, #34160, #123871 ) ) ;
#137006=VERTEX_POINT ( 'NONE', #143428 ) ;
#137014=VERTEX_POINT ( 'NONE', #42724 ) ;
#137027=( GEOMETRIC_REPRESENTATION_CONTEXT ( 3 ) GLOBAL_UNCERTAINTY_ASSIGNED_CONTEXT ( ( #59413 ) ) GLOBAL_UNIT_ASSIGNED_CONTEXT ( ( #120046, #63603, #31663 ) ) REPRESENTATION_CONTEXT ( 'NONE', 'WORKASPACE' ) );
#137035=EDGE_CURVE ( 'NONE', #5277, #74851, #121665, .T. ) ;
#137051=( NAMED_UNIT ( * ) SI_UNIT ( $, .STERADIAN. ) SOLID_ANGLE_UNIT ( ) );
#137059=( NAMED_UNIT ( * ) SI_UNIT ( $, .STERADIAN. ) SOLID_ANGLE_UNIT ( ) );
#137068=SURFACE_STYLE_USAGE ( .BOTH. , #125485 ) ;
#137081=CARTESIAN_POINT ( 'NONE',  ( 1.087903141435219379, 6.871911579029515771, 3.967499999999989146 ) ) ;
#137091=SURFACE_STYLE_FILL_AREA ( #102343 ) ;
#137105=COLOUR_RGB ( '', 0.72549020, 0.75294118, 0.79215686) ;
#137113=AXIS2_PLACEMENT_3D ( 'NONE', #76255, #54518, #79139 ) ;
#137123=CARTESIAN_POINT ( 'NONE',  ( 25.39999999999999858, 1.194621026894846283, 17.40906030209848510 ) ) ;
#137135=EDGE_LOOP ( 'NONE', ( #36601, #76876, #37071, #58286 ) ) ;
#137151=EDGE_CURVE ( 'NONE', #112625, #96438, #68242, .T. ) ;
#137157=CARTESIAN_POINT ( 'NONE',  ( 181.1500000000000057, -47.62213595499959951, 36.92500000000000426 ) ) ;
#137178=CIRCLE ( 'NONE', #86255, 28.00000000000001776 ) ;
#137180=STYLED_ITEM ( 'NONE', ( #38443 ), #16114 ) ;
#137185=MECHANICAL_DESIGN_GEOMETRIC_PRESENTATION_REPRESENTATION('',(#125603),#23751);
#137258=CARTESIAN_POINT ( 'NONE',  ( 10.71290314143521982, 3.967499999999992699, -6.871911579029513994 ) ) ;
#137295=CARTESIAN_POINT ( 'NONE',  ( 4.207903141435219929, -6.871911579029513106, -3.967499999999993587 ) ) ;
#137308=CARTESIAN_POINT ( 'NONE',  ( 184.1374510928294512, -50.57777258831011125, -35.91905586107257875 ) ) ;
#137323=( LENGTH_UNIT ( ) NAMED_UNIT ( * ) SI_UNIT ( .MILLI., .METRE. ) );
#137353=FILL_AREA_STYLE ('',( #123087 ) ) ;
#137354=( NAMED_UNIT ( * ) PLANE_ANGLE_UNIT ( ) SI_UNIT ( $, .RADIAN. ) );
#137404=VERTEX_POINT ( 'NONE', #135107 ) ;
#137430=CARTESIAN_POINT ( 'NONE',  ( 15.06663961620376924, 1.633150327867695095, 6.094999999999988205 ) ) ;
#137435=ORIENTED_EDGE ( 'NONE', *, *, #126109, .F. ) ;
#137449=CARTESIAN_POINT ( 'NONE',  ( 5.250000000000000000, -7.464222240803106570E-16, -6.094999999999989981 ) ) ;
#137459=CARTESIAN_POINT ( 'NONE',  ( 21.12456980810188867, -6.871911579029512218, 3.967499999999996252 ) ) ;
#137495=FACE_OUTER_BOUND ( 'NONE', #135340, .T. ) ;
#137506=CARTESIAN_POINT ( 'NONE',  ( 25.95833333333333570, -3.047499999999997211, -5.278424836066143655 ) ) ;
#137517=CARTESIAN_POINT ( 'NONE',  ( 166.8575281714868481, 26.96999999999994202, 31.92499999999998295 ) ) ;
#137530=CARTESIAN_POINT ( 'NONE',  ( 13.27083333333333393, 6.094999999999991758, 1.633150327867686880 ) ) ;
#137532=CARTESIAN_POINT ( 'NONE',  ( 2.962472949537105826, -7.464222240803106570E-16, -6.094999999999989981 ) ) ;
#137549=ADVANCED_FACE ( 'NONE', ( #71982, #124903, #48072 ), #105285, .F. ) ;
#137571=DIRECTION ( 'NONE',  ( -1.000000000000000000, -0.000000000000000000, -0.000000000000000000 ) ) ;
#137573=VERTEX_POINT ( 'NONE', #72726 ) ;
#137587=ADVANCED_FACE ( 'NONE', ( #9512 ), #92061, .T. ) ;
#137616=DIRECTION ( 'NONE',  ( -0.000000000000000000, 1.000000000000000000, -0.000000000000000000 ) ) ;
#137636=CARTESIAN_POINT ( 'NONE',  ( 30.40040314143521982, -7.934999999999989839, 2.126176841940957907 ) ) ;
#137671=UNCERTAINTY_MEASURE_WITH_UNIT (LENGTH_MEASURE( 1.000000000000000082E-05 ), #108838, 'distance_accuracy_value', 'NONE');
#137683=CARTESIAN_POINT ( 'NONE',  ( 33.81206980810188156, 7.934999999999993392, 2.126176841940951689 ) ) ;
#137684=CARTESIAN_POINT ( 'NONE',  ( 3.624569808101886448, -6.871911579029512218, 3.967499999999996252 ) ) ;
#137695=SURFACE_STYLE_FILL_AREA ( #93460 ) ;
#137739=CARTESIAN_POINT ( 'NONE',  ( 27.99999999999999645, -57.14999999999999147, -53.92499999999967741 ) ) ;
#137740=CARTESIAN_POINT ( 'NONE',  ( 7.067069808101885897, 2.126176841940952134, -7.934999999999992504 ) ) ;
#137743=STYLED_ITEM ( 'NONE', ( #135672 ), #44864 ) ;
#137744=CARTESIAN_POINT ( 'NONE',  ( 181.1500000000000057, -3.180000000000061444, 31.92499999999998295 ) ) ;
#137756=EDGE_CURVE ( 'NONE', #49688, #89590, #49608, .T. ) ;
#137766=FACE_OUTER_BOUND ( 'NONE', #78925, .T. ) ;
#137808=CARTESIAN_POINT ( 'NONE',  ( 0.5045698081018860082, 6.871911579029510442, -3.967499999999998916 ) ) ;
#137812=( BOUNDED_CURVE ( )  B_SPLINE_CURVE ( 2, ( #49542, #116191, #92275, #73413, #39365, #26335, #127800, #38635, #82866, #95136, #71278, #126346, #127052 ),
 .UNSPECIFIED., .F., .T. ) 
 B_SPLINE_CURVE_WITH_KNOTS ( ( 3, 2, 2, 2, 2, 2, 3 ),
 ( 0.4500000000000000111, 0.4583333333333333148, 0.4666666666666666741, 0.4749999999999999778, 0.4833333333333333370, 0.4916666666666666408, 0.5000000000000000000 ),
 .UNSPECIFIED. ) 
 CURVE ( )  GEOMETRIC_REPRESENTATION_ITEM ( )  RATIONAL_B_SPLINE_CURVE ( ( 1.000000000000000000, 0.9659258262890683122, 1.000000000000000000, 0.9659258262890683122, 1.000000000000000000, 0.9659258262890683122, 1.000000000000000000, 0.9659258262890683122, 1.000000000000000000, 0.9659258262890683122, 1.000000000000000000, 0.9659258262890683122, 1.000000000000000000 ) ) 
 REPRESENTATION_ITEM ( '' )  );
#137819=SURFACE_SIDE_STYLE ('',( #94285 ) ) ;
#137822=CARTESIAN_POINT ( 'NONE',  ( 183.9257687383477560, -48.73293412427588578, -38.67339632249938575 ) ) ;
#137881=DIRECTION ( 'NONE',  ( 0.000000000000000000, 1.000000000000000000, 0.000000000000000000 ) ) ;
#137893=FACE_OUTER_BOUND ( 'NONE', #26589, .T. ) ;
#137934=( NAMED_UNIT ( * ) PLANE_ANGLE_UNIT ( ) SI_UNIT ( $, .RADIAN. ) );
#137935=CARTESIAN_POINT ( 'NONE',  ( 184.1500000000000057, 26.96999999999993847, -34.92499999999998295 ) ) ;
#137958=ORIENTED_EDGE ( 'NONE', *, *, #111888, .T. ) ;
#137974=CARTESIAN_POINT ( 'NONE',  ( 8.671236474768553748, 0.000000000000000000, 7.934999999999990727 ) ) ;
#138004=CARTESIAN_POINT ( 'NONE',  ( 3.916236474768553411, -7.934999999999990727, 4.858786175617117713E-16 ) ) ;
#138018=PRESENTATION_STYLE_ASSIGNMENT (( #6024 ) ) ;
#138024=LINE ( 'NONE', #48882, #41980 ) ;
#138028=CARTESIAN_POINT ( 'NONE',  ( 10.50000000000000000, 0.000000000000000000, 6.094999999999989981 ) ) ;
#138059=LINE ( 'NONE', #5373, #129632 ) ;
#138070=EDGE_LOOP ( 'NONE', ( #116230, #10990, #78051, #12525 ) ) ;
#138115=AXIS2_PLACEMENT_3D ( 'NONE', #82478, #40414, #41102 ) ;
#138118=CARTESIAN_POINT ( 'NONE',  ( 24.39999999999999858, -7.600000000000061817, 28.92499999999998650 ) ) ;
#138126=ORIENTED_EDGE ( 'NONE', *, *, #116709, .T. ) ;
#138127=MECHANICAL_DESIGN_GEOMETRIC_PRESENTATION_REPRESENTATION('',(#8408),#22390);
#138138=CARTESIAN_POINT ( 'NONE',  ( 19.87913961620377279, -5.278424836066145431, -3.047499999999993658 ) ) ;
#138183=CARTESIAN_POINT ( 'NONE',  ( 3.187477005606029756, -48.82538788374344563, -38.96958855984476600 ) ) ;
#138197=AXIS2_PLACEMENT_3D ( 'NONE', #110087, #131146, #97797 ) ;
#138208=DIRECTION ( 'NONE',  ( 1.000000000000000000, 0.000000000000000000, 0.000000000000000000 ) ) ;
#138214=CARTESIAN_POINT ( 'NONE',  ( 25.22916666666666785, -6.094999999999989093, 1.633150327867691765 ) ) ;
#138229=LINE ( 'NONE', #49100, #113383 ) ;
#138247=SURFACE_STYLE_USAGE ( .BOTH. , #94006 ) ;
#138252=EDGE_LOOP ( 'NONE', ( #128208, #33149, #84781, #67398, #84776, #139842, #112414, #88277, #107025, #1154, #48984, #82031, #97867, #134017, #40436, #62731, #112091, #12410 ) ) ;
#138300=CARTESIAN_POINT ( 'NONE',  ( 12.14997294953710849, -4.461849672132299105, 4.461849672132299993 ) ) ;
#138315=( LENGTH_UNIT ( ) NAMED_UNIT ( * ) SI_UNIT ( .MILLI., .METRE. ) );
#138318=FILL_AREA_STYLE_COLOUR ( '', #83072 ) ;
#138324=TOROIDAL_SURFACE ( 'NONE', #136038, 25.00000000000002487, 3.000000000000000000 ) ;
#138331=FILL_AREA_STYLE_COLOUR ( '', #85906 ) ;
#138337=CARTESIAN_POINT ( 'NONE',  ( 1.728736474768552522, 5.808823158059031044, -5.808823158059038150 ) ) ;
#138348=FILL_AREA_STYLE_COLOUR ( '', #77409 ) ;
#138360=CARTESIAN_POINT ( 'NONE',  ( 55.47768537941234257, -49.13871568196521622, -40.16438383193002437 ) ) ;
#138377=CARTESIAN_POINT ( 'NONE',  ( 28.85373647476855652, -5.808823158059035485, -5.808823158059033709 ) ) ;
#138378=CARTESIAN_POINT ( 'NONE',  ( 11.06206980810188689, -7.934999999999990727, -2.126176841940955242 ) ) ;
#138386=EDGE_LOOP ( 'NONE', ( #50877, #18011, #16387, #83853 ) ) ;
#138395=EDGE_CURVE ( 'NONE', #58880, #32751, #83904, .T. ) ;
#138442=CARTESIAN_POINT ( 'NONE',  ( 7.212903141435218934, 3.967499999999992699, -6.871911579029513994 ) ) ;
#138510=( LENGTH_UNIT ( ) NAMED_UNIT ( * ) SI_UNIT ( .MILLI., .METRE. ) );
#138592=VERTEX_POINT ( 'NONE', #59749 ) ;
#138626=B_SPLINE_CURVE_WITH_KNOTS ( 'NONE', 3,
 ( #97670, #78791, #77388, #100541 ),
 .UNSPECIFIED., .F., .F.,
 ( 4, 4 ),
 ( 0.000000000000000000, 0.001115544020566811706 ),
 .UNSPECIFIED. ) ;
#138668=AXIS2_PLACEMENT_3D ( 'NONE', #138933, #138208, #83116 ) ;
#138677=EDGE_LOOP ( 'NONE', ( #86480, #19195, #103708, #45758 ) ) ;
#138680=CARTESIAN_POINT ( 'NONE',  ( 184.1500000000000057, -57.15000000000003411, 15.92499999999935589 ) ) ;
#138690=ORIENTED_EDGE ( 'NONE', *, *, #69978, .T. ) ;
#138694=FACE_OUTER_BOUND ( 'NONE', #107235, .T. ) ;
#138695=CARTESIAN_POINT ( 'NONE',  ( 9.983736474768551972, -5.808823158059035485, -5.808823158059033709 ) ) ;
#138724=CARTESIAN_POINT ( 'NONE',  ( 5.957903141435219929, 6.871911579029515771, 3.967499999999989146 ) ) ;
#138735=CARTESIAN_POINT ( 'NONE',  ( 183.8105469881216436, -51.90335959434332125, -39.28179725402795697 ) ) ;
#138736=ORIENTED_EDGE ( 'NONE', *, *, #80508, .T. ) ;
#138744=CARTESIAN_POINT ( 'NONE',  ( 184.1500000000000057, -30.18000000000009564, 12.69999999999954454 ) ) ;
#138754=UNCERTAINTY_MEASURE_WITH_UNIT (LENGTH_MEASURE( 1.000000000000000082E-05 ), #36118, 'distance_accuracy_value', 'NONE');
#138780=DIRECTION ( 'NONE',  ( 0.000000000000000000, 1.000000000000000000, 0.000000000000000000 ) ) ;
#138824=DIRECTION ( 'NONE',  ( -1.000000000000000000, -0.000000000000000000, -0.000000000000000000 ) ) ;
#138860=CARTESIAN_POINT ( 'NONE',  ( 20.17080628287043709, -3.047499999999997211, -5.278424836066143655 ) ) ;
#138871=CARTESIAN_POINT ( 'NONE',  ( 3.000000000000000000, -43.14999999999999147, 31.92499999999998295 ) ) ;
#138893=ORIENTED_EDGE ( 'NONE', *, *, #129002, .T. ) ;
#138896=CARTESIAN_POINT ( 'NONE',  ( 31.77040314143522082, -7.934999999999989839, 2.126176841940957907 ) ) ;
#138907=CARTESIAN_POINT ( 'NONE',  ( 3.483440076893626003, -49.11775834062216006, -40.20665288735838061 ) ) ;
#138933=CARTESIAN_POINT ( 'NONE',  ( 25.39999999999999858, -43.14999999999999147, -40.92499999999998295 ) ) ;
#138938=CARTESIAN_POINT ( 'NONE',  ( 19.83333333333333570, 5.278424836066143655, -3.047499999999997655 ) ) ;
#138947=FACE_OUTER_BOUND ( 'NONE', #116023, .T. ) ;
#138987=VERTEX_POINT ( 'NONE', #142301 ) ;
#139032=( NAMED_UNIT ( * ) SI_UNIT ( $, .STERADIAN. ) SOLID_ANGLE_UNIT ( ) );
#139052=CARTESIAN_POINT ( 'NONE',  ( 0.07239000078485262335, -48.13855614192807764, 37.56434003615987649 ) ) ;
#139055=CARTESIAN_POINT ( 'NONE',  ( 6.978736474768552966, -5.808823158059033709, 5.808823158059035485 ) ) ;
#139093=UNCERTAINTY_MEASURE_WITH_UNIT (LENGTH_MEASURE( 1.000000000000000082E-05 ), #79225, 'distance_accuracy_value', 'NONE');
#139098=AXIS2_PLACEMENT_3D ( 'NONE', #77936, #35159, #123601 ) ;
#139104=CARTESIAN_POINT ( 'NONE',  ( 27.39540314143522437, 2.126176841940962348, 7.934999999999989839 ) ) ;
#139106=CARTESIAN_POINT ( 'NONE',  ( 6.978736474768552966, -5.808823158059033709, 5.808823158059035485 ) ) ;
#139117=CARTESIAN_POINT ( 'NONE',  ( 23.08747294953710494, -6.094999999999989981, 3.732111120401553285E-16 ) ) ;
#139118=( GEOMETRIC_REPRESENTATION_CONTEXT ( 3 ) GLOBAL_UNCERTAINTY_ASSIGNED_CONTEXT ( ( #17290 ) ) GLOBAL_UNIT_ASSIGNED_CONTEXT ( ( #128184, #6328, #74521 ) ) REPRESENTATION_CONTEXT ( 'NONE', 'WORKASPACE' ) );
#139137=CARTESIAN_POINT ( 'NONE',  ( 56.00844637038723306, -48.60795469097144661, 38.18754904900261238 ) ) ;
#139171=CARTESIAN_POINT ( 'NONE',  ( 6.775403141435219823, -2.126176841940958351, -7.934999999999988951 ) ) ;
#139195=AXIS2_PLACEMENT_3D ( 'NONE', #5860, #113938, #135015 ) ;
#139201=CARTESIAN_POINT ( 'NONE',  ( 25.39999999999999858, -5.131256043349313067, -6.052638797879072108 ) ) ;
#139245=CARTESIAN_POINT ( 'NONE',  ( 12.31706980810188412, -2.126176841940956130, 7.934999999999991616 ) ) ;
#139278=( NAMED_UNIT ( * ) SI_UNIT ( $, .STERADIAN. ) SOLID_ANGLE_UNIT ( ) );
#139282=UNCERTAINTY_MEASURE_WITH_UNIT (LENGTH_MEASURE( 1.000000000000000082E-05 ), #60207, 'distance_accuracy_value', 'NONE');
#139314=PRESENTATION_STYLE_ASSIGNMENT (( #95042 ) ) ;
#139328=DIRECTION ( 'NONE',  ( -1.000000000000000000, -0.000000000000000000, -0.000000000000000000 ) ) ;
#139372=AXIS2_PLACEMENT_3D ( 'NONE', #108861, #35660, #103696 ) ;
#139390=DIRECTION ( 'NONE',  ( -1.000000000000000000, -0.000000000000000000, -0.000000000000000000 ) ) ;
#139400=FILL_AREA_STYLE_COLOUR ( '', #97781 ) ;
#139412=CARTESIAN_POINT ( 'NONE',  ( 20.31663961620377279, -1.633150327867672447, -6.094999999999999751 ) ) ;
#139425=CARTESIAN_POINT ( 'NONE',  ( 4.587903141435219823, 6.871911579029515771, 3.967499999999989146 ) ) ;
#139437=CARTESIAN_POINT ( 'NONE',  ( 10.10830628287044064, 1.633150327867697316, -6.094999999999986429 ) ) ;
#139463=CARTESIAN_POINT ( 'NONE',  ( 11.79123647476855297, -9.717572351234235426E-16, -7.934999999999990727 ) ) ;
#139488=LINE ( 'NONE', #138744, #131951 ) ;
#139494=CARTESIAN_POINT ( 'NONE',  ( 1.886621248228312897, 1.817244688922907692, -5.954744489827652032 ) ) ;
#139509=DIRECTION ( 'NONE',  ( 0.000000000000000000, 1.000000000000000000, 6.938893903907228378E-15 ) ) ;
#139522=CARTESIAN_POINT ( 'NONE',  ( 152.4000000000000057, 25.96999999999993847, -33.92499999999998295 ) ) ;
#139587=ORIENTED_EDGE ( 'NONE', *, *, #133719, .T. ) ;
#139593=CIRCLE ( 'NONE', #9883, 2.999999999999990674 ) ;
#139594=CARTESIAN_POINT ( 'NONE',  ( 12.29580628287044242, -5.278424836066144543, 3.047499999999995879 ) ) ;
#139629=CARTESIAN_POINT ( 'NONE',  ( 33.08290314143522437, 3.967499999999992699, -6.871911579029513994 ) ) ;
#139663=SURFACE_STYLE_USAGE ( .BOTH. , #128060 ) ;
#139664=DIRECTION ( 'NONE',  ( 0.000000000000000000, 0.000000000000000000, -1.000000000000000000 ) ) ;
#139669=( NAMED_UNIT ( * ) SI_UNIT ( $, .STERADIAN. ) SOLID_ANGLE_UNIT ( ) );
#139674=CARTESIAN_POINT ( 'NONE',  ( 34.56250000000000000, 4.461849672132300881, 4.461849672132299105 ) ) ;
#139698=CARTESIAN_POINT ( 'NONE',  ( 1.381925232626255884, -0.1896660010837854515, 6.713074767373758966 ) ) ;
#139736=CARTESIAN_POINT ( 'NONE',  ( 181.1499999999998067, -47.62213595499959951, 36.92500000000000426 ) ) ;
#139772=CARTESIAN_POINT ( 'NONE',  ( 156.1499999999997783, -52.14999999999999147, -34.92499999999975557 ) ) ;
#139780=ADVANCED_FACE ( 'NONE', ( #25139 ), #78844, .F. ) ;
#139790=CARTESIAN_POINT ( 'NONE',  ( 1.582903141435219485, 3.967499999999992699, -6.871911579029513994 ) ) ;
#139837=CARTESIAN_POINT ( 'NONE',  ( 5.979166666666666075, 6.094999999999988205, -1.633150327867694651 ) ) ;
#139838=CARTESIAN_POINT ( 'NONE',  ( 11.93706980810188512, 2.126176841940952134, -7.934999999999992504 ) ) ;
#139839=CIRCLE ( 'NONE', #114348, 28.00000000000002487 ) ;
#139842=ORIENTED_EDGE ( 'NONE', *, *, #9908, .T. ) ;
#139853=CARTESIAN_POINT ( 'NONE',  ( 55.18164086290596515, -52.14999999999999147, -41.64500000000001023 ) ) ;
#139854=SURFACE_SIDE_STYLE ('',( #131813 ) ) ;
#139861=CARTESIAN_POINT ( 'NONE',  ( 56.52198303709688787, -46.44627868284401728, 35.89947574910241457 ) ) ;
#139862=B_SPLINE_CURVE_WITH_KNOTS ( 'NONE', 3,
 ( #116255, #113380, #16946, #14070, #138735, #127870, #136563, #81517, #61220, #137308, #39430, #102547 ),
 .UNSPECIFIED., .F., .F.,
 ( 4, 2, 2, 2, 2, 4 ),
 ( 0.000000000000000000, 0.001816333612422253588, 0.002724500418633388731, 0.003632667224844524090, 0.005449000837266803482, 0.007265334449689082007 ),
 .UNSPECIFIED. ) ;
#139873=TOROIDAL_SURFACE ( 'NONE', #946, 25.00000000000002487, 3.000000000000000000 ) ;
#139888=CARTESIAN_POINT ( 'NONE',  ( 12.90040314143521982, -7.934999999999988951, 2.126176841940957907 ) ) ;
#139921=( GEOMETRIC_REPRESENTATION_CONTEXT ( 3 ) GLOBAL_UNCERTAINTY_ASSIGNED_CONTEXT ( ( #107327 ) ) GLOBAL_UNIT_ASSIGNED_CONTEXT ( ( #65044, #99049, #119375 ) ) REPRESENTATION_CONTEXT ( 'NONE', 'WORKASPACE' ) );
#139940=ORIENTED_EDGE ( 'NONE', *, *, #51179, .F. ) ;
#139956=CARTESIAN_POINT ( 'NONE',  ( 10.56706980810188945, 2.126176841940952134, -7.934999999999993392 ) ) ;
#139971=CARTESIAN_POINT ( 'NONE',  ( 181.1500000013235478, -47.86718710719702585, -37.19897551713905415 ) ) ;
#140029=( NAMED_UNIT ( * ) PLANE_ANGLE_UNIT ( ) SI_UNIT ( $, .RADIAN. ) );
#140040=DIRECTION ( 'NONE',  ( 0.000000000000000000, 1.000000000000000000, 1.286409696682840916E-16 ) ) ;
#140063=VERTEX_POINT ( 'NONE', #95405 ) ;
#140075=( NAMED_UNIT ( * ) SI_UNIT ( $, .STERADIAN. ) SOLID_ANGLE_UNIT ( ) );
#140082=CARTESIAN_POINT ( 'NONE',  ( 3.000000000000000000, -47.62213595499959951, 36.92500000000000426 ) ) ;
#140098=FILL_AREA_STYLE ('',( #139400 ) ) ;
#140121=CARTESIAN_POINT ( 'NONE',  ( 16.83790314143521982, -6.871911579029513106, -3.967499999999993587 ) ) ;
#140152=CARTESIAN_POINT ( 'NONE',  ( 9.749569808101886892, 3.967499999999998916, 6.871911579029510442 ) ) ;
#140160=CARTESIAN_POINT ( 'NONE',  ( 4.712472949537106715, 0.000000000000000000, 6.094999999999989981 ) ) ;
#140164=DIRECTION ( 'NONE',  ( 0.000000000000000000, -1.000000000000000000, 0.000000000000000000 ) ) ;
#140182=AXIS2_PLACEMENT_3D ( 'NONE', #70694, #135233, #59802 ) ;
#140209=LINE ( 'NONE', #117695, #121851 ) ;
#140275=CARTESIAN_POINT ( 'NONE',  ( 18.12913961620377279, 5.278424836066147208, 3.047499999999990550 ) ) ;
#140285=ORIENTED_EDGE ( 'NONE', *, *, #23516, .T. ) ;
#140286=ORIENTED_EDGE ( 'NONE', *, *, #122325, .T. ) ;
#140293=COLOUR_RGB ( '', 0.40784314, 0.44705882, 0.49803922) ;
#140305=CARTESIAN_POINT ( 'NONE',  ( 27.54123647476855652, 0.000000000000000000, 7.934999999999990727 ) ) ;
#140326=ORIENTED_EDGE ( 'NONE', *, *, #13984, .T. ) ;
#140340=SURFACE_STYLE_FILL_AREA ( #94670 ) ;
#140341=UNCERTAINTY_MEASURE_WITH_UNIT (LENGTH_MEASURE( 1.000000000000000082E-05 ), #94244, 'distance_accuracy_value', 'NONE');
#140349=CARTESIAN_POINT ( 'NONE',  ( 31.50000000000000000, 0.000000000000000000, 6.094999999999989981 ) ) ;
#140393=ORIENTED_EDGE ( 'NONE', *, *, #110687, .F. ) ;
#140401=( NAMED_UNIT ( * ) SI_UNIT ( $, .STERADIAN. ) SOLID_ANGLE_UNIT ( ) );
#140427=CARTESIAN_POINT ( 'NONE',  ( 12.29580628287044242, -5.278424836066144543, 3.047499999999995879 ) ) ;
#140459=CARTESIAN_POINT ( 'NONE',  ( 2.999999999999999556, -47.62213595499959951, 36.92500000000000426 ) ) ;
#140461=CARTESIAN_POINT ( 'NONE',  ( 2.749569808101886004, 3.967499999999998916, 6.871911579029510442 ) ) ;
#140483=DIRECTION ( 'NONE',  ( -1.000000000000000000, 0.000000000000000000, 0.000000000000000000 ) ) ;
#140484=CARTESIAN_POINT ( 'NONE',  ( 55.62203754808112421, -51.91654526991841578, -39.52330221398148069 ) ) ;
#140504=CARTESIAN_POINT ( 'NONE',  ( 8.020833333333333925, -6.094999999999989981, -1.633150327867689100 ) ) ;
#140505=CARTESIAN_POINT ( 'NONE',  ( 17.04123647476855652, 0.000000000000000000, 7.934999999999990727 ) ) ;
#140521=( NAMED_UNIT ( * ) SI_UNIT ( $, .STERADIAN. ) SOLID_ANGLE_UNIT ( ) );
#140539=CARTESIAN_POINT ( 'NONE',  ( 128.5279624519181141, -51.91654526992253693, 39.52330221397851062 ) ) ;
#140562=CARTESIAN_POINT ( 'NONE',  ( 5.171236474768553748, 0.000000000000000000, 7.934999999999990727 ) ) ;
#140578=PLANE ( 'NONE',  #141555 ) ;
#140584=CARTESIAN_POINT ( 'NONE',  ( 25.39999999999999858, -1.505985334814471388, -7.801307722062915673 ) ) ;
#140587=VERTEX_POINT ( 'NONE', #720 ) ;
#140612=EDGE_LOOP ( 'NONE', ( #128499, #27184, #113627, #50839 ) ) ;
#140628=CARTESIAN_POINT ( 'NONE',  ( 12.75456980810188767, -6.871911579029512218, 3.967499999999996252 ) ) ;
#140667=CARTESIAN_POINT ( 'NONE',  ( 0.1600000000000021405, -7.631040150288877832, 2.276131627664947921 ) ) ;
#140696=FACE_OUTER_BOUND ( 'NONE', #80040, .T. ) ;
#140700=FILL_AREA_STYLE ('',( #40703 ) ) ;
#140716=EDGE_CURVE ( 'NONE', #8328, #95030, #46479, .T. ) ;
#140717=DIRECTION ( 'NONE',  ( 0.000000000000000000, 1.286409696682840916E-16, -1.000000000000000000 ) ) ;
#140733=CIRCLE ( 'NONE', #136086, 28.00000000000002487 ) ;
#140751=ORIENTED_EDGE ( 'NONE', *, *, #30202, .T. ) ;
#140755=ORIENTED_EDGE ( 'NONE', *, *, #102135, .T. ) ;
#140761=EDGE_CURVE ( 'NONE', #46517, #73841, #64979, .T. ) ;
#140793=CARTESIAN_POINT ( 'NONE',  ( 21.79623647476855552, 7.934999999999990727, -1.457635852685135314E-15 ) ) ;
#140826=CARTESIAN_POINT ( 'NONE',  ( 12.08290314143522082, 3.967499999999992699, -6.871911579029513994 ) ) ;
#140833=CARTESIAN_POINT ( 'NONE',  ( 6.024972949537104938, -4.461849672132299993, -4.461849672132299105 ) ) ;
#140841=SURFACE_STYLE_FILL_AREA ( #96599 ) ;
#140852=CARTESIAN_POINT ( 'NONE',  ( 131.8806778009765708, -49.14999999999999147, 40.92499999999999005 ) ) ;
#140854=CARTESIAN_POINT ( 'NONE',  ( 1.802887254483181323, 1.153283441868768300, -6.189908599751838381 ) ) ;
#140896=CARTESIAN_POINT ( 'NONE',  ( 15.45833333333333393, -3.047499999999997211, -5.278424836066143655 ) ) ;
#140909=SURFACE_STYLE_USAGE ( .BOTH. , #107573 ) ;
#140934=STYLED_ITEM ( 'NONE', ( #76151 ), #49850 ) ;
#140965=CARTESIAN_POINT ( 'NONE',  ( 23.67080628287044064, -3.047499999999997211, -5.278424836066143655 ) ) ;
#140969=ORIENTED_EDGE ( 'NONE', *, *, #43639, .T. ) ;
#141002=CARTESIAN_POINT ( 'NONE',  ( 31.33290314143522082, -3.967499999999994476, 6.871911579029513106 ) ) ;
#141012=STYLED_ITEM ( 'NONE', ( #17454 ), #47140 ) ;
#141033=ORIENTED_EDGE ( 'NONE', *, *, #11053, .F. ) ;
#141036=FACE_OUTER_BOUND ( 'NONE', #60781, .T. ) ;
#141051=CARTESIAN_POINT ( 'NONE',  ( 31.35416666666666785, 1.633150327867695095, 6.094999999999988205 ) ) ;
#141065=CARTESIAN_POINT ( 'NONE',  ( 25.39999999999999858, -7.600000000000055600, -33.92499999999998295 ) ) ;
#141110=CARTESIAN_POINT ( 'NONE',  ( 183.8247562798506749, -48.93522302958620429, 39.28544916627627970 ) ) ;
#141140=SURFACE_SIDE_STYLE ('',( #54882 ) ) ;
#141164=CARTESIAN_POINT ( 'NONE',  ( 0.8183591370940052068, -49.14999999999998437, 41.64499999999997470 ) ) ;
#141168=CARTESIAN_POINT ( 'NONE',  ( 2.166236474768552966, 7.934999999999990727, -1.457635852685135314E-15 ) ) ;
#141214=CARTESIAN_POINT ( 'NONE',  ( 9.187500000000001776, 4.461849672132297329, -4.461849672132302658 ) ) ;
#141215=CARTESIAN_POINT ( 'NONE',  ( 16.31206980810188867, 7.934999999999992504, 2.126176841940951689 ) ) ;
#141220=ORIENTED_EDGE ( 'NONE', *, *, #89778, .F. ) ;
#141230=CARTESIAN_POINT ( 'NONE',  ( 130.7303687233793994, -48.51451318982863370, -38.21513923099880117 ) ) ;
#141239=VERTEX_POINT ( 'NONE', #141065 ) ;
#141242=DIRECTION ( 'NONE',  ( -0.000000000000000000, 1.000000000000000000, -0.000000000000000000 ) ) ;
#141245=CARTESIAN_POINT ( 'NONE',  ( 56.62524208091845423, -47.99115898043764616, 37.22402166429048975 ) ) ;
#141253=CARTESIAN_POINT ( 'NONE',  ( 126.8009042512159539, -49.32595796886460704, 36.54674188582824002 ) ) ;
#141260=EDGE_LOOP ( 'NONE', ( #90899, #45419, #39420, #140755, #94667, #71931, #101398, #15415, #106174, #98289 ) ) ;
#141274=CARTESIAN_POINT ( 'NONE',  ( 17.12956980810188767, -3.967499999999998028, -6.871911579029511330 ) ) ;
#141286=CIRCLE ( 'NONE', #78810, 2.999999999999999556 ) ;
#141306=CARTESIAN_POINT ( 'NONE',  ( 25.40000000000000924, 6.150563586872422661, -5.029781026407817990 ) ) ;
#141318=DIRECTION ( 'NONE',  ( 0.000000000000000000, 0.000000000000000000, 1.000000000000000000 ) ) ;
#141319=SURFACE_SIDE_STYLE ('',( #99968 ) ) ;
#141342=( GEOMETRIC_REPRESENTATION_CONTEXT ( 3 ) GLOBAL_UNCERTAINTY_ASSIGNED_CONTEXT ( ( #2482 ) ) GLOBAL_UNIT_ASSIGNED_CONTEXT ( ( #112838, #134625, #24408 ) ) REPRESENTATION_CONTEXT ( 'NONE', 'WORKASPACE' ) );
#141349=( GEOMETRIC_REPRESENTATION_CONTEXT ( 3 ) GLOBAL_UNCERTAINTY_ASSIGNED_CONTEXT ( ( #56579 ) ) GLOBAL_UNIT_ASSIGNED_CONTEXT ( ( #38703, #4571, #127117 ) ) REPRESENTATION_CONTEXT ( 'NONE', 'WORKASPACE' ) );
#141350=CARTESIAN_POINT ( 'NONE',  ( 10.42123647476855375, -9.717572351234235426E-16, -7.934999999999990727 ) ) ;
#141356=CARTESIAN_POINT ( 'NONE',  ( 55.28643332384059761, -49.19207878845114834, -41.22112633375382984 ) ) ;
#141358=ORIENTED_EDGE ( 'NONE', *, *, #110186, .F. ) ;
#141380=CARTESIAN_POINT ( 'NONE',  ( 0.1164707300447627020, -51.38852430739338217, -37.54101415799215857 ) ) ;
#141381=ORIENTED_EDGE ( 'NONE', *, *, #80668, .T. ) ;
#141393=CARTESIAN_POINT ( 'NONE',  ( 3.500000000000000444, 0.000000000000000000, 6.094999999999989981 ) ) ;
#141420=CARTESIAN_POINT ( 'NONE',  ( 153.4000000000000057, -16.48000000000005016, -34.92499999999998295 ) ) ;
#141443=ADVANCED_FACE ( 'NONE', ( #101131 ), #123007, .T. ) ;
#141536=CARTESIAN_POINT ( 'NONE',  ( 17.42123647476855908, -9.717572351234235426E-16, -7.934999999999990727 ) ) ;
#141555=AXIS2_PLACEMENT_3D ( 'NONE', #44909, #23062, #32562 ) ;
#141565=CARTESIAN_POINT ( 'NONE',  ( 4.958333333333333925, -3.047499999999997211, -5.278424836066143655 ) ) ;
#141575=CARTESIAN_POINT ( 'NONE',  ( 11.35373647476855119, -5.808823158059035485, -5.808823158059033709 ) ) ;
#141643=CARTESIAN_POINT ( 'NONE',  ( 15.02083333333333393, -6.094999999999989981, -1.633150327867689322 ) ) ;
#141649=EDGE_LOOP ( 'NONE', ( #131341, #76409, #108837, #109665 ) ) ;
#141658=DIRECTION ( 'NONE',  ( 0.000000000000000000, 0.000000000000000000, 1.000000000000000000 ) ) ;
#141663=CARTESIAN_POINT ( 'NONE',  ( 3.000000000000000000, -7.600000000000055600, -31.92499999999998650 ) ) ;
#141712=CARTESIAN_POINT ( 'NONE',  ( 29.35830628287044064, -1.633150327867689988, 6.094999999999989981 ) ) ;
#141737=VERTEX_POINT ( 'NONE', #119143 ) ;
#141740=AXIS2_PLACEMENT_3D ( 'NONE', #131440, #143020, #79242 ) ;
#141741=( GEOMETRIC_REPRESENTATION_CONTEXT ( 3 ) GLOBAL_UNCERTAINTY_ASSIGNED_CONTEXT ( ( #133202 ) ) GLOBAL_UNIT_ASSIGNED_CONTEXT ( ( #108989, #108257, #64089 ) ) REPRESENTATION_CONTEXT ( 'NONE', 'WORKASPACE' ) );
#141761=CARTESIAN_POINT ( 'NONE',  ( 55.56056557994607914, -52.00875322212550600, 39.86617647058822911 ) ) ;
#141777=CARTESIAN_POINT ( 'NONE',  ( 128.5894344200537489, -52.00875322212550600, 39.86617647058822911 ) ) ;
#141809=FILL_AREA_STYLE ('',( #97557 ) ) ;
#141824=FILL_AREA_STYLE ('',( #97571 ) ) ;
#141850=EDGE_CURVE ( 'NONE', #138592, #60071, #78515, .T. ) ;
#141854=CARTESIAN_POINT ( 'NONE',  ( 181.1499999999997783, -47.87246431468552998, 37.20487561447688307 ) ) ;
#141863=ORIENTED_EDGE ( 'NONE', *, *, #95752, .T. ) ;
#141868=CARTESIAN_POINT ( 'NONE',  ( 183.7102003651226596, -49.08473565290510265, 39.91868829876759861 ) ) ;
#141928=CARTESIAN_POINT ( 'NONE',  ( 11.35373647476855119, -5.808823158059035485, -5.808823158059033709 ) ) ;
#141933=ORIENTED_EDGE ( 'NONE', *, *, #98117, .F. ) ;
#141939=DIRECTION ( 'NONE',  ( 0.000000000000000000, 0.000000000000000000, -1.000000000000000000 ) ) ;
#141972=CARTESIAN_POINT ( 'NONE',  ( 9.041666666666666075, 3.047499999999993214, -5.278424836066146320 ) ) ;
#141973=CARTESIAN_POINT ( 'NONE',  ( 15.43706980810188512, 2.126176841940952134, -7.934999999999992504 ) ) ;
#141984=CARTESIAN_POINT ( 'NONE',  ( 128.2885478629881959, -48.75494892434343797, -38.51155878621305106 ) ) ;
#141991=( NAMED_UNIT ( * ) PLANE_ANGLE_UNIT ( ) SI_UNIT ( $, .RADIAN. ) );
#142007=CARTESIAN_POINT ( 'NONE',  ( 126.9785101690858085, -47.44491123045132497, 36.62621018406386497 ) ) ;
#142027=STYLED_ITEM ( 'NONE', ( #59973 ), #79080 ) ;
#142046=( NAMED_UNIT ( * ) PLANE_ANGLE_UNIT ( ) SI_UNIT ( $, .RADIAN. ) );
#142097=CARTESIAN_POINT ( 'NONE',  ( 7.650403141435218934, 7.934999999999989839, -2.126176841940961904 ) ) ;
#142101=CARTESIAN_POINT ( 'NONE',  ( 25.39999999999999858, -7.600000000000055600, -28.92499999999998650 ) ) ;
#142126=( GEOMETRIC_REPRESENTATION_CONTEXT ( 3 ) GLOBAL_UNCERTAINTY_ASSIGNED_CONTEXT ( ( #72099 ) ) GLOBAL_UNIT_ASSIGNED_CONTEXT ( ( #18386, #10385, #96653 ) ) REPRESENTATION_CONTEXT ( 'NONE', 'WORKASPACE' ) );
#142165=SURFACE_STYLE_USAGE ( .BOTH. , #30539 ) ;
#142168=CARTESIAN_POINT ( 'NONE',  ( 24.35416666666666785, 1.633150327867675555, 6.094999999999998863 ) ) ;
#142219=CARTESIAN_POINT ( 'NONE',  ( 14.00000000000000178, 0.000000000000000000, 6.094999999999989981 ) ) ;
#142253=EDGE_LOOP ( 'NONE', ( #118614, #102154, #89286, #63201 ) ) ;
#142266=CARTESIAN_POINT ( 'NONE',  ( 18.00456980810188767, 6.871911579029510442, -3.967499999999998916 ) ) ;
#142298=CARTESIAN_POINT ( 'NONE',  ( 184.1500000000000057, -30.18000000000009564, -12.70000000000045404 ) ) ;
#142299=AXIS2_PLACEMENT_3D ( 'NONE', #58145, #48660, #126216 ) ;
#142301=CARTESIAN_POINT ( 'NONE',  ( 156.1499999999997783, -57.14999999999999147, -62.92499999999978400 ) ) ;
#142329=CARTESIAN_POINT ( 'NONE',  ( 0.000000000000000000, -49.14999999999999147, 34.92500000000001847 ) ) ;
#142373=( NAMED_UNIT ( * ) SI_UNIT ( $, .STERADIAN. ) SOLID_ANGLE_UNIT ( ) );
#142421=DIRECTION ( 'NONE',  ( 0.000000000000000000, 0.000000000000000000, 1.000000000000000000 ) ) ;
#142423=ORIENTED_EDGE ( 'NONE', *, *, #28806, .T. ) ;
#142427=ORIENTED_EDGE ( 'NONE', *, *, #107580, .T. ) ;
#142429=EDGE_CURVE ( 'NONE', #85199, #130484, #95037, .T. ) ;
#142431=CARTESIAN_POINT ( 'NONE',  ( 29.64997294953710139, -4.461849672132299105, 4.461849672132299993 ) ) ;
#142448=EDGE_CURVE ( 'NONE', #24260, #119311, #6595, .T. ) ;
#142473=FILL_AREA_STYLE_COLOUR ( '', #135448 ) ;
#142491=( NAMED_UNIT ( * ) SI_UNIT ( $, .STERADIAN. ) SOLID_ANGLE_UNIT ( ) );
#142492=EDGE_CURVE ( 'NONE', #63172, #61426, #7044, .T. ) ;
#142494=DIRECTION ( 'NONE',  ( -1.000000000000000000, -0.000000000000000000, 0.000000000000000000 ) ) ;
#142500=CARTESIAN_POINT ( 'NONE',  ( 53.41205288902393278, -48.51956544822607498, 36.87500513592860329 ) ) ;
#142513=CARTESIAN_POINT ( 'NONE',  ( 32.95833333333334281, -3.047499999999997211, -5.278424836066143655 ) ) ;
#142583=DIRECTION ( 'NONE',  ( 0.000000000000000000, -0.7453559924999275665, 0.6666666666666692942 ) ) ;
#142588=ORIENTED_EDGE ( 'NONE', *, *, #41429, .F. ) ;
#142600=STYLED_ITEM ( 'NONE', ( #49466 ), #39731 ) ;
#142605=CARTESIAN_POINT ( 'NONE',  ( 3.000000000000000000, -4.600000000000013856, 20.40202195861967382 ) ) ;
#142620=CARTESIAN_POINT ( 'NONE',  ( 12.08290314143522082, 3.967499999999992699, -6.871911579029513994 ) ) ;
#142627=CARTESIAN_POINT ( 'NONE',  ( 19.54166666666666785, 3.047499999999993214, -5.278424836066146320 ) ) ;
#142636=ORIENTED_EDGE ( 'NONE', *, *, #23516, .F. ) ;
#142643=DIRECTION ( 'NONE',  ( 0.000000000000000000, 0.000000000000000000, 1.000000000000000000 ) ) ;
#142647=VERTEX_POINT ( 'NONE', #80493 ) ;
#142663=CARTESIAN_POINT ( 'NONE',  ( 1.895833333333333703, 1.633150327867687324, -6.094999999999991758 ) ) ;
#142664=CARTESIAN_POINT ( 'NONE',  ( 14.99956980810188689, -3.967499999999998028, -6.871911579029511330 ) ) ;
#142694=AXIS2_PLACEMENT_3D ( 'NONE', #87076, #132020, #52292 ) ;
#142698=CARTESIAN_POINT ( 'NONE',  ( 123.5545056966327451, -44.02090675802679698, 34.92500000000510596 ) ) ;
#142702=CARTESIAN_POINT ( 'NONE',  ( 184.0335292699551246, -51.38852430739340349, 37.54101415799218699 ) ) ;
#142717=CARTESIAN_POINT ( 'NONE',  ( 18.73373647476854842, 5.808823158059035485, 5.808823158059032821 ) ) ;
#142719=CARTESIAN_POINT ( 'NONE',  ( 161.1238792263967241, 26.96999999999994202, 34.89931327300447350 ) ) ;
#142726=ORIENTED_EDGE ( 'NONE', *, *, #21656, .T. ) ;
#142761=CARTESIAN_POINT ( 'NONE',  ( 0.000000000000000000, -30.18000000000009564, 15.92499999999935945 ) ) ;
#142773=SURFACE_SIDE_STYLE ('',( #51500 ) ) ;
#142785=CARTESIAN_POINT ( 'NONE',  ( 21.94206980810188057, 7.934999999999993392, 2.126176841940951689 ) ) ;
#142817=AXIS2_PLACEMENT_3D ( 'NONE', #126195, #82696, #127627 ) ;
#142826=CARTESIAN_POINT ( 'NONE',  ( 0.1600000000000009748, -7.113645484598424495, 3.515717980648092045 ) ) ;
#142858=CARTESIAN_POINT ( 'NONE',  ( 23.18750000000000355, 4.461849672132297329, -4.461849672132302658 ) ) ;
#142868=EDGE_CURVE ( 'NONE', #80652, #112055, #97763, .T. ) ;
#142883=( GEOMETRIC_REPRESENTATION_CONTEXT ( 3 ) GLOBAL_UNCERTAINTY_ASSIGNED_CONTEXT ( ( #138754 ) ) GLOBAL_UNIT_ASSIGNED_CONTEXT ( ( #36118, #25942, #101348 ) ) REPRESENTATION_CONTEXT ( 'NONE', 'WORKASPACE' ) );
#142887=CARTESIAN_POINT ( 'NONE',  ( 0.000000000000000000, 0.000000000000000000, 0.000000000000000000 ) ) ;
#142917=ORIENTED_EDGE ( 'NONE', *, *, #42385, .F. ) ;
#142922=COLOUR_RGB ( '', 0.09019608, 0.27058824, 0.51372549) ;
#142950=CARTESIAN_POINT ( 'NONE',  ( 20.33790314143522338, -6.871911579029513106, -3.967499999999993587 ) ) ;
#142970=TOROIDAL_SURFACE ( 'NONE', #18244, 6.000000000000000000, 3.000000000000000000 ) ;
#142974=MECHANICAL_DESIGN_GEOMETRIC_PRESENTATION_REPRESENTATION('',(#52724),#75836);
#143003=ORIENTED_EDGE ( 'NONE', *, *, #122261, .F. ) ;
#143020=DIRECTION ( 'NONE',  ( -1.000000000000000000, -0.000000000000000000, -0.000000000000000000 ) ) ;
#143030=MECHANICAL_DESIGN_GEOMETRIC_PRESENTATION_REPRESENTATION('',(#36542),#80542);
#143048=PRESENTATION_STYLE_ASSIGNMENT (( #85095 ) ) ;
#143054=CARTESIAN_POINT ( 'NONE',  ( 15.60416666666666607, -1.633150327867691765, -6.094999999999989093 ) ) ;
#143058=CYLINDRICAL_SURFACE ( 'NONE', #106392, 28.00000000000001776 ) ;
#143070=LINE ( 'NONE', #119854, #134882 ) ;
#143089=VERTEX_POINT ( 'NONE', #135423 ) ;
#143110=VERTEX_POINT ( 'NONE', #106290 ) ;
#143123=CARTESIAN_POINT ( 'NONE',  ( 24.39997294953710139, 4.461849672132297329, -4.461849672132302658 ) ) ;
#143127=EDGE_LOOP ( 'NONE', ( #129665, #142423, #22858, #137958, #12149 ) ) ;
#143179=CARTESIAN_POINT ( 'NONE',  ( 125.7224624600519434, -47.70829528212279769, 34.92499999999998295 ) ) ;
#143185=CIRCLE ( 'NONE', #92248, 4.000000000000000000 ) ;
#143196=CARTESIAN_POINT ( 'NONE',  ( 61.46640106136307935, -43.14999999999999147, 34.92499999999998295 ) ) ;
#143229=AXIS2_PLACEMENT_3D ( 'NONE', #4217, #89861, #46417 ) ;
#143294=( BOUNDED_CURVE ( )  B_SPLINE_CURVE ( 3, ( #66293, #22040, #11138, #132995 ),
 .UNSPECIFIED., .F., .T. ) 
 B_SPLINE_CURVE_WITH_KNOTS ( ( 4, 4 ),
 ( 0.1773996044403779171, 1.570796326794896558 ),
 .UNSPECIFIED. ) 
 CURVE ( )  GEOMETRIC_REPRESENTATION_ITEM ( )  RATIONAL_B_SPLINE_CURVE ( ( 1.000000000000000000, 0.8446433258982485315, 0.8446433258982485315, 1.000000000000000000 ) ) 
 REPRESENTATION_ITEM ( '' )  );
#143309=ORIENTED_EDGE ( 'NONE', *, *, #132256, .F. ) ;
#143320=CARTESIAN_POINT ( 'NONE',  ( 11.06206980810188689, -7.934999999999991616, -2.126176841940955242 ) ) ;
#143348=EDGE_CURVE ( 'NONE', #19621, #91232, #37420, .T. ) ;
#143354=UNCERTAINTY_MEASURE_WITH_UNIT (LENGTH_MEASURE( 1.000000000000000082E-05 ), #87968, 'distance_accuracy_value', 'NONE');
#143364=CARTESIAN_POINT ( 'NONE',  ( 15.45833333333333393, -3.047499999999997211, -5.278424836066143655 ) ) ;
#143365=CARTESIAN_POINT ( 'NONE',  ( 17.91623647476855652, -7.934999999999990727, 4.858786175617117713E-16 ) ) ;
#143381=COLOUR_RGB ( '', 0.40784314, 0.44705882, 0.49803922) ;
#143386=FILL_AREA_STYLE ('',( #6585 ) ) ;
#143396=VERTEX_POINT ( 'NONE', #50364 ) ;
#143398=ORIENTED_EDGE ( 'NONE', *, *, #17130, .F. ) ;
#143421=LINE ( 'NONE', #44128, #124138 ) ;
#143428=CARTESIAN_POINT ( 'NONE',  ( 4.712472949537106715, 0.000000000000000000, 6.094999999999989981 ) ) ;
#143435=DIRECTION ( 'NONE',  ( 0.000000000000000000, 0.000000000000000000, 1.000000000000000000 ) ) ;
#143443=CARTESIAN_POINT ( 'NONE',  ( 24.39999999999999858, -16.48000000000005016, -33.92499999999998295 ) ) ;
#143452=B_SPLINE_CURVE_WITH_KNOTS ( 'NONE', 3,
 ( #14255, #127863, #46945, #18321 ),
 .UNSPECIFIED., .F., .F.,
 ( 4, 4 ),
 ( 0.000000000000000000, 0.001824211539880347737 ),
 .UNSPECIFIED. ) ;
#143460=DIRECTION ( 'NONE',  ( 0.000000000000000000, 0.000000000000000000, -1.000000000000000000 ) ) ;
#143488=CARTESIAN_POINT ( 'NONE',  ( 20.19206980810188767, -7.934999999999991616, -2.126176841940955242 ) ) ;
#143529=DIRECTION ( 'NONE',  ( -1.000000000000000000, -0.000000000000000000, -0.000000000000000000 ) ) ;
#143538=CARTESIAN_POINT ( 'NONE',  ( 22.58290314143522082, 3.967499999999992699, -6.871911579029513994 ) ) ;
#143541=DIRECTION ( 'NONE',  ( -0.000000000000000000, 5.559056632600921604E-15, -1.000000000000000000 ) ) ;
ENDSEC;
END-ISO-10303-21;
